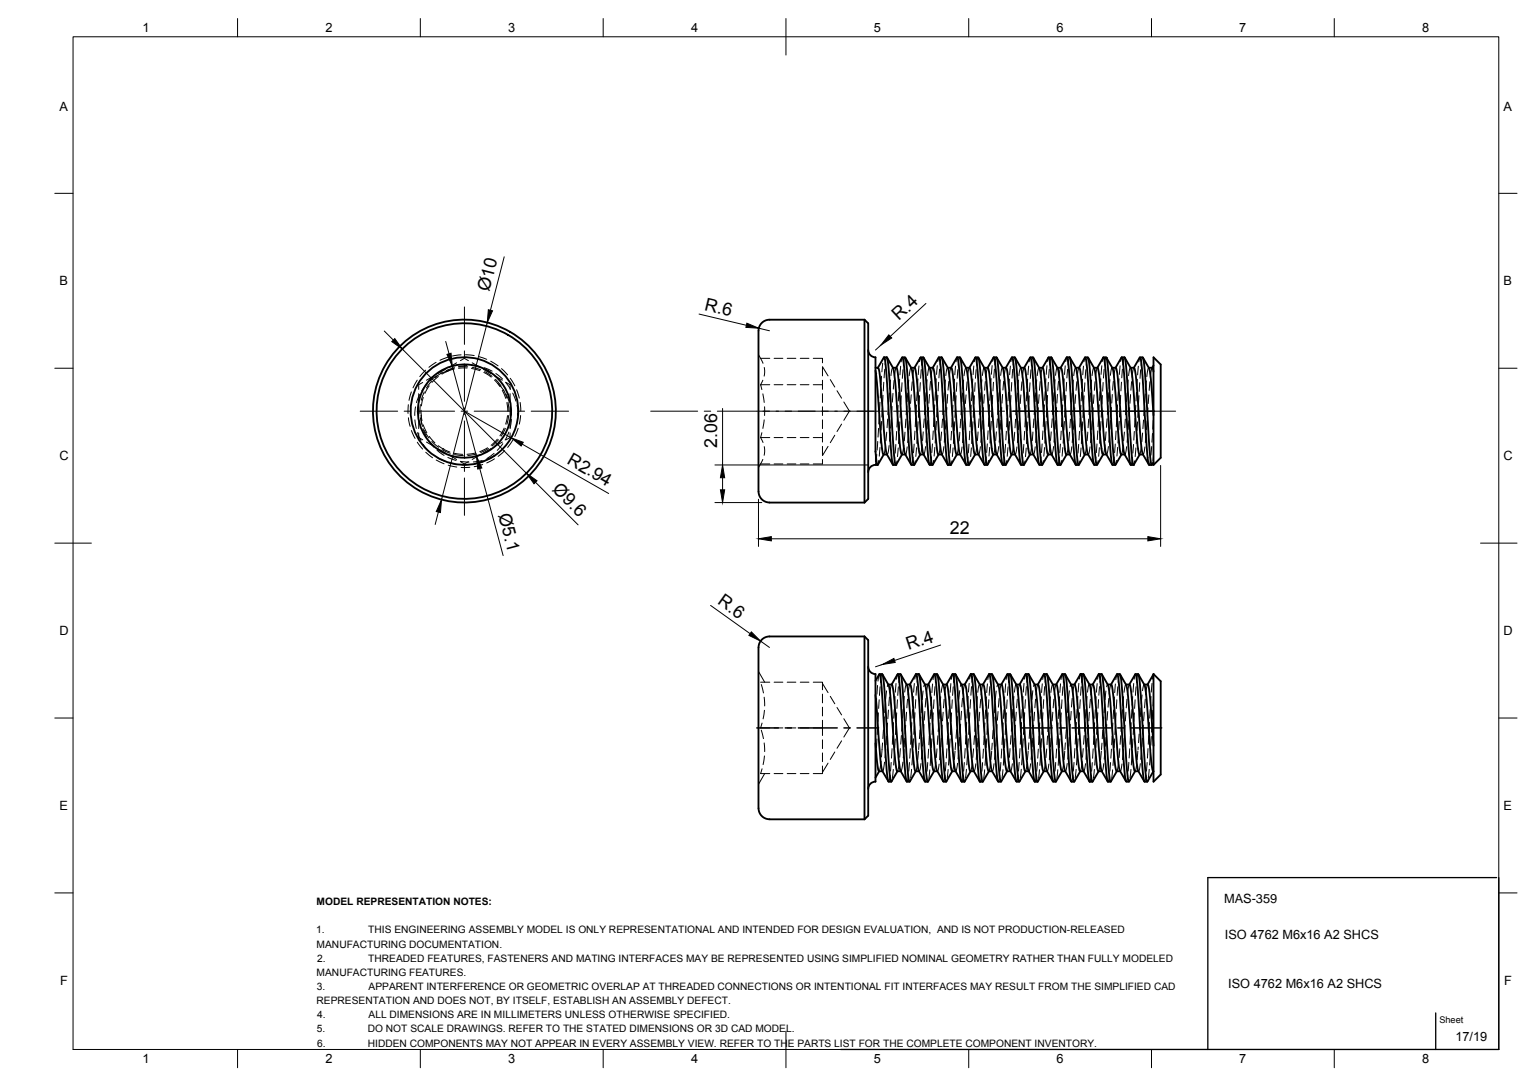
ISO-10303-21;
HEADER;
/* Generated by software containing ST-Developer
 * from STEP Tools, Inc. (www.steptools.com) 
 */

FILE_DESCRIPTION(
/* description */ (''),
/* implementation_level */ '2;1');

FILE_NAME(
/* name */ 'ISO 4762 M6x16 A2 SHCS.step',
/* time_stamp */ '2026-10-15T14:25:16-07:00',
/* author */ (''),
/* organization */ (''),
/* preprocessor_version */ 'ST-DEVELOPER v20.2',
/* originating_system */ 'Autodesk Translation Framework v15.15.0.0',
/* authorisation */ '');

FILE_SCHEMA (('AUTOMOTIVE_DESIGN { 1 0 10303 214 3 1 1 }'));
ENDSEC;

DATA;
#10=MECHANICAL_DESIGN_GEOMETRIC_PRESENTATION_REPRESENTATION('',(#339),#86429);
#159=TOROIDAL_SURFACE('',#17210,0.3342,0.04);
#160=TOROIDAL_SURFACE('',#17226,0.44,0.06);
#258=B_SPLINE_SURFACE_WITH_KNOTS('',3,3,((#85302,#85303,#85304,#85305,#85306,
#85307,#85308,#85309,#85310,#85311,#85312,#85313,#85314,#85315,#85316,#85317,
#85318,#85319,#85320,#85321,#85322,#85323,#85324,#85325,#85326,#85327,#85328,
#85329,#85330,#85331,#85332,#85333,#85334,#85335,#85336,#85337,#85338,#85339,
#85340,#85341,#85342,#85343,#85344,#85345,#85346,#85347,#85348,#85349,#85350,
#85351,#85352,#85353,#85354,#85355,#85356,#85357,#85358,#85359,#85360,#85361,
#85362,#85363,#85364,#85365,#85366,#85367,#85368,#85369,#85370,#85371,#85372,
#85373,#85374,#85375,#85376,#85377,#85378,#85379,#85380,#85381,#85382,#85383,
#85384,#85385,#85386,#85387,#85388,#85389,#85390,#85391,#85392,#85393,#85394,
#85395,#85396,#85397,#85398,#85399,#85400,#85401,#85402),(#85403,#85404,
#85405,#85406,#85407,#85408,#85409,#85410,#85411,#85412,#85413,#85414,#85415,
#85416,#85417,#85418,#85419,#85420,#85421,#85422,#85423,#85424,#85425,#85426,
#85427,#85428,#85429,#85430,#85431,#85432,#85433,#85434,#85435,#85436,#85437,
#85438,#85439,#85440,#85441,#85442,#85443,#85444,#85445,#85446,#85447,#85448,
#85449,#85450,#85451,#85452,#85453,#85454,#85455,#85456,#85457,#85458,#85459,
#85460,#85461,#85462,#85463,#85464,#85465,#85466,#85467,#85468,#85469,#85470,
#85471,#85472,#85473,#85474,#85475,#85476,#85477,#85478,#85479,#85480,#85481,
#85482,#85483,#85484,#85485,#85486,#85487,#85488,#85489,#85490,#85491,#85492,
#85493,#85494,#85495,#85496,#85497,#85498,#85499,#85500,#85501,#85502,#85503),
(#85504,#85505,#85506,#85507,#85508,#85509,#85510,#85511,#85512,#85513,
#85514,#85515,#85516,#85517,#85518,#85519,#85520,#85521,#85522,#85523,#85524,
#85525,#85526,#85527,#85528,#85529,#85530,#85531,#85532,#85533,#85534,#85535,
#85536,#85537,#85538,#85539,#85540,#85541,#85542,#85543,#85544,#85545,#85546,
#85547,#85548,#85549,#85550,#85551,#85552,#85553,#85554,#85555,#85556,#85557,
#85558,#85559,#85560,#85561,#85562,#85563,#85564,#85565,#85566,#85567,#85568,
#85569,#85570,#85571,#85572,#85573,#85574,#85575,#85576,#85577,#85578,#85579,
#85580,#85581,#85582,#85583,#85584,#85585,#85586,#85587,#85588,#85589,#85590,
#85591,#85592,#85593,#85594,#85595,#85596,#85597,#85598,#85599,#85600,#85601,
#85602,#85603,#85604),(#85605,#85606,#85607,#85608,#85609,#85610,#85611,
#85612,#85613,#85614,#85615,#85616,#85617,#85618,#85619,#85620,#85621,#85622,
#85623,#85624,#85625,#85626,#85627,#85628,#85629,#85630,#85631,#85632,#85633,
#85634,#85635,#85636,#85637,#85638,#85639,#85640,#85641,#85642,#85643,#85644,
#85645,#85646,#85647,#85648,#85649,#85650,#85651,#85652,#85653,#85654,#85655,
#85656,#85657,#85658,#85659,#85660,#85661,#85662,#85663,#85664,#85665,#85666,
#85667,#85668,#85669,#85670,#85671,#85672,#85673,#85674,#85675,#85676,#85677,
#85678,#85679,#85680,#85681,#85682,#85683,#85684,#85685,#85686,#85687,#85688,
#85689,#85690,#85691,#85692,#85693,#85694,#85695,#85696,#85697,#85698,#85699,
#85700,#85701,#85702,#85703,#85704,#85705)),.UNSPECIFIED.,.F.,.F.,.F.,(4,
4),(4,1,1,1,1,1,1,1,1,1,1,1,1,1,1,1,1,1,1,1,1,1,1,1,1,1,1,1,1,1,1,1,1,1,
1,1,1,1,1,1,1,1,1,1,1,1,1,1,1,1,1,1,1,1,1,1,1,1,1,1,1,1,1,1,1,1,1,1,1,1,
1,1,1,1,1,1,1,1,1,1,1,1,1,1,1,1,1,1,1,1,1,1,1,1,1,1,1,1,4),(-0.000485376732247951,
0.0662851291984278),(8.30747755240103,9.30363388226323,10.2997902121254,
11.2959465419876,12.2921028718499,13.2882592017121,14.2844155315743,15.2805718614365,
16.2767281912987,17.2728845211609,18.2690408510231,19.2651971808853,20.2613535107475,
21.2575098406097,22.2536661704719,23.2498225003341,24.2459788301963,25.2421351600585,
26.2382914899207,27.234447819783,28.2306041496452,29.2267604795074,30.2229168093696,
31.2190731392318,32.215229469094,33.2113857989562,34.2075421288184,35.2036984586806,
36.1998547885428,37.196011118405,38.1921674482672,39.1883237781294,40.1844801079916,
41.1806364378539,42.1767927677161,43.1729490975783,44.1691054274405,45.1652617573027,
46.1614180871649,47.1575744170271,48.1537307468893,49.1498870767515,50.1460434066137,
51.1421997364759,52.1383560663381,53.1345123962003,54.1306687260625,55.1268250559247,
56.122981385787,57.1191377156492,58.1152940455114,59.1114503753736,60.1076067052358,
61.103763035098,62.0999193649602,63.0960756948224,64.0922320246846,65.0883883545468,
66.084544684409,67.0807010142712,68.0768573441334,69.0730136739956,70.0691700038579,
71.0653263337201,72.0614826635823,73.0576389934445,74.0537953233067,75.0499516531689,
76.0461079830311,77.0422643128933,78.0384206427555,79.0345769726177,80.0307333024799,
81.0268896323421,82.0230459622043,83.0192022920665,84.0153586219288,85.011514951791,
86.0076712816532,87.0038276115154,87.9999839413776,88.9961402712398,89.992296601102,
90.9884529309642,91.9846092608264,92.9807655906886,93.9769219205508,94.973078250413,
95.9692345802752,96.9653909101374,97.9615472399996,98.9577035698618,99.9538598997241,
100.950016229586,101.946172559448,102.942328889311,103.938485219173,104.934641549035,
105.931283255629),.UNSPECIFIED.);
#259=B_SPLINE_SURFACE_WITH_KNOTS('',3,3,((#85831,#85832,#85833,#85834,#85835,
#85836,#85837,#85838,#85839,#85840,#85841,#85842,#85843,#85844,#85845,#85846,
#85847,#85848,#85849,#85850,#85851,#85852,#85853,#85854,#85855,#85856,#85857,
#85858,#85859,#85860,#85861,#85862,#85863,#85864,#85865,#85866,#85867,#85868,
#85869,#85870,#85871,#85872,#85873,#85874,#85875,#85876,#85877,#85878,#85879,
#85880,#85881,#85882,#85883,#85884,#85885,#85886,#85887,#85888,#85889,#85890,
#85891,#85892,#85893,#85894,#85895,#85896,#85897,#85898,#85899,#85900,#85901,
#85902,#85903,#85904,#85905,#85906,#85907,#85908,#85909,#85910,#85911,#85912,
#85913,#85914,#85915,#85916,#85917,#85918,#85919,#85920,#85921,#85922,#85923,
#85924,#85925,#85926,#85927,#85928,#85929,#85930,#85931),(#85932,#85933,
#85934,#85935,#85936,#85937,#85938,#85939,#85940,#85941,#85942,#85943,#85944,
#85945,#85946,#85947,#85948,#85949,#85950,#85951,#85952,#85953,#85954,#85955,
#85956,#85957,#85958,#85959,#85960,#85961,#85962,#85963,#85964,#85965,#85966,
#85967,#85968,#85969,#85970,#85971,#85972,#85973,#85974,#85975,#85976,#85977,
#85978,#85979,#85980,#85981,#85982,#85983,#85984,#85985,#85986,#85987,#85988,
#85989,#85990,#85991,#85992,#85993,#85994,#85995,#85996,#85997,#85998,#85999,
#86000,#86001,#86002,#86003,#86004,#86005,#86006,#86007,#86008,#86009,#86010,
#86011,#86012,#86013,#86014,#86015,#86016,#86017,#86018,#86019,#86020,#86021,
#86022,#86023,#86024,#86025,#86026,#86027,#86028,#86029,#86030,#86031,#86032),
(#86033,#86034,#86035,#86036,#86037,#86038,#86039,#86040,#86041,#86042,
#86043,#86044,#86045,#86046,#86047,#86048,#86049,#86050,#86051,#86052,#86053,
#86054,#86055,#86056,#86057,#86058,#86059,#86060,#86061,#86062,#86063,#86064,
#86065,#86066,#86067,#86068,#86069,#86070,#86071,#86072,#86073,#86074,#86075,
#86076,#86077,#86078,#86079,#86080,#86081,#86082,#86083,#86084,#86085,#86086,
#86087,#86088,#86089,#86090,#86091,#86092,#86093,#86094,#86095,#86096,#86097,
#86098,#86099,#86100,#86101,#86102,#86103,#86104,#86105,#86106,#86107,#86108,
#86109,#86110,#86111,#86112,#86113,#86114,#86115,#86116,#86117,#86118,#86119,
#86120,#86121,#86122,#86123,#86124,#86125,#86126,#86127,#86128,#86129,#86130,
#86131,#86132,#86133),(#86134,#86135,#86136,#86137,#86138,#86139,#86140,
#86141,#86142,#86143,#86144,#86145,#86146,#86147,#86148,#86149,#86150,#86151,
#86152,#86153,#86154,#86155,#86156,#86157,#86158,#86159,#86160,#86161,#86162,
#86163,#86164,#86165,#86166,#86167,#86168,#86169,#86170,#86171,#86172,#86173,
#86174,#86175,#86176,#86177,#86178,#86179,#86180,#86181,#86182,#86183,#86184,
#86185,#86186,#86187,#86188,#86189,#86190,#86191,#86192,#86193,#86194,#86195,
#86196,#86197,#86198,#86199,#86200,#86201,#86202,#86203,#86204,#86205,#86206,
#86207,#86208,#86209,#86210,#86211,#86212,#86213,#86214,#86215,#86216,#86217,
#86218,#86219,#86220,#86221,#86222,#86223,#86224,#86225,#86226,#86227,#86228,
#86229,#86230,#86231,#86232,#86233,#86234)),.UNSPECIFIED.,.F.,.F.,.F.,(4,
4),(4,1,1,1,1,1,1,1,1,1,1,1,1,1,1,1,1,1,1,1,1,1,1,1,1,1,1,1,1,1,1,1,1,1,
1,1,1,1,1,1,1,1,1,1,1,1,1,1,1,1,1,1,1,1,1,1,1,1,1,1,1,1,1,1,1,1,1,1,1,1,
1,1,1,1,1,1,1,1,1,1,1,1,1,1,1,1,1,1,1,1,1,1,1,1,1,1,1,1,4),(-0.000418551673040404,
0.0663322186430087),(11.6145474273763,12.6111891776804,13.6073455075426,
14.6035018374048,15.5996581672671,16.5958144971293,17.5919708269915,18.5881271568537,
19.5842834867159,20.5804398165781,21.5765961464403,22.5727524763025,23.5689088061647,
24.5650651360269,25.5612214658891,26.5573777957513,27.5535341256135,28.5496904554757,
29.545846785338,30.5420031152002,31.5381594450624,32.5343157749246,33.5304721047868,
34.526628434649,35.5227847645112,36.5189410943734,37.5150974242356,38.5112537540978,
39.50741008396,40.5035664138222,41.4997227436844,42.4958790735466,43.4920354034089,
44.4881917332711,45.4843480631333,46.4805043929955,47.4766607228577,48.4728170527199,
49.4689733825821,50.4651297124443,51.4612860423065,52.4574423721687,53.4535987020309,
54.4497550318931,55.4459113617553,56.4420676916176,57.4382240214798,58.434380351342,
59.4305366812042,60.4266930110664,61.4228493409286,62.4190056707908,63.415162000653,
64.4113183305152,65.4074746603774,66.4036309902396,67.3997873201018,68.395943649964,
69.3920999798262,70.3882563096884,71.3844126395506,72.3805689694129,73.3767252992751,
74.3728816291373,75.3690379589995,76.3651942888617,77.3613506187239,78.3575069485861,
79.3536632784483,80.3498196083105,81.3459759381727,82.3421322680349,83.3382885978971,
84.3344449277593,85.3306012576216,86.3267575874838,87.322913917346,88.3190702472082,
89.3152265770704,90.3113829069326,91.3075392367948,92.303695566657,93.2998518965192,
94.2960082263814,95.2921645562436,96.2883208861058,97.284477215968,98.2806335458303,
99.2767898756925,100.272946205555,101.269102535417,102.265258865279,103.261415195141,
104.257571525003,105.253727854866,106.249884184728,107.24604051459,108.242196844452,
109.238353174315),.UNSPECIFIED.);
#280=(
BOUNDED_CURVE()
B_SPLINE_CURVE(2,(#86249,#86250,#86251),.UNSPECIFIED.,.F.,.F.)
B_SPLINE_CURVE_WITH_KNOTS((3,3),(-0.639366558443436,-0.433164349146202),
 .UNSPECIFIED.)
CURVE()
GEOMETRIC_REPRESENTATION_ITEM()
RATIONAL_B_SPLINE_CURVE((1.35866716012837,1.4637604307034,1.4637604307034))
REPRESENTATION_ITEM('')
);
#281=(
BOUNDED_CURVE()
B_SPLINE_CURVE(2,(#86253,#86254,#86255),.UNSPECIFIED.,.F.,.F.)
B_SPLINE_CURVE_WITH_KNOTS((3,3),(0.0319010196424347,0.336489692457453),
 .UNSPECIFIED.)
CURVE()
GEOMETRIC_REPRESENTATION_ITEM()
RATIONAL_B_SPLINE_CURVE((1.03712812921102,1.19757240916823,1.03712812921102))
REPRESENTATION_ITEM('')
);
#282=(
BOUNDED_CURVE()
B_SPLINE_CURVE(2,(#86257,#86258,#86259),.UNSPECIFIED.,.F.,.F.)
B_SPLINE_CURVE_WITH_KNOTS((3,3),(0.0319010196424348,0.336489692457454),
 .UNSPECIFIED.)
CURVE()
GEOMETRIC_REPRESENTATION_ITEM()
RATIONAL_B_SPLINE_CURVE((1.03712812921102,1.19757240916823,1.03712812921102))
REPRESENTATION_ITEM('')
);
#283=(
BOUNDED_CURVE()
B_SPLINE_CURVE(2,(#86261,#86262,#86263),.UNSPECIFIED.,.F.,.F.)
B_SPLINE_CURVE_WITH_KNOTS((3,3),(0.031901019642435,0.336489692457454),
 .UNSPECIFIED.)
CURVE()
GEOMETRIC_REPRESENTATION_ITEM()
RATIONAL_B_SPLINE_CURVE((1.03712812921102,1.19757240916823,1.03712812921102))
REPRESENTATION_ITEM('')
);
#284=(
BOUNDED_CURVE()
B_SPLINE_CURVE(2,(#86265,#86266,#86267),.UNSPECIFIED.,.F.,.F.)
B_SPLINE_CURVE_WITH_KNOTS((3,3),(0.0319010196424349,0.336489692457453),
 .UNSPECIFIED.)
CURVE()
GEOMETRIC_REPRESENTATION_ITEM()
RATIONAL_B_SPLINE_CURVE((1.03712812921102,1.19757240916823,1.03712812921102))
REPRESENTATION_ITEM('')
);
#285=(
BOUNDED_CURVE()
B_SPLINE_CURVE(2,(#86269,#86270,#86271),.UNSPECIFIED.,.F.,.F.)
B_SPLINE_CURVE_WITH_KNOTS((3,3),(0.0319010196424348,0.336489692457453),
 .UNSPECIFIED.)
CURVE()
GEOMETRIC_REPRESENTATION_ITEM()
RATIONAL_B_SPLINE_CURVE((1.03712812921102,1.19757240916823,1.03712812921102))
REPRESENTATION_ITEM('')
);
#286=(
BOUNDED_CURVE()
B_SPLINE_CURVE(2,(#86272,#86273,#86274),.UNSPECIFIED.,.F.,.F.)
B_SPLINE_CURVE_WITH_KNOTS((3,3),(-0.433164349146202,-0.226962139848967),
 .UNSPECIFIED.)
CURVE()
GEOMETRIC_REPRESENTATION_ITEM()
RATIONAL_B_SPLINE_CURVE((1.4637604307034,1.4637604307034,1.35866716012837))
REPRESENTATION_ITEM('')
);
#303=SHAPE_REPRESENTATION_RELATIONSHIP('SRR','None',#86518,#321);
#321=ADVANCED_BREP_SHAPE_REPRESENTATION('',(#357),#86427);
#339=STYLED_ITEM('',(#86617),#357);
#357=MANIFOLD_SOLID_BREP('Body1',#15629);
#1057=B_SPLINE_CURVE_WITH_KNOTS('',3,(#77452,#77453,#77454,#77455,#77456,
#77457,#77458,#77459,#77460,#77461,#77462,#77463,#77464,#77465,#77466,#77467,
#77468,#77469,#77470,#77471,#77472,#77473,#77474,#77475,#77476,#77477,#77478,
#77479,#77480,#77481,#77482,#77483,#77484,#77485,#77486,#77487,#77488,#77489,
#77490,#77491,#77492,#77493,#77494,#77495,#77496,#77497,#77498,#77499,#77500,
#77501,#77502,#77503,#77504,#77505,#77506,#77507,#77508,#77509,#77510,#77511,
#77512,#77513,#77514,#77515,#77516,#77517,#77518,#77519,#77520,#77521,#77522,
#77523,#77524,#77525,#77526,#77527),.UNSPECIFIED.,.F.,.F.,(4,3,3,3,3,3,
3,3,3,3,3,3,3,3,3,3,3,3,3,3,3,3,3,3,3,4),(10.3765279447494,10.5534408108777,
10.7390672436552,10.9156311402548,11.092209959865,11.2691639748381,11.2959465419876,
11.4749627408317,11.6536283105826,11.8322755610944,12.0108999290652,12.1899418681108,
12.2921028718499,12.4705669207875,12.6486653263687,12.8267315154106,13.0047661728317,
13.1832164114546,13.2882592017121,13.4670164932441,13.6454135437631,13.8237819839401,
14.0021213662665,14.1808742422402,14.2844155315743,14.3150784600182),
 .UNSPECIFIED.);
#1058=B_SPLINE_CURVE_WITH_KNOTS('',3,(#77530,#77531,#77532,#77533,#77534,
#77535,#77536,#77537,#77538,#77539,#77540,#77541,#77542,#77543,#77544,#77545,
#77546,#77547,#77548,#77549,#77550,#77551,#77552,#77553,#77554,#77555,#77556,
#77557,#77558,#77559,#77560,#77561,#77562,#77563,#77564,#77565,#77566,#77567,
#77568,#77569,#77570,#77571,#77572,#77573,#77574,#77575,#77576,#77577,#77578),
 .UNSPECIFIED.,.F.,.F.,(4,3,3,3,3,3,3,3,3,3,3,3,3,3,3,3,4),(11.6150328478182,
11.7979860071945,11.9808051200463,12.1638372320247,12.3469748436598,12.5306212400219,
12.6111891776804,12.7880694650036,12.9645487109607,13.1409651633225,13.3173295184066,
13.4941088918777,13.6073455075426,13.7863288313326,13.9649582660013,14.1435821147139,
14.3143563514564),.UNSPECIFIED.);
#1059=B_SPLINE_CURVE_WITH_KNOTS('',3,(#77584,#77585,#77586,#77587,#77588,
#77589,#77590,#77591,#77592,#77593,#77594,#77595,#77596,#77597,#77598,#77599,
#77600,#77601,#77602,#77603,#77604,#77605,#77606,#77607,#77608,#77609,#77610,
#77611,#77612,#77613,#77614,#77615,#77616,#77617,#77618,#77619,#77620,#77621,
#77622,#77623,#77624,#77625,#77626,#77627,#77628,#77629,#77630,#77631,#77632,
#77633,#77634,#77635,#77636,#77637,#77638,#77639,#77640,#77641,#77642,#77643,
#77644,#77645,#77646,#77647,#77648,#77649,#77650,#77651,#77652,#77653,#77654,
#77655,#77656,#77657,#77658,#77659,#77660,#77661,#77662,#77663,#77664,#77665,
#77666,#77667,#77668,#77669,#77670,#77671,#77672,#77673,#77674,#77675,#77676,
#77677,#77678,#77679,#77680,#77681,#77682,#77683,#77684,#77685,#77686,#77687,
#77688,#77689,#77690,#77691,#77692,#77693,#77694,#77695,#77696,#77697,#77698,
#77699,#77700,#77701,#77702,#77703,#77704,#77705,#77706,#77707,#77708,#77709,
#77710,#77711,#77712,#77713,#77714,#77715,#77716,#77717,#77718,#77719,#77720,
#77721,#77722,#77723,#77724,#77725,#77726,#77727,#77728,#77729,#77730,#77731,
#77732,#77733,#77734,#77735,#77736,#77737,#77738,#77739,#77740,#77741),
 .UNSPECIFIED.,.F.,.F.,(4,2,2,2,2,2,2,2,2,2,2,2,2,2,2,2,2,2,2,2,2,2,2,2,
2,2,2,2,2,2,2,2,2,2,2,2,2,2,2,2,2,2,2,2,2,2,2,2,2,2,2,2,2,2,2,2,2,2,2,2,
2,2,2,2,2,2,2,2,2,2,2,2,2,2,2,2,2,2,4),(-1.1637686371979,-1.15330190866645,
-1.1266227046362,-1.09256064921497,-1.08738467839962,-1.08447804691533,
-1.08221855966446,-1.078997200995,-1.0720929569109,-1.04172615958735,-0.985477222491362,
-0.973796375831997,-0.968166209598214,-0.963720443538658,-0.958703261039998,
-0.950091205374077,-0.939562238885692,-0.916459677578588,-0.889953461342887,
-0.855674071252519,-0.850495008033263,-0.847587736517607,-0.845328814306583,
-0.84210950273686,-0.835213509442295,-0.804921450089816,-0.748914527944634,
-0.737014184892147,-0.731344381402372,-0.726895540281821,-0.721904410910814,
-0.713411634220441,-0.664373131981111,-0.621067249054008,-0.614391305574181,
-0.611213164706316,-0.608717662740495,-0.605671704503774,-0.599674578529323,
-0.591733080982927,-0.571582639447149,-0.524620788345343,-0.503713938265148,
-0.496545413852407,-0.491834230609183,-0.48728251741021,-0.480927115237638,
-0.464837122792203,-0.440267116686382,-0.389050830868198,-0.379089415497616,
-0.375263526244851,-0.372703238844456,-0.36999731328955,-0.365610004255846,
-0.349585865669542,-0.315288663196602,-0.272878790086403,-0.263461724321359,
-0.257718225983789,-0.253258721643605,-0.248303879589581,-0.239991273220952,
-0.19806005041918,-0.155468977463997,-0.142952258400057,-0.138787202372248,
-0.136393940808784,-0.133822998673744,-0.13006462663369,-0.119778194296598,
-0.103142576294788,-0.050478661657663,-0.0298185732069449,-0.0226922099751356,
-0.0179928562598389,-0.0137879733802478,-0.00934196527458575,-0.000699766182984735),
 .UNSPECIFIED.);
#1060=B_SPLINE_CURVE_WITH_KNOTS('',3,(#77742,#77743,#77744,#77745,#77746,
#77747,#77748,#77749,#77750,#77751,#77752,#77753,#77754,#77755,#77756,#77757,
#77758,#77759,#77760,#77761,#77762,#77763,#77764,#77765,#77766,#77767,#77768,
#77769),.UNSPECIFIED.,.F.,.F.,(4,3,3,3,3,3,3,3,3,4),(14.3150784600182,14.4937457776235,
14.6720840543341,14.8504232808183,15.0287613104912,15.2075061341743,15.2805718614365,
15.4753006968871,15.6687760212031,15.7079632676679),.UNSPECIFIED.);
#1061=B_SPLINE_CURVE_WITH_KNOTS('',3,(#77771,#77772,#77773,#77774,#77775,
#77776,#77777,#77778,#77779,#77780,#77781,#77782,#77783,#77784,#77785,#77786,
#77787,#77788,#77789,#77790,#77791,#77792,#77793,#77794,#77795,#77796,#77797,
#77798),.UNSPECIFIED.,.F.,.F.,(4,3,3,3,3,3,3,3,3,4),(14.3143563514564,14.4933094485465,
14.6035018374048,14.782517919735,14.9611833677346,15.1398304904322,15.3184547270006,
15.4974965315266,15.5996581672671,15.7079632679489),.UNSPECIFIED.);
#1062=B_SPLINE_CURVE_WITH_KNOTS('',3,(#77799,#77800,#77801,#77802,#77803,
#77804,#77805,#77806,#77807),.UNSPECIFIED.,.F.,.F.,(4,1,1,1,1,1,4),(15.7079719561269,
16.5958144971293,17.5919708269915,18.5881271568537,19.5842834867159,20.5804398165781,
20.5982114559267),.UNSPECIFIED.);
#1063=B_SPLINE_CURVE_WITH_KNOTS('',3,(#77812,#77813,#77814,#77815,#77816,
#77817,#77818,#77819,#77820,#77821,#77822,#77823,#77824,#77825,#77826,#77827,
#77828,#77829,#77830,#77831,#77832,#77833,#77834,#77835,#77836,#77837,#77838,
#77839,#77840,#77841,#77842,#77843,#77844,#77845,#77846,#77847,#77848,#77849,
#77850,#77851,#77852,#77853,#77854,#77855,#77856,#77857,#77858,#77859,#77860,
#77861,#77862,#77863,#77864,#77865,#77866,#77867,#77868,#77869,#77870,#77871,
#77872,#77873,#77874,#77875,#77876,#77877,#77878,#77879,#77880,#77881,#77882,
#77883,#77884,#77885,#77886,#77887,#77888,#77889,#77890,#77891,#77892,#77893,
#77894,#77895,#77896,#77897,#77898,#77899,#77900,#77901,#77902,#77903,#77904,
#77905,#77906,#77907,#77908,#77909,#77910,#77911,#77912,#77913,#77914,#77915,
#77916,#77917,#77918,#77919,#77920,#77921,#77922,#77923,#77924,#77925,#77926,
#77927,#77928,#77929,#77930,#77931,#77932,#77933,#77934,#77935,#77936,#77937,
#77938,#77939,#77940,#77941,#77942,#77943,#77944,#77945,#77946,#77947,#77948,
#77949,#77950,#77951,#77952,#77953,#77954,#77955,#77956,#77957,#77958,#77959,
#77960,#77961,#77962,#77963,#77964,#77965,#77966,#77967,#77968,#77969,#77970,
#77971,#77972,#77973,#77974,#77975,#77976,#77977,#77978,#77979,#77980,#77981,
#77982,#77983,#77984,#77985,#77986,#77987,#77988,#77989,#77990,#77991,#77992,
#77993,#77994,#77995,#77996,#77997,#77998,#77999,#78000,#78001,#78002,#78003,
#78004,#78005,#78006,#78007,#78008,#78009,#78010,#78011),.UNSPECIFIED.,
 .F.,.F.,(4,2,2,2,2,2,2,2,2,2,2,2,2,2,2,2,2,2,2,2,2,2,2,2,2,2,2,2,2,2,2,
2,2,2,2,2,2,2,2,2,2,2,2,2,2,2,2,2,2,2,2,2,2,2,2,2,2,2,2,2,2,2,2,2,2,2,2,
2,2,2,2,2,2,2,2,2,2,2,2,2,2,2,2,2,2,2,2,2,2,2,2,2,2,2,2,2,2,2,2,4),(-2.65808856585573,
-2.63896562788725,-2.63024927627796,-2.62521051743156,-2.62076872278231,
-2.61517461241825,-2.6062689530765,-2.5513950124766,-2.51544918010836,-2.50936210629664,
-2.50629807350984,-2.50380303304675,-2.50064471262094,-2.49407411644601,
-2.44976929489784,-2.40203764363037,-2.39331977274927,-2.38828057986316,
-2.38383866330352,-2.37824474799765,-2.36934011948885,-2.31445077379584,
-2.27851439127394,-2.27242733281257,-2.26936323959744,-2.2668681185348,
-2.26370965614897,-2.25713861298752,-2.2017312222126,-2.17077686377812,
-2.15859407969893,-2.15287242873246,-2.14841731415237,-2.14345454859754,
-2.13509748541681,-2.0951234442445,-2.05593101002078,-2.0387950323599,-2.03431776630312,
-2.03159340734376,-2.02904621173316,-2.02588911944168,-2.01787577779181,
-1.96444395966839,-1.93959584089493,-1.92857108602373,-1.91964494170661,
-1.91456171004154,-1.91012494278449,-1.90459542172365,-1.89381350566269,
-1.83664403989336,-1.80598134791393,-1.79904746452727,-1.79582076722484,
-1.79356077273059,-1.79065792279702,-1.78549903676126,-1.75436601730428,
-1.74873945594128,-1.72440702662619,-1.70150725376204,-1.68616841063085,
-1.67992413442162,-1.67539174120084,-1.67121220600676,-1.66437677015089,
-1.64621779537558,-1.59677293989029,-1.57591590069346,-1.56395836850383,
-1.55998444930628,-1.55736887806426,-1.55469837777831,-1.55046830899439,
-1.53739869282542,-1.4952686832497,-1.45374841823445,-1.44537309055035,
-1.44040618715214,-1.43595146846488,-1.43023605973783,-1.41808965995798,
-1.38854667801837,-1.37144368022104,-1.3320774905639,-1.32522592009405,
-1.32201448470216,-1.31951701519194,-1.31649796412889,-1.31063541532598,
-1.27331494399624,-1.21970325024029,-1.2106828051401,-1.20505488719733,
-1.20060947887647,-1.19559121578042,-1.18697354308848,-1.1764356290778,
-1.1637686371979),.UNSPECIFIED.);
#1064=B_SPLINE_CURVE_WITH_KNOTS('',3,(#78013,#78014,#78015,#78016,#78017),
 .UNSPECIFIED.,.F.,.F.,(4,1,4),(20.5982114559267,21.5765961464403,21.9911426690459),
 .UNSPECIFIED.);
#1065=B_SPLINE_CURVE_WITH_KNOTS('',3,(#78018,#78019,#78020,#78021,#78022,
#78023,#78024,#78025,#78026,#78027,#78028,#78029,#78030,#78031,#78032,#78033,
#78034,#78035,#78036,#78037,#78038,#78039,#78040,#78041,#78042,#78043,#78044,
#78045,#78046,#78047,#78048,#78049,#78050,#78051,#78052,#78053,#78054,#78055,
#78056,#78057,#78058,#78059,#78060,#78061,#78062,#78063,#78064,#78065,#78066,
#78067,#78068,#78069,#78070,#78071,#78072,#78073,#78074,#78075,#78076,#78077,
#78078,#78079,#78080,#78081,#78082,#78083,#78084,#78085,#78086,#78087,#78088,
#78089,#78090,#78091,#78092,#78093,#78094,#78095,#78096,#78097,#78098,#78099,
#78100,#78101,#78102,#78103,#78104,#78105,#78106,#78107,#78108,#78109,#78110,
#78111,#78112,#78113,#78114,#78115,#78116,#78117,#78118,#78119,#78120,#78121,
#78122,#78123,#78124,#78125,#78126,#78127,#78128,#78129,#78130,#78131,#78132,
#78133,#78134,#78135,#78136,#78137,#78138,#78139,#78140,#78141,#78142,#78143,
#78144,#78145,#78146,#78147,#78148,#78149,#78150,#78151,#78152,#78153,#78154,
#78155,#78156,#78157,#78158,#78159,#78160,#78161,#78162,#78163,#78164,#78165,
#78166,#78167,#78168,#78169,#78170,#78171,#78172,#78173,#78174,#78175,#78176,
#78177,#78178,#78179),.UNSPECIFIED.,.F.,.F.,(4,2,2,2,2,2,2,2,2,2,2,2,2,
2,2,2,2,2,2,2,2,2,2,2,2,2,2,2,2,2,2,2,2,2,2,2,2,2,2,2,2,2,2,2,2,2,2,2,2,
2,2,2,2,2,2,2,2,2,2,2,2,2,2,2,2,2,2,2,2,2,2,2,2,2,2,2,2,2,2,2,4),(-2.98904427612266,
-2.98271778473439,-2.97723402516263,-2.972808221092,-2.96859102543041,-2.9638636072836,
-2.95660538824093,-2.9347749884518,-2.8780081973523,-2.86484611471672,-2.85611824490066,
-2.85258738524914,-2.85005559451206,-2.84723593943615,-2.84231751051577,
-2.82084252248546,-2.77782499244362,-2.75666538903467,-2.74214902509585,
-2.73603421462947,-2.73152544592232,-2.72731801991099,-2.72032021305432,
-2.70093465123872,-2.65264122893888,-2.63211123115884,-2.62407775210138,
-2.61802862591414,-2.61497288896346,-2.61247871788276,-2.60931409623699,
-2.60270569116392,-2.55889221680947,-2.51069964266647,-2.50201121946722,
-2.49697984405979,-2.49253943310642,-2.48694023389954,-2.47541478443228,
-2.4189661619931,-2.38852972679637,-2.38162043088732,-2.3783993783485,-2.37614113267091,
-2.37323753987195,-2.36807078495652,-2.33461177733176,-2.30788095203421,
-2.28444726017468,-2.27382408444184,-2.26515242446383,-2.260124416451,-2.25568323515178,
-2.25007803662293,-2.23852146689319,-2.18210551792869,-2.15167878190711,
-2.14477021088004,-2.1415491492634,-2.13929074525505,-2.13638671022134,
-2.13121871603868,-2.0976648901883,-2.07107968066547,-2.04761151404457,
-2.03697807939041,-2.02829972680073,-2.02326999295449,-2.01882855559658,
-2.01322473389622,-2.00428263892065,-1.94016200242408,-1.92088338084325,
-1.91316033955907,-1.90729069036377,-1.90427084749759,-1.90177442137465,
-1.89856660520185,-1.89173066883819,-1.85200521610118,-1.82619474000714),
 .UNSPECIFIED.);
#1066=B_SPLINE_CURVE_WITH_KNOTS('',3,(#78185,#78186,#78187,#78188,#78189,
#78190,#78191,#78192,#78193,#78194,#78195,#78196,#78197,#78198,#78199,#78200,
#78201,#78202,#78203,#78204,#78205,#78206,#78207,#78208,#78209,#78210,#78211,
#78212,#78213,#78214,#78215,#78216,#78217,#78218,#78219,#78220,#78221,#78222,
#78223,#78224,#78225,#78226,#78227,#78228,#78229,#78230,#78231,#78232,#78233,
#78234,#78235,#78236,#78237,#78238,#78239,#78240,#78241,#78242,#78243,#78244,
#78245,#78246,#78247,#78248,#78249,#78250,#78251,#78252,#78253,#78254,#78255,
#78256,#78257,#78258,#78259,#78260,#78261,#78262,#78263,#78264,#78265,#78266,
#78267,#78268,#78269,#78270,#78271,#78272,#78273,#78274,#78275,#78276,#78277,
#78278,#78279,#78280,#78281,#78282,#78283,#78284,#78285,#78286,#78287,#78288,
#78289,#78290,#78291,#78292,#78293,#78294,#78295,#78296,#78297,#78298,#78299,
#78300,#78301,#78302,#78303,#78304,#78305,#78306,#78307,#78308,#78309,#78310,
#78311,#78312,#78313,#78314,#78315,#78316,#78317,#78318,#78319,#78320,#78321,
#78322,#78323,#78324,#78325,#78326,#78327,#78328,#78329,#78330,#78331,#78332,
#78333,#78334),.UNSPECIFIED.,.F.,.F.,(4,2,2,2,2,2,2,2,2,2,2,2,2,2,2,2,2,
2,2,2,2,2,2,2,2,2,2,2,2,2,2,2,2,2,2,2,2,2,2,2,2,2,2,2,2,2,2,2,2,2,2,2,2,
2,2,2,2,2,2,2,2,2,2,2,2,2,2,2,2,2,2,2,2,2,4),(-1.16370274550239,-1.1568070636298,
-1.13677589009422,-1.09022559976082,-1.06886026428964,-1.06164448485992,
-1.05692378948761,-1.0523786955524,-1.04605868477085,-1.03020861191811,
-1.00617866458583,-0.960418696062841,-0.945412959897615,-0.940975534683176,
-0.938259967017763,-0.935677531247388,-0.931866614661771,-0.921205588553841,
-0.903674646488405,-0.850676930739111,-0.831467699059262,-0.824489994217004,
-0.820285042041834,-0.81577164368852,-0.809637560886505,-0.795009473094288,
-0.773617630303817,-0.730663875046565,-0.709419145398833,-0.704509960324899,
-0.701691479497393,-0.69915723216955,-0.695618378437064,-0.686847962239203,
-0.673600358750618,-0.640301644144528,-0.597358254095201,-0.589007533560267,
-0.584046121250254,-0.579590717172288,-0.573866598030166,-0.561670356831813,
-0.530349090617642,-0.475447713250732,-0.468765208229255,-0.465585489510032,
-0.463089540991608,-0.460043956096899,-0.454049880629331,-0.419293719725962,
-0.362790523781181,-0.354060467579551,-0.348517507309125,-0.344079690939804,
-0.339005837902028,-0.330124410646265,-0.319169620966451,-0.29457213689166,
-0.24317543339214,-0.233373696231229,-0.229572198251925,-0.227088455460331,
-0.224467495629112,-0.220543910049425,-0.215691303369064,-0.185311480080651,
-0.129024907015343,-0.117373078218063,-0.111748538710975,-0.107303611633095,
-0.102283579199003,-0.093656951979499,-0.045572454012865,-0.0264879389893685,
-0.000696886015620926),.UNSPECIFIED.);
#1067=B_SPLINE_CURVE_WITH_KNOTS('',3,(#78335,#78336,#78337,#78338,#78339,
#78340,#78341,#78342,#78343,#78344,#78345,#78346,#78347,#78348,#78349,#78350,
#78351,#78352,#78353,#78354,#78355,#78356,#78357,#78358,#78359,#78360,#78361,
#78362,#78363,#78364,#78365,#78366,#78367,#78368,#78369,#78370,#78371,#78372,
#78373,#78374,#78375,#78376,#78377,#78378,#78379,#78380,#78381,#78382,#78383,
#78384),.UNSPECIFIED.,.F.,.F.,(4,2,2,2,2,2,2,2,2,2,2,2,2,2,2,2,2,2,2,2,
2,2,2,2,4),(-2.98929417603817,-2.98366351093371,-2.98108078519344,-2.97872868114393,
-2.97602838999981,-2.97166071400982,-2.95731736208476,-2.90550643056215,
-2.88469583141012,-2.87034731868861,-2.86425776659884,-2.85975166729322,
-2.85553532914993,-2.84849538068428,-2.82877056877828,-2.78076354833954,
-2.76031364017731,-2.7522987727458,-2.74625987964001,-2.74320552365715,
-2.74071023304375,-2.73754130231533,-2.73091460922501,-2.68712217695227,
-2.65808856585573),.UNSPECIFIED.);
#1068=B_SPLINE_CURVE_WITH_KNOTS('',3,(#78385,#78386,#78387,#78388,#78389,
#78390,#78391,#78392,#78393,#78394,#78395,#78396,#78397,#78398,#78399,#78400,
#78401,#78402,#78403,#78404,#78405,#78406,#78407,#78408,#78409,#78410,#78411,
#78412,#78413,#78414,#78415,#78416,#78417,#78418,#78419,#78420,#78421,#78422,
#78423,#78424,#78425,#78426,#78427,#78428,#78429,#78430,#78431,#78432,#78433,
#78434,#78435,#78436,#78437,#78438,#78439,#78440,#78441,#78442,#78443,#78444,
#78445,#78446,#78447,#78448,#78449,#78450,#78451,#78452,#78453,#78454,#78455,
#78456,#78457,#78458,#78459,#78460,#78461,#78462,#78463,#78464,#78465,#78466,
#78467,#78468,#78469,#78470,#78471,#78472,#78473,#78474,#78475,#78476,#78477,
#78478,#78479,#78480,#78481,#78482,#78483,#78484,#78485,#78486,#78487,#78488,
#78489,#78490,#78491,#78492,#78493,#78494,#78495,#78496,#78497,#78498,#78499,
#78500,#78501,#78502,#78503,#78504,#78505,#78506,#78507,#78508,#78509,#78510,
#78511,#78512,#78513,#78514,#78515,#78516,#78517,#78518,#78519,#78520,#78521,
#78522,#78523,#78524,#78525,#78526,#78527,#78528,#78529,#78530,#78531,#78532,
#78533,#78534,#78535,#78536,#78537,#78538,#78539,#78540,#78541,#78542,#78543,
#78544,#78545,#78546,#78547,#78548,#78549,#78550,#78551,#78552,#78553,#78554,
#78555,#78556,#78557,#78558,#78559,#78560,#78561,#78562,#78563,#78564,#78565,
#78566,#78567,#78568,#78569,#78570,#78571,#78572,#78573,#78574,#78575,#78576,
#78577,#78578,#78579,#78580,#78581,#78582,#78583,#78584,#78585,#78586,#78587,
#78588,#78589,#78590),.UNSPECIFIED.,.F.,.F.,(4,2,2,2,2,2,2,2,2,2,2,2,2,
2,2,2,2,2,2,2,2,2,2,2,2,2,2,2,2,2,2,2,2,2,2,2,2,2,2,2,2,2,2,2,2,2,2,2,2,
2,2,2,2,2,2,2,2,2,2,2,2,2,2,2,2,2,2,2,2,2,2,2,2,2,2,2,2,2,2,2,2,2,2,2,2,
2,2,2,2,2,2,2,2,2,2,2,2,2,2,2,2,2,4),(-1.82619474000714,-1.81669741450079,
-1.79650086386287,-1.789613921023,-1.78496136321705,-1.78042251728144,-1.77491811234969,
-1.76127711035731,-1.74625882417755,-1.68188711327217,-1.67211761041369,
-1.66842967734056,-1.66587063032776,-1.66311420019153,-1.65848885920151,
-1.64151002192613,-1.60225772689917,-1.56897584375519,-1.55672051941941,
-1.55098639324071,-1.54653051962872,-1.54157609445583,-1.53325563140524,
-1.49466335660825,-1.45743394032513,-1.437550799349,-1.43271462594213,-1.42991222682865,
-1.42737282286278,-1.42379962009082,-1.41480533885329,-1.40108138580043,
-1.34043394780875,-1.32244194173736,-1.31563144561288,-1.31145732217809,
-1.30692316509088,-1.30066249446532,-1.28520789385302,-1.26205154942839,
-1.2352577680559,-1.20133550613098,-1.19616217617814,-1.19325661030326,
-1.19099786028261,-1.18777748573651,-1.18087490185015,-1.15051586874477,
-1.09430007401147,-1.08258277692584,-1.07694694805024,-1.07250191359706,
-1.06749108174361,-1.0589041346484,-1.04841376525451,-1.02544119200211,
-1.00018973591792,-0.96714389852926,-0.960900215830101,-0.957762813917686,
-0.955221096582854,-0.952489029087609,-0.947974317147941,-0.930342404916655,
-0.888683926910013,-0.851675930912225,-0.843385475754152,-0.838437776911538,
-0.833981018607295,-0.828236015619667,-0.815918204719248,-0.780911992980148,
-0.738774158470005,-0.725680028827143,-0.721447940407098,-0.718777634633902,
-0.716163722646667,-0.712194629329707,-0.700269438407626,-0.679498921374576,
-0.630347434893704,-0.611914528525312,-0.605042390726706,-0.600857341912173,
-0.596331960689134,-0.590121185929433,-0.574993877641159,-0.552545240818545,
-0.525568261588957,-0.490706261849459,-0.485516419066132,-0.482607273277968,
-0.480349276223882,-0.477134579256861,-0.470261993623915,-0.440196236852249,
-0.384897242937592,-0.372356597316411,-0.366634047993919,-0.362168080016405,
-0.357259060357152,-0.349149922815078,-0.331944024529),.UNSPECIFIED.);
#1069=B_SPLINE_CURVE_WITH_KNOTS('',3,(#78595,#78596,#78597,#78598,#78599,
#78600,#78601,#78602,#78603,#78604,#78605,#78606,#78607,#78608,#78609,#78610,
#78611,#78612,#78613,#78614,#78615,#78616,#78617,#78618,#78619,#78620,#78621,
#78622,#78623,#78624,#78625,#78626,#78627,#78628,#78629,#78630,#78631,#78632,
#78633,#78634,#78635,#78636,#78637,#78638,#78639,#78640,#78641,#78642,#78643,
#78644,#78645,#78646,#78647,#78648,#78649,#78650,#78651,#78652,#78653,#78654,
#78655,#78656,#78657,#78658,#78659,#78660,#78661,#78662,#78663,#78664,#78665,
#78666,#78667,#78668,#78669,#78670,#78671,#78672,#78673,#78674,#78675,#78676,
#78677,#78678,#78679,#78680,#78681,#78682,#78683,#78684,#78685,#78686,#78687,
#78688,#78689,#78690,#78691,#78692,#78693,#78694,#78695,#78696,#78697,#78698,
#78699,#78700,#78701,#78702,#78703,#78704,#78705,#78706,#78707,#78708,#78709,
#78710,#78711,#78712,#78713,#78714,#78715,#78716,#78717,#78718,#78719,#78720,
#78721,#78722,#78723,#78724,#78725,#78726,#78727,#78728,#78729,#78730,#78731,
#78732,#78733,#78734,#78735,#78736,#78737,#78738,#78739,#78740,#78741,#78742,
#78743,#78744,#78745,#78746,#78747,#78748,#78749,#78750,#78751,#78752,#78753,
#78754,#78755,#78756,#78757,#78758,#78759,#78760,#78761,#78762,#78763,#78764,
#78765,#78766,#78767,#78768,#78769,#78770,#78771,#78772,#78773,#78774,#78775,
#78776,#78777,#78778,#78779,#78780,#78781,#78782,#78783,#78784,#78785,#78786,
#78787,#78788,#78789,#78790,#78791,#78792),.UNSPECIFIED.,.F.,.F.,(4,2,2,
2,2,2,2,2,2,2,2,2,2,2,2,2,2,2,2,2,2,2,2,2,2,2,2,2,2,2,2,2,2,2,2,2,2,2,2,
2,2,2,2,2,2,2,2,2,2,2,2,2,2,2,2,2,2,2,2,2,2,2,2,2,2,2,2,2,2,2,2,2,2,2,2,
2,2,2,2,2,2,2,2,2,2,2,2,2,2,2,2,2,2,2,2,2,2,2,4),(-2.65779610798801,-2.64562846272747,
-2.60539466897641,-2.59993510794725,-2.59699977757073,-2.59449419130625,
-2.59122688046561,-2.58387137384898,-2.52947682521431,-2.5045178668195,
-2.49346363101895,-2.48451958776003,-2.47943357363947,-2.47499861327236,
-2.46947687916789,-2.45836581710353,-2.40144586488319,-2.37086433866569,
-2.36393979188862,-2.3607154206473,-2.3584562875984,-2.35555347922215,-2.35039226412067,
-2.31812074255177,-2.31274400261798,-2.2892518720084,-2.26640335760273,
-2.25594928612956,-2.24738482600682,-2.24237868461594,-2.23793270748448,
-2.23228870337808,-2.22321002925658,-2.17029679400594,-2.13275401676145,
-2.12665282896889,-2.12358626746513,-2.12109169838593,-2.11793716643286,
-2.1113848807021,-2.06676972492304,-2.01930673296878,-2.01060593952897,
-2.00557084313888,-2.00112913862138,-1.99553093590684,-1.98661005050956,
-1.93190836177424,-1.89505724763879,-1.88944323507208,-1.88647547099182,
-1.88397380115751,-1.88075105932935,-1.87364845895274,-1.82617224122379,
-1.78178492927898,-1.77341929044655,-1.76845513984121,-1.76400104671987,
-1.75828386923519,-1.74895229982513,-1.70113421315615,-1.65903167114846,
-1.65288311093852,-1.64980701890483,-1.64731252070541,-1.6441679185956,
-1.63766814368582,-1.59197443816894,-1.57816910688654,-1.5555758876386,
-1.54037970337555,-1.53415780035787,-1.52962986346544,-1.5248794105215,
-1.51752078509346,-1.49484243099641,-1.45484019718156,-1.42066591456986,
-1.41548888453754,-1.41258223510258,-1.41032322344123,-1.40710314550051,
-1.4002036909885,-1.36987820446382,-1.31375981100097,-1.30196519050354,
-1.29631459278727,-1.29186747410937,-1.28686429341757,-1.27831569524545,
-1.22924081769557,-1.18611808435823,-1.17941967489536,-1.17623716529217,
-1.17374136543791,-1.17069882392811,-1.16471888888895,-1.16370274550239),
 .UNSPECIFIED.);
#1070=B_SPLINE_CURVE_WITH_KNOTS('',3,(#78794,#78795,#78796,#78797,#78798,
#78799,#78800,#78801,#78802,#78803,#78804,#78805,#78806,#78807,#78808,#78809,
#78810,#78811,#78812,#78813,#78814,#78815,#78816,#78817,#78818,#78819,#78820,
#78821,#78822,#78823,#78824,#78825,#78826,#78827,#78828,#78829,#78830,#78831,
#78832,#78833,#78834,#78835,#78836,#78837,#78838,#78839,#78840,#78841,#78842,
#78843),.UNSPECIFIED.,.F.,.F.,(4,2,2,2,2,2,2,2,2,2,2,2,2,2,2,2,2,2,2,2,
2,2,2,2,4),(-0.331944024529,-0.312841878134531,-0.295797672941764,-0.256356303392932,
-0.249523574006143,-0.246316348325045,-0.24381997457475,-0.240799682720564,
-0.234927739803417,-0.195081674214772,-0.144398316709289,-0.135177121109271,
-0.129492211160779,-0.125042428831186,-0.12006158181438,-0.111614647314127,
-0.10134315480156,-0.0791140033701062,-0.0287009707118166,-0.0151068306855188,
-0.0108193652246315,-0.00813703130472152,-0.00579380909874595,-0.00316163883082362,
-0.000696074731363536),.UNSPECIFIED.);
#1071=B_SPLINE_CURVE_WITH_KNOTS('',3,(#78844,#78845,#78846,#78847,#78848,
#78849,#78850,#78851,#78852,#78853,#78854,#78855,#78856,#78857,#78858,#78859,
#78860,#78861,#78862,#78863,#78864,#78865,#78866,#78867,#78868,#78869,#78870,
#78871,#78872,#78873,#78874,#78875,#78876,#78877,#78878,#78879,#78880,#78881,
#78882,#78883,#78884,#78885,#78886,#78887,#78888,#78889,#78890,#78891,#78892,
#78893,#78894,#78895,#78896,#78897,#78898,#78899,#78900,#78901,#78902,#78903,
#78904,#78905,#78906,#78907,#78908,#78909,#78910,#78911,#78912,#78913,#78914,
#78915,#78916,#78917,#78918,#78919,#78920,#78921,#78922,#78923,#78924,#78925,
#78926,#78927,#78928,#78929,#78930,#78931,#78932,#78933,#78934,#78935,#78936,
#78937,#78938,#78939,#78940,#78941,#78942,#78943,#78944,#78945,#78946,#78947,
#78948,#78949,#78950,#78951,#78952,#78953,#78954,#78955,#78956,#78957,#78958,
#78959,#78960,#78961,#78962,#78963,#78964,#78965,#78966,#78967,#78968,#78969,
#78970,#78971,#78972,#78973,#78974,#78975,#78976,#78977,#78978,#78979,#78980,
#78981,#78982,#78983,#78984,#78985,#78986,#78987,#78988,#78989,#78990,#78991,
#78992,#78993,#78994,#78995,#78996,#78997,#78998,#78999,#79000,#79001,#79002,
#79003,#79004,#79005,#79006,#79007,#79008,#79009,#79010,#79011,#79012,#79013,
#79014,#79015,#79016,#79017,#79018,#79019,#79020,#79021,#79022,#79023,#79024,
#79025,#79026,#79027,#79028,#79029,#79030,#79031,#79032,#79033,#79034,#79035,
#79036,#79037,#79038,#79039),.UNSPECIFIED.,.F.,.F.,(4,2,2,2,2,2,2,2,2,2,
2,2,2,2,2,2,2,2,2,2,2,2,2,2,2,2,2,2,2,2,2,2,2,2,2,2,2,2,2,2,2,2,2,2,2,2,
2,2,2,2,2,2,2,2,2,2,2,2,2,2,2,2,2,2,2,2,2,2,2,2,2,2,2,2,2,2,2,2,2,2,2,2,
2,2,2,2,2,2,2,2,2,2,2,2,2,2,2,4),(-2.98986290590906,-2.9811645609045,-2.93860454829328,
-2.89411772806824,-2.88536790530145,-2.8803230618328,-2.87588370936346,
-2.87030313328637,-2.86144069728388,-2.79693950862918,-2.77781347126643,
-2.77012912135672,-2.76594868825332,-2.76245881001136,-2.76241330075756,
-2.76236793090525,-2.7623226514419,-2.76227741250219,-2.76223216313041,
-2.76218685102507,-2.7621414222526,-2.76209582093373,-2.7620499889014,-2.76200386531906,
-2.76195738624712,-2.7619104841631,-2.76186308740373,-2.76181511954432,
-2.76176649867618,-2.76171713657784,-2.76166693774644,-2.76161579827013,
-2.76156360450819,-2.76151023152379,-2.76145554121485,-2.76139938008659,
-2.76134157654138,-2.76130713089662,-2.7588952078203,-2.75575019173004,
-2.74924639835194,-2.70397057987953,-2.65698912986836,-2.64833458917462,
-2.64330966533014,-2.63886715545892,-2.63325481985386,-2.62166306138798,
-2.56527676212363,-2.53485753660154,-2.52794910234861,-2.52472774225655,
-2.52246900472342,-2.51956438114988,-2.51439489299499,-2.48075844393766,
-2.45428442783653,-2.43079032625652,-2.42014887725035,-2.41146516604408,
-2.40643384957864,-2.40199191514795,-2.3963886777886,-2.38484700688701,
-2.32839887375958,-2.29795931995531,-2.29104856636941,-2.28782664159736,
-2.2855677078503,-2.28266311284791,-2.2774942984965,-2.24396712553781,-2.21694798800437,
-2.18885651097065,-2.17675251197165,-2.17104566766734,-2.1665928882549,
-2.16162330150009,-2.1532316396023,-2.10914264085504,-2.07326352521092,
-2.05686094880649,-2.05244370148903,-2.04973277551116,-2.0471784146474,
-2.04337912651513,-2.03358852798327,-1.98220305753126,-1.95761568076255,
-1.94151656959651,-1.93516060948433,-1.93060946631103,-1.92589974097122,
-1.91873524137024,-1.89786176046146,-1.85083914353397,-1.83066715315173,
-1.82676239401596),.UNSPECIFIED.);
#1072=B_SPLINE_CURVE_WITH_KNOTS('',3,(#79045,#79046,#79047,#79048,#79049,
#79050,#79051,#79052,#79053,#79054,#79055,#79056,#79057,#79058,#79059,#79060,
#79061,#79062,#79063,#79064,#79065,#79066,#79067,#79068,#79069,#79070,#79071,
#79072,#79073,#79074,#79075,#79076,#79077,#79078,#79079,#79080,#79081,#79082,
#79083,#79084,#79085,#79086,#79087,#79088,#79089,#79090,#79091,#79092,#79093,
#79094,#79095,#79096,#79097,#79098,#79099,#79100,#79101,#79102,#79103,#79104,
#79105,#79106,#79107,#79108,#79109,#79110,#79111,#79112,#79113,#79114,#79115,
#79116,#79117,#79118,#79119,#79120,#79121,#79122,#79123,#79124,#79125,#79126,
#79127,#79128,#79129,#79130,#79131,#79132,#79133,#79134,#79135,#79136,#79137,
#79138,#79139,#79140,#79141,#79142,#79143,#79144,#79145,#79146,#79147,#79148,
#79149,#79150,#79151,#79152,#79153,#79154,#79155,#79156,#79157,#79158,#79159,
#79160,#79161,#79162,#79163,#79164,#79165,#79166,#79167,#79168,#79169,#79170,
#79171,#79172,#79173,#79174,#79175,#79176,#79177,#79178,#79179,#79180,#79181,
#79182,#79183,#79184,#79185,#79186,#79187,#79188,#79189,#79190,#79191,#79192,
#79193,#79194,#79195,#79196,#79197,#79198,#79199,#79200),.UNSPECIFIED.,
 .F.,.F.,(4,2,2,2,2,2,2,2,2,2,2,2,2,2,2,2,2,2,2,2,2,2,2,2,2,2,2,2,2,2,2,
2,2,2,2,2,2,2,2,2,2,2,2,2,2,2,2,2,2,2,2,2,2,2,2,2,2,2,2,2,2,2,2,2,2,2,2,
2,2,2,2,2,2,2,2,2,2,4),(-1.16379924314915,-1.15636896341719,-1.15072066708933,
-1.14627242167782,-1.14126489131265,-1.13270105731949,-1.122248306252,-1.09940987025486,
-1.07662727515485,-1.04094595192493,-1.0339798750836,-1.03074690518291,
-1.02824774255948,-1.02524482100174,-1.01946304593492,-1.01189225967026,
-0.993214480620849,-0.930428876149755,-0.919137758977803,-0.91358027292429,
-0.909140699661688,-0.904075522018791,-0.89523755988362,-0.848586864867644,
-0.803271713780177,-0.796745700141823,-0.79359547923121,-0.791100113886125,
-0.788027371158756,-0.781898592007223,-0.741786031843394,-0.691828023119278,
-0.68256938397034,-0.676872150100689,-0.672419035246775,-0.667440953377183,
-0.659014738978724,-0.610846558273101,-0.566350925816522,-0.559786690543437,
-0.556629115506364,-0.554133508653195,-0.551067343783175,-0.544971869070915,
-0.508097090812731,-0.45439106830036,-0.445377150286841,-0.43975067632214,
-0.43530481552055,-0.430284357372875,-0.421658607396983,-0.411108472381106,
-0.387934685436907,-0.361082605444902,-0.327237667455879,-0.32206376080669,
-0.319157366076106,-0.31689761785202,-0.31367527182871,-0.306766223562171,
-0.276355430680164,-0.220041575978518,-0.208419630605263,-0.202800111613543,
-0.198355065547207,-0.193585482945275,-0.185515120101929,-0.175629661124755,
-0.15468558629736,-0.126343850363146,-0.0930276647544607,-0.0861036582085444,
-0.0828786447279151,-0.0803802108174482,-0.0773715980702051,-0.0715610444402044,
-0.0639408967511788,-0.000697042157991375),.UNSPECIFIED.);
#1073=B_SPLINE_CURVE_WITH_KNOTS('',3,(#79201,#79202,#79203,#79204,#79205,
#79206,#79207,#79208,#79209,#79210,#79211,#79212,#79213,#79214,#79215,#79216,
#79217,#79218,#79219,#79220,#79221,#79222,#79223,#79224,#79225,#79226,#79227,
#79228,#79229,#79230,#79231,#79232,#79233,#79234,#79235,#79236,#79237,#79238,
#79239,#79240,#79241,#79242,#79243,#79244,#79245,#79246,#79247,#79248),
 .UNSPECIFIED.,.F.,.F.,(4,2,2,2,2,2,2,2,2,2,2,2,2,2,2,2,2,2,2,2,2,2,2,4),
(-2.98915910611891,-2.97245947833514,-2.96192457934277,-2.95701634474704,
-2.95285674097329,-2.94840886300484,-2.94274081448435,-2.93357753277321,
-2.90038509321121,-2.85100678772585,-2.84310478890941,-2.83713139739069,
-2.83409067085517,-2.83159548951468,-2.82841268419511,-2.82170994269704,
-2.77869299185966,-2.72942034717541,-2.72097004287315,-2.71598853099697,
-2.71153890583765,-2.70585519559141,-2.69663786776816,-2.65779610798801),
 .UNSPECIFIED.);
#1074=B_SPLINE_CURVE_WITH_KNOTS('',3,(#79249,#79250,#79251,#79252,#79253,
#79254,#79255,#79256,#79257,#79258,#79259,#79260,#79261,#79262,#79263,#79264,
#79265,#79266,#79267,#79268,#79269,#79270,#79271,#79272,#79273,#79274,#79275,
#79276,#79277,#79278,#79279,#79280,#79281,#79282,#79283,#79284,#79285,#79286,
#79287,#79288,#79289,#79290,#79291,#79292,#79293,#79294,#79295,#79296,#79297,
#79298,#79299,#79300,#79301,#79302,#79303,#79304,#79305,#79306,#79307,#79308,
#79309,#79310,#79311,#79312,#79313,#79314,#79315,#79316,#79317,#79318,#79319,
#79320,#79321,#79322,#79323,#79324,#79325,#79326,#79327,#79328,#79329,#79330,
#79331,#79332,#79333,#79334,#79335,#79336,#79337,#79338,#79339,#79340,#79341,
#79342,#79343,#79344,#79345,#79346,#79347,#79348,#79349,#79350,#79351,#79352,
#79353,#79354,#79355,#79356,#79357,#79358,#79359,#79360,#79361,#79362,#79363,
#79364,#79365,#79366,#79367,#79368,#79369,#79370,#79371,#79372,#79373,#79374,
#79375,#79376,#79377,#79378,#79379,#79380,#79381,#79382,#79383,#79384,#79385,
#79386,#79387,#79388,#79389,#79390,#79391,#79392,#79393,#79394,#79395,#79396,
#79397,#79398,#79399,#79400,#79401,#79402,#79403,#79404,#79405,#79406,#79407,
#79408,#79409,#79410,#79411,#79412,#79413,#79414,#79415,#79416,#79417,#79418,
#79419,#79420,#79421,#79422,#79423,#79424,#79425,#79426,#79427,#79428,#79429,
#79430,#79431,#79432,#79433,#79434,#79435,#79436,#79437,#79438,#79439,#79440,
#79441,#79442,#79443,#79444,#79445,#79446),.UNSPECIFIED.,.F.,.F.,(4,2,2,
2,2,2,2,2,2,2,2,2,2,2,2,2,2,2,2,2,2,2,2,2,2,2,2,2,2,2,2,2,2,2,2,2,2,2,2,
2,2,2,2,2,2,2,2,2,2,2,2,2,2,2,2,2,2,2,2,2,2,2,2,2,2,2,2,2,2,2,2,2,2,2,2,
2,2,2,2,2,2,2,2,2,2,2,2,2,2,2,2,2,2,2,2,2,2,2,4),(-1.82676239401596,-1.82272046736094,
-1.81672091864089,-1.81367460450555,-1.81117924027603,-1.80800188504408,
-1.8013298649085,-1.7580267840685,-1.70924301533283,-1.70062747953582,-1.69561033741196,
-1.69116586736496,-1.68553910548193,-1.67652046621759,-1.61274221472753,
-1.59331247162085,-1.58189494164362,-1.57798706850257,-1.57538545123259,
-1.57269840983678,-1.56839104192817,-1.55463061891724,-1.4955156127764,
-1.47041984850611,-1.46275451371483,-1.45793950490291,-1.45344188485792,
-1.44740446573964,-1.43337791652622,-1.413220985141,-1.38407955151575,-1.38005003406147,
-1.34749079807617,-1.34232668583597,-1.33942307286952,-1.33716382487661,
-1.33394011285789,-1.32702015150965,-1.29649124919368,-1.23973617586962,
-1.22848682257969,-1.22293841141856,-1.21850097949893,-1.21343274810444,
-1.20457502187683,-1.15733511690643,-1.11269733616998,-1.10614179980468,
-1.10298658428462,-1.10049195548535,-1.09742599605467,-1.09132813154709,
-1.05408312357184,-1.00082882547132,-0.99177827370505,-0.986142248348315,
-0.981696912608493,-0.976685587035129,-0.968097401569503,-0.957605304200283,
-0.934627738823065,-0.909330944315578,-0.876330208293993,-0.869413873939793,
-0.866190919756722,-0.863693398680025,-0.860685152702294,-0.854873429719196,
-0.847250648331001,-0.82836692863714,-0.763302226245086,-0.754566639982387,
-0.749022920635514,-0.744586250510679,-0.739515645666495,-0.730645165239772,
-0.683031336154004,-0.638842550674269,-0.632260667672222,-0.629100609290637,
-0.626606077557796,-0.623545066603632,-0.617471143539917,-0.582497314957043,
-0.526431192927454,-0.517653839910276,-0.512097855466582,-0.50766019084905,
-0.502597991192227,-0.493767450989743,-0.447247709854124,-0.401792231986257,
-0.395275352028411,-0.39212771591288,-0.389633504948396,-0.386561177872874,
-0.380430377273958,-0.339941241296865,-0.332197600308329),.UNSPECIFIED.);
#1075=B_SPLINE_CURVE_WITH_KNOTS('',3,(#79451,#79452,#79453,#79454,#79455,
#79456,#79457,#79458,#79459,#79460,#79461,#79462,#79463,#79464,#79465,#79466,
#79467,#79468,#79469,#79470,#79471,#79472,#79473,#79474,#79475,#79476,#79477,
#79478,#79479,#79480,#79481,#79482,#79483,#79484,#79485,#79486,#79487,#79488,
#79489,#79490,#79491,#79492,#79493,#79494,#79495,#79496,#79497,#79498,#79499,
#79500,#79501,#79502,#79503,#79504,#79505,#79506,#79507,#79508,#79509,#79510,
#79511,#79512,#79513,#79514,#79515,#79516,#79517,#79518,#79519,#79520,#79521,
#79522,#79523,#79524,#79525,#79526,#79527,#79528,#79529,#79530,#79531,#79532,
#79533,#79534,#79535,#79536,#79537,#79538,#79539,#79540,#79541,#79542,#79543,
#79544,#79545,#79546,#79547,#79548,#79549,#79550,#79551,#79552,#79553,#79554,
#79555,#79556,#79557,#79558,#79559,#79560,#79561,#79562,#79563,#79564,#79565,
#79566,#79567,#79568,#79569,#79570,#79571,#79572,#79573,#79574,#79575,#79576,
#79577,#79578,#79579,#79580,#79581,#79582,#79583,#79584,#79585,#79586,#79587,
#79588,#79589,#79590,#79591,#79592,#79593,#79594,#79595,#79596,#79597,#79598,
#79599,#79600,#79601,#79602,#79603,#79604,#79605,#79606,#79607,#79608,#79609,
#79610,#79611,#79612,#79613,#79614,#79615,#79616,#79617,#79618,#79619,#79620,
#79621,#79622,#79623,#79624,#79625,#79626,#79627,#79628,#79629,#79630,#79631,
#79632,#79633,#79634,#79635,#79636,#79637,#79638,#79639,#79640),
 .UNSPECIFIED.,.F.,.F.,(4,2,2,2,2,2,2,2,2,2,2,2,2,2,2,2,2,2,2,2,2,2,2,2,
2,2,2,2,2,2,2,2,2,2,2,2,2,2,2,2,2,2,2,2,2,2,2,2,2,2,2,2,2,2,2,2,2,2,2,2,
2,2,2,2,2,2,2,2,2,2,2,2,2,2,2,2,2,2,2,2,2,2,2,2,2,2,2,2,2,2,2,2,2,2,4),
(-2.65859608544945,-2.62817910170511,-2.58437028368493,-2.57601440365146,
-2.571051323549,-2.56659528312859,-2.5608715489283,-2.55152047038777,-2.49369700679251,
-2.46283216116232,-2.45587742894055,-2.45264657005837,-2.45038579877802,
-2.44748496724804,-2.44233627240993,-2.41233954330086,-2.40526107340166,
-2.38119073015443,-2.3583020538318,-2.347834471791,-2.33926050119821,-2.33425083955854,
-2.32980295714294,-2.32415819594495,-2.31508180698964,-2.25156923357792,
-2.23202522553656,-2.22056246588569,-2.2166479852476,-2.21404426909698,
-2.21135738552999,-2.20705406924471,-2.19334050291578,-2.15169049035824,
-2.11696751793303,-2.10465790537969,-2.09891227863287,-2.09445312207183,
-2.08950077478548,-2.08119764972497,-2.04378958095283,-1.99125956410559,
-1.98265868956199,-1.97914565951749,-1.97661460206172,-1.97378222075131,
-1.96881201920436,-1.94630493608452,-1.88114589965967,-1.86800701449476,
-1.86211633147386,-1.85763872917848,-1.85275879231972,-1.84479471115785,
-1.81479636460211,-1.76670608254294,-1.74793815324269,-1.74333865183246,
-1.740587009559,-1.73805288610591,-1.73495088315162,-1.72885517867193,-1.68626225621433,
-1.6425125587349,-1.63048752591444,-1.62479329641393,-1.62033998404953,
-1.61535904853054,-1.60692146675987,-1.564779200056,-1.53311180376467,-1.51841426851518,
-1.50897317785005,-1.5053318262702,-1.50278007777218,-1.50000379410264,
-1.49529141098926,-1.47479374619411,-1.41286016526844,-1.3959282015441,
-1.389271789414,-1.38512366001183,-1.38056335713426,-1.37416400039939,-1.35777411797176,
-1.33252148097241,-1.27740740931621,-1.27076402206258,-1.26759127004963,
-1.26509504021232,-1.26204205650427,-1.25601317382717,-1.21827261936714,
-1.16545743281103,-1.16379924314915),.UNSPECIFIED.);
#1076=B_SPLINE_CURVE_WITH_KNOTS('',3,(#79642,#79643,#79644,#79645,#79646,
#79647,#79648,#79649,#79650,#79651,#79652,#79653,#79654,#79655,#79656,#79657,
#79658,#79659,#79660,#79661,#79662,#79663,#79664,#79665,#79666,#79667,#79668,
#79669,#79670,#79671,#79672,#79673,#79674,#79675,#79676,#79677,#79678,#79679,
#79680,#79681,#79682,#79683,#79684,#79685,#79686,#79687),.UNSPECIFIED.,
 .F.,.F.,(4,2,2,2,2,2,2,2,2,2,2,2,2,2,2,2,2,2,2,2,2,2,4),(-0.332197600308329,
-0.290459994424418,-0.281158016782542,-0.275449637666639,-0.270996994379766,
-0.266028932018693,-0.257643229512439,-0.21223658910391,-0.164557803963349,
-0.158226854367379,-0.155115112347663,-0.152621276036858,-0.149514409956841,
-0.143208445307593,-0.134725934841315,-0.0826658288797491,-0.0497946970644482,
-0.0415948920940171,-0.0366663182927132,-0.0323511497472415,-0.0280322450478533,
-0.0224655565253524,-0.000695812465232673),.UNSPECIFIED.);
#1077=B_SPLINE_CURVE_WITH_KNOTS('',3,(#79688,#79689,#79690,#79691,#79692,
#79693,#79694,#79695,#79696,#79697,#79698,#79699,#79700,#79701,#79702,#79703,
#79704,#79705,#79706,#79707,#79708,#79709,#79710,#79711,#79712,#79713,#79714,
#79715,#79716,#79717,#79718,#79719,#79720,#79721,#79722,#79723,#79724,#79725,
#79726,#79727,#79728,#79729,#79730,#79731,#79732,#79733,#79734,#79735,#79736,
#79737,#79738,#79739,#79740,#79741,#79742,#79743,#79744,#79745,#79746,#79747,
#79748,#79749,#79750,#79751,#79752,#79753,#79754,#79755,#79756,#79757,#79758,
#79759,#79760,#79761,#79762,#79763,#79764,#79765,#79766,#79767,#79768,#79769,
#79770,#79771,#79772,#79773,#79774,#79775),.UNSPECIFIED.,.F.,.F.,(4,3,3,
3,3,3,3,3,3,3,3,3,3,3,3,3,3,3,3,3,3,3,3,3,3,3,3,3,3,4),(47.1238898042296,
47.3286926477564,47.4766607228577,47.6553657376643,47.8337102124053,48.0120264379798,
48.1903137393774,48.3690157785142,48.4728170527199,48.6515220675267,48.8298665422679,
49.0081827678426,49.1864700692404,49.3651721083774,49.4689733825821,49.647678397389,
49.8260228721303,50.004339097705,50.1826263991029,50.36132843824,50.4651297124443,
50.6438347272511,50.8221792019923,51.0004954275669,51.1787827289647,51.3574847681017,
51.4612860423065,51.6399881173827,51.8269247910562,52.0138614647296),
 .UNSPECIFIED.);
#1078=B_SPLINE_CURVE_WITH_KNOTS('',3,(#79781,#79782,#79783,#79784,#79785,
#79786,#79787,#79788,#79789,#79790,#79791,#79792,#79793,#79794,#79795,#79796,
#79797,#79798,#79799,#79800,#79801,#79802,#79803,#79804,#79805,#79806,#79807,
#79808,#79809,#79810,#79811,#79812,#79813,#79814,#79815,#79816,#79817,#79818,
#79819,#79820,#79821,#79822,#79823,#79824,#79825,#79826,#79827,#79828,#79829,
#79830,#79831,#79832,#79833,#79834,#79835,#79836,#79837,#79838,#79839,#79840,
#79841,#79842,#79843,#79844,#79845,#79846,#79847,#79848,#79849,#79850,#79851,
#79852,#79853,#79854,#79855,#79856,#79857,#79858,#79859,#79860,#79861,#79862,
#79863,#79864,#79865,#79866,#79867,#79868,#79869,#79870,#79871,#79872,#79873,
#79874,#79875,#79876,#79877,#79878,#79879,#79880,#79881,#79882,#79883,#79884,
#79885,#79886,#79887,#79888,#79889,#79890,#79891,#79892,#79893,#79894,#79895,
#79896,#79897,#79898,#79899,#79900,#79901,#79902,#79903,#79904,#79905,#79906,
#79907,#79908,#79909,#79910,#79911,#79912,#79913,#79914,#79915,#79916,#79917,
#79918,#79919,#79920,#79921,#79922,#79923,#79924,#79925,#79926,#79927,#79928,
#79929,#79930,#79931,#79932,#79933,#79934,#79935,#79936),.UNSPECIFIED.,
 .F.,.F.,(4,2,2,2,2,2,2,2,2,2,2,2,2,2,2,2,2,2,2,2,2,2,2,2,2,2,2,2,2,2,2,
2,2,2,2,2,2,2,2,2,2,2,2,2,2,2,2,2,2,2,2,2,2,2,2,2,2,2,2,2,2,2,2,2,2,2,2,
2,2,2,2,2,2,2,2,2,2,4),(-1.16393257116699,-1.13155274745225,-1.12508806491967,
-1.12194991398079,-1.11945515879177,-1.11637208757233,-1.11018972849946,
-1.10192554845814,-1.08044126644041,-1.02872142490933,-1.01297389570421,
-1.0065022436161,-1.00197480216914,-0.99730401055951,-0.990332310858646,
-0.96940172797567,-0.931778065923655,-0.89532455660756,-0.888423995035991,
-0.885203506784727,-0.882705566670822,-0.879693897099228,-0.873867475291317,
-0.86621997042688,-0.847241099589446,-0.782427276276276,-0.773638560814754,
-0.768078550296022,-0.763639584726894,-0.758577934423205,-0.749753602736751,
-0.703428419713985,-0.657754162968758,-0.651249509549554,-0.648103773210307,
-0.645609003600592,-0.642533342645965,-0.636387935069918,-0.594544566656325,
-0.546486952813495,-0.537163651934748,-0.531448438119805,-0.526994087816146,
-0.522027811896464,-0.513654114227301,-0.468960984030539,-0.420395221834905,
-0.41416299930872,-0.411070136488645,-0.408575570263599,-0.405447822538307,
-0.399036818154827,-0.363229375887451,-0.308855308108324,-0.299906966489975,
-0.294300145689517,-0.289856880380281,-0.284825625308487,-0.276146012998223,
-0.26551053925916,-0.242038703259375,-0.196888389307316,-0.180593129937533,
-0.176038425688853,-0.173297083493113,-0.170729374605992,-0.166996425831666,
-0.15738313407824,-0.130095110759329,-0.0901850250516212,-0.0672920231607177,
-0.059911131319319,-0.0551555669674362,-0.0506293516416139,-0.0461590020233244,
-0.0401480748676892,-0.0268826235989323,-0.00069612616442647),
 .UNSPECIFIED.);
#1079=B_SPLINE_CURVE_WITH_KNOTS('',3,(#79937,#79938,#79939,#79940,#79941,
#79942,#79943,#79944,#79945,#79946,#79947,#79948,#79949,#79950,#79951,#79952,
#79953,#79954,#79955,#79956,#79957,#79958,#79959,#79960,#79961,#79962,#79963,
#79964,#79965,#79966,#79967,#79968,#79969,#79970,#79971,#79972,#79973,#79974,
#79975,#79976,#79977,#79978,#79979,#79980,#79981,#79982,#79983,#79984,#79985,
#79986,#79987,#79988,#79989,#79990,#79991,#79992,#79993,#79994,#79995,#79996,
#79997,#79998,#79999,#80000,#80001,#80002,#80003,#80004,#80005,#80006,#80007,
#80008,#80009,#80010,#80011,#80012),.UNSPECIFIED.,.F.,.F.,(4,2,2,2,2,2,
2,2,2,2,2,2,2,2,2,2,2,2,2,2,2,2,2,2,2,2,2,2,2,2,2,2,2,2,2,2,2,4),(-2.98974118664277,
-2.9416975746077,-2.93336580449747,-2.92978943526336,-2.92656213697401,
-2.92430195639035,-2.921399211717,-2.91624122597365,-2.88532156037506,-2.84760447046011,
-2.82915334249667,-2.81608733299606,-2.81111829359434,-2.8109105208265,
-2.81069964473556,-2.81063190304778,-2.81055390944443,-2.81046354560391,
-2.81035807252723,-2.81023387906299,-2.81008609442015,-2.80990796855895,
-2.80968983646161,-2.80941729046844,-2.80906772872268,-2.80853924051187,
-2.80410704328531,-2.79865537218159,-2.79023542997861,-2.7311467053471,
-2.70772846347949,-2.69486040900539,-2.69078207162925,-2.68814425328089,
-2.68581230526217,-2.68259562236814,-2.6743501568114,-2.65859608544945),
 .UNSPECIFIED.);
#1080=B_SPLINE_CURVE_WITH_KNOTS('',3,(#80014,#80015,#80016,#80017,#80018,
#80019,#80020,#80021,#80022,#80023,#80024,#80025,#80026,#80027,#80028,#80029,
#80030,#80031,#80032,#80033,#80034,#80035,#80036,#80037,#80038,#80039,#80040,
#80041),.UNSPECIFIED.,.F.,.F.,(4,3,3,3,3,3,3,3,3,4),(52.0138614647296,52.1921543062006,
52.3708570227255,52.4574423721687,52.6348644963006,52.8119290116488,52.9889615116405,
53.1659777362677,53.3433764698701,53.4070747282947),.UNSPECIFIED.);
#1081=B_SPLINE_CURVE_WITH_KNOTS('',3,(#80042,#80043,#80044,#80045,#80046,
#80047,#80048,#80049,#80050),.UNSPECIFIED.,.F.,.F.,(4,1,1,1,1,1,4),(53.4070751110264,
53.4535987020309,54.4497550318931,55.4459113617553,56.4420676916176,57.4382240214798,
58.2964842709159),.UNSPECIFIED.);
#1082=B_SPLINE_CURVE_WITH_KNOTS('',3,(#80055,#80056,#80057,#80058,#80059,
#80060,#80061,#80062,#80063,#80064,#80065,#80066,#80067,#80068,#80069,#80070,
#80071,#80072,#80073,#80074,#80075,#80076,#80077,#80078,#80079,#80080,#80081,
#80082,#80083,#80084,#80085,#80086,#80087,#80088,#80089,#80090,#80091,#80092,
#80093,#80094,#80095,#80096,#80097,#80098,#80099,#80100,#80101,#80102,#80103,
#80104,#80105,#80106,#80107,#80108,#80109,#80110,#80111,#80112,#80113,#80114,
#80115,#80116,#80117,#80118,#80119,#80120,#80121,#80122,#80123,#80124,#80125,
#80126,#80127,#80128,#80129,#80130,#80131,#80132,#80133,#80134,#80135,#80136,
#80137,#80138,#80139,#80140,#80141,#80142,#80143,#80144,#80145,#80146,#80147,
#80148,#80149,#80150,#80151,#80152,#80153,#80154,#80155,#80156,#80157,#80158,
#80159,#80160,#80161,#80162,#80163,#80164,#80165,#80166,#80167,#80168,#80169,
#80170,#80171,#80172,#80173,#80174,#80175,#80176,#80177,#80178,#80179,#80180,
#80181,#80182,#80183,#80184,#80185,#80186,#80187,#80188,#80189,#80190,#80191,
#80192,#80193,#80194,#80195,#80196,#80197,#80198,#80199,#80200,#80201,#80202,
#80203,#80204,#80205,#80206,#80207,#80208,#80209,#80210,#80211,#80212,#80213,
#80214,#80215,#80216,#80217,#80218,#80219,#80220,#80221,#80222,#80223,#80224,
#80225,#80226,#80227,#80228,#80229,#80230,#80231,#80232,#80233,#80234,#80235,
#80236,#80237,#80238,#80239,#80240,#80241,#80242,#80243,#80244,#80245,#80246),
 .UNSPECIFIED.,.F.,.F.,(4,2,2,2,2,2,2,2,2,2,2,2,2,2,2,2,2,2,2,2,2,2,2,2,
2,2,2,2,2,2,2,2,2,2,2,2,2,2,2,2,2,2,2,2,2,2,2,2,2,2,2,2,2,2,2,2,2,2,2,2,
2,2,2,2,2,2,2,2,2,2,2,2,2,2,2,2,2,2,2,2,2,2,2,2,2,2,2,2,2,2,2,2,2,2,2,4),
(-2.65812282560335,-2.65609699128128,-2.64955229356263,-2.63339689211074,
-2.58207407150936,-2.56069569338651,-2.55245727120162,-2.54629043259187,
-2.54321084446186,-2.54071658851728,-2.53757615897018,-2.53109744581758,
-2.48509912782643,-2.43835965870025,-2.42995458367584,-2.42498218460008,
-2.42052997378903,-2.41482810673074,-2.40554937263751,-2.35612514627718,
-2.31506274394733,-2.30920697324126,-2.30618966912741,-2.30369261021286,
-2.30048039587027,-2.29362251326402,-2.25497219199909,-2.23716803001726,
-2.21304675727553,-2.1971548306507,-2.19082894486108,-2.18628297735503,
-2.18156429881501,-2.1743574920879,-2.15307812928642,-2.10642116379529,
-2.08635600590746,-2.07843585955492,-2.07245165207644,-2.0694083257875,
-2.06691265799576,-2.06373132326798,-2.05703873172475,-2.01391759173219,
-1.96467170210203,-1.95623993787477,-1.95126162790353,-1.94681015305105,
-1.94111757200194,-1.9318718907078,-1.88162993264105,-1.84175288919916,
-1.83562701974959,-1.83255536611484,-1.83006067600227,-1.82691105577105,
-1.82038544458358,-1.77515741683054,-1.76093619671953,-1.72696074534334,
-1.71896295912128,-1.714076913027,-1.70960311978179,-1.70383039747025,-1.69100500895248,
-1.63598476414788,-1.60600401440032,-1.59913947131505,-1.59592577583619,
-1.59366741375037,-1.59075613963496,-1.58555880492903,-1.55044120753398,
-1.5099349408516,-1.49535496976521,-1.4844335683876,-1.47887576359204,-1.47443686612957,
-1.46937346486588,-1.46054125620643,-1.41401142198338,-1.36857378073382,
-1.36205553265905,-1.35890713458109,-1.35641223781902,-1.35333886831204,
-1.34720528298511,-1.30652825722033,-1.25720599546436,-1.24792404146539,
-1.24222062929442,-1.23776750125297,-1.23279437272048,-1.22438884000068,
-1.17781105905313,-1.16393257116699),.UNSPECIFIED.);
#1083=B_SPLINE_CURVE_WITH_KNOTS('',3,(#80248,#80249,#80250,#80251,#80252,
#80253),.UNSPECIFIED.,.F.,.F.,(4,1,1,4),(58.2964842709159,58.434380351342,
59.4305366812042,59.6902579129782),.UNSPECIFIED.);
#1084=B_SPLINE_CURVE_WITH_KNOTS('',3,(#80254,#80255,#80256,#80257,#80258,
#80259,#80260,#80261,#80262,#80263,#80264,#80265,#80266,#80267,#80268,#80269,
#80270,#80271,#80272,#80273,#80274,#80275,#80276,#80277,#80278,#80279,#80280,
#80281,#80282,#80283,#80284,#80285,#80286,#80287,#80288,#80289,#80290,#80291,
#80292,#80293,#80294,#80295,#80296,#80297,#80298,#80299,#80300,#80301,#80302,
#80303,#80304,#80305,#80306,#80307,#80308,#80309,#80310,#80311,#80312,#80313,
#80314,#80315,#80316,#80317,#80318,#80319,#80320,#80321,#80322,#80323,#80324,
#80325,#80326,#80327,#80328,#80329,#80330,#80331,#80332,#80333,#80334,#80335,
#80336,#80337,#80338,#80339,#80340,#80341,#80342,#80343,#80344,#80345,#80346,
#80347,#80348,#80349,#80350,#80351,#80352,#80353,#80354,#80355,#80356,#80357,
#80358,#80359,#80360,#80361,#80362,#80363,#80364,#80365,#80366,#80367,#80368,
#80369,#80370,#80371,#80372,#80373,#80374,#80375,#80376,#80377,#80378,#80379,
#80380,#80381,#80382,#80383,#80384,#80385,#80386,#80387,#80388,#80389,#80390,
#80391,#80392,#80393,#80394,#80395,#80396,#80397,#80398,#80399,#80400,#80401,
#80402,#80403,#80404,#80405,#80406,#80407,#80408,#80409,#80410,#80411,#80412,
#80413),.UNSPECIFIED.,.F.,.F.,(4,2,2,2,2,2,2,2,2,2,2,2,2,2,2,2,2,2,2,2,
2,2,2,2,2,2,2,2,2,2,2,2,2,2,2,2,2,2,2,2,2,2,2,2,2,2,2,2,2,2,2,2,2,2,2,2,
2,2,2,2,2,2,2,2,2,2,2,2,2,2,2,2,2,2,2,2,2,2,2,4),(-2.98927830252312,-2.96007703371949,
-2.94627172720157,-2.94043632582468,-2.93602942806353,-2.93153805841539,
-2.92671432558015,-2.91900124319429,-2.89258098671331,-2.84704520996693,
-2.82333748062794,-2.81803075287548,-2.81502772865095,-2.81253080016714,
-2.80930383533054,-2.80260575670843,-2.76173416207959,-2.72719450521302,
-2.70725443875293,-2.70039854341351,-2.69575307636219,-2.69121058733973,
-2.68568869997879,-2.6719730477799,-2.60595704463375,-2.59189767154082,
-2.58274940190906,-2.57915338819893,-2.57661080786696,-2.57381939323942,
-2.56903149346558,-2.54976264042986,-2.54549026530621,-2.47961753095012,
-2.46747261778621,-2.46175968744556,-2.45730764938475,-2.45234453173439,
-2.44397768525016,-2.40087635545215,-2.36421314368282,-2.34763317326389,
-2.34320235560184,-2.34048911236113,-2.33793773003614,-2.33415050794017,
-2.32442998449772,-2.27298913602557,-2.24840100875826,-2.23745049704346,
-2.22857202021463,-2.2235005399539,-2.21906521324565,-2.21352594924394,
-2.20231873073976,-2.14550632849385,-2.11495651631871,-2.10803575456699,
-2.10481253480691,-2.10255399373007,-2.09965173184545,-2.09449111839401,
-2.0622021565422,-2.0579190497288,-2.02874782315065,-2.00865073859859,-1.99465383451477,
-1.98862248674134,-1.98412693369933,-1.97931182704577,-1.9716413137151,
-1.9459971387455,-1.8819292548182,-1.87228165100106,-1.86861162301658,-1.86605609540221,
-1.86329368678732,-1.85863965119246,-1.84129763632644,-1.8262871493728),
 .UNSPECIFIED.);
#1085=B_SPLINE_CURVE_WITH_KNOTS('',3,(#80419,#80420,#80421,#80422,#80423,
#80424,#80425,#80426,#80427,#80428,#80429,#80430,#80431,#80432,#80433,#80434,
#80435,#80436,#80437,#80438,#80439,#80440,#80441,#80442,#80443,#80444,#80445,
#80446,#80447,#80448,#80449,#80450,#80451,#80452,#80453,#80454,#80455,#80456,
#80457,#80458,#80459,#80460,#80461,#80462,#80463,#80464,#80465,#80466,#80467,
#80468,#80469,#80470,#80471,#80472,#80473,#80474,#80475,#80476,#80477,#80478,
#80479,#80480,#80481,#80482,#80483,#80484,#80485,#80486,#80487,#80488,#80489,
#80490,#80491,#80492,#80493,#80494,#80495,#80496,#80497,#80498,#80499,#80500,
#80501,#80502,#80503,#80504,#80505,#80506,#80507,#80508,#80509,#80510,#80511,
#80512,#80513,#80514,#80515,#80516,#80517,#80518,#80519,#80520,#80521,#80522,
#80523,#80524,#80525,#80526,#80527,#80528,#80529,#80530,#80531,#80532,#80533,
#80534,#80535,#80536,#80537,#80538,#80539,#80540,#80541,#80542,#80543,#80544,
#80545,#80546,#80547,#80548,#80549,#80550,#80551,#80552,#80553,#80554,#80555,
#80556,#80557,#80558,#80559,#80560,#80561,#80562,#80563,#80564,#80565,#80566,
#80567,#80568,#80569,#80570,#80571,#80572,#80573,#80574,#80575,#80576),
 .UNSPECIFIED.,.F.,.F.,(4,2,2,2,2,2,2,2,2,2,2,2,2,2,2,2,2,2,2,2,2,2,2,2,
2,2,2,2,2,2,2,2,2,2,2,2,2,2,2,2,2,2,2,2,2,2,2,2,2,2,2,2,2,2,2,2,2,2,2,2,
2,2,2,2,2,2,2,2,2,2,2,2,2,2,2,2,2,2,4),(-1.16355052402537,-1.11305031683564,
-1.10152596335983,-1.09592528045025,-1.09148272382327,-1.08644784742858,
-1.07775055560716,-1.03061364858019,-0.985569135421594,-0.979032311349418,
-0.975880384273367,-0.973385441481947,-0.970315406463096,-0.964198472860405,
-0.92512811681522,-0.874022662882113,-0.864822853670405,-0.859143163638298,
-0.854692692973826,-0.849706086437886,-0.841236835269212,-0.79201087328454,
-0.748883051222585,-0.742184258743587,-0.739001515207173,-0.736505506455984,
-0.733462679148961,-0.727482093872668,-0.719569348803431,-0.699535464588616,
-0.652977667494132,-0.631614703220788,-0.624398752927781,-0.619677750668199,
-0.615132218307279,-0.608811362045385,-0.592957825392288,-0.568921095850618,
-0.52315079265491,-0.508155617381412,-0.50371899288127,-0.501003453474276,
-0.498420638942382,-0.494608572700817,-0.483940387963933,-0.466392730706132,
-0.413273339262541,-0.394171618112931,-0.38720759832878,-0.383004907155321,
-0.378489423675612,-0.372344420091701,-0.357648890096711,-0.336116874575393,
-0.293888591595522,-0.272185266102778,-0.267253496571308,-0.264429985420716,
-0.261897136644301,-0.258368366494303,-0.249663408043189,-0.236553980462424,
-0.183645076248432,-0.158706404247294,-0.151054888756445,-0.146242199275311,
-0.141742374417978,-0.135695240735358,-0.121613073214625,-0.10134426098883,
-0.065061020047664,-0.0415041796078312,-0.0326900434510546,-0.0290461462357153,
-0.0265196476117824,-0.0241882205948804,-0.0214282766404578,-0.0173833660770604,
-0.000695720168090065),.UNSPECIFIED.);
#1086=B_SPLINE_CURVE_WITH_KNOTS('',3,(#80577,#80578,#80579,#80580,#80581,
#80582,#80583,#80584,#80585,#80586,#80587,#80588,#80589,#80590,#80591,#80592,
#80593,#80594,#80595,#80596,#80597,#80598,#80599,#80600,#80601,#80602,#80603,
#80604,#80605,#80606,#80607,#80608,#80609,#80610,#80611,#80612,#80613,#80614,
#80615,#80616,#80617,#80618,#80619,#80620,#80621,#80622),.UNSPECIFIED.,
 .F.,.F.,(4,2,2,2,2,2,2,2,2,2,2,2,2,2,2,2,2,2,2,2,2,2,4),(-2.98951265346651,
-2.98409967932115,-2.91825065185881,-2.90610864682674,-2.90039505197607,
-2.89594160028733,-2.89097595314149,-2.88260239747836,-2.84093330960873,
-2.81069275544095,-2.7947630285004,-2.78793211548667,-2.7827841882569,-2.7798871036176,
-2.777388936278,-2.77415583531056,-2.76743020143402,-2.72751422494492,-2.69232778408112,
-2.67217175728409,-2.66528917333918,-2.66063715892619,-2.65812282560335),
 .UNSPECIFIED.);
#1087=B_SPLINE_CURVE_WITH_KNOTS('',3,(#80623,#80624,#80625,#80626,#80627,
#80628,#80629,#80630,#80631,#80632,#80633,#80634,#80635,#80636,#80637,#80638,
#80639,#80640,#80641,#80642,#80643,#80644,#80645,#80646,#80647,#80648,#80649,
#80650,#80651,#80652,#80653,#80654,#80655,#80656,#80657,#80658,#80659,#80660,
#80661,#80662,#80663,#80664,#80665,#80666,#80667,#80668,#80669,#80670,#80671,
#80672,#80673,#80674,#80675,#80676,#80677,#80678,#80679,#80680,#80681,#80682,
#80683,#80684,#80685,#80686,#80687,#80688,#80689,#80690,#80691,#80692,#80693,
#80694,#80695,#80696,#80697,#80698,#80699,#80700,#80701,#80702,#80703,#80704,
#80705,#80706,#80707,#80708,#80709,#80710,#80711,#80712,#80713,#80714,#80715,
#80716,#80717,#80718,#80719,#80720,#80721,#80722,#80723,#80724,#80725,#80726,
#80727,#80728,#80729,#80730,#80731,#80732,#80733,#80734,#80735,#80736,#80737,
#80738,#80739,#80740,#80741,#80742,#80743,#80744,#80745,#80746,#80747,#80748,
#80749,#80750,#80751,#80752,#80753,#80754,#80755,#80756,#80757,#80758,#80759,
#80760,#80761,#80762,#80763,#80764,#80765,#80766,#80767,#80768,#80769,#80770,
#80771,#80772,#80773,#80774,#80775,#80776,#80777,#80778,#80779,#80780,#80781,
#80782,#80783,#80784,#80785,#80786,#80787,#80788,#80789,#80790,#80791,#80792,
#80793,#80794,#80795,#80796,#80797,#80798,#80799,#80800,#80801,#80802,#80803,
#80804,#80805,#80806,#80807,#80808,#80809,#80810,#80811,#80812,#80813,#80814,
#80815,#80816,#80817,#80818,#80819,#80820),.UNSPECIFIED.,.F.,.F.,(4,2,2,
2,2,2,2,2,2,2,2,2,2,2,2,2,2,2,2,2,2,2,2,2,2,2,2,2,2,2,2,2,2,2,2,2,2,2,2,
2,2,2,2,2,2,2,2,2,2,2,2,2,2,2,2,2,2,2,2,2,2,2,2,2,2,2,2,2,2,2,2,2,2,2,2,
2,2,2,2,2,2,2,2,2,2,2,2,2,2,2,2,2,2,2,2,2,2,2,4),(-1.8262871493728,-1.80231153183424,
-1.76317482492192,-1.75458341261169,-1.74957200192133,-1.74512764668482,
-1.73949430107403,-1.73045098226865,-1.67708805318982,-1.63952445875179,
-1.63366206118258,-1.63064371219958,-1.62814720372425,-1.62493760734453,
-1.61809210874062,-1.57885366766302,-1.54321036276671,-1.52957411040255,
-1.51906339441778,-1.51365803596146,-1.50922989415587,-1.5040540523161,
-1.49493674754578,-1.48342831534252,-1.45679658909519,-1.41757600249844,
-1.40051642176199,-1.39588458032644,-1.39312690873883,-1.3905688321058,
-1.38688535720896,-1.37714522893103,-1.31287498189162,-1.28761151980343,
-1.27993194034675,-1.27511452193528,-1.27061909236573,-1.26459140667491,
-1.25062010980713,-1.2305730718803,-1.20129097680454,-1.19694774515022,
-1.16467323340541,-1.15951111923406,-1.15660829078806,-1.15434944133921,
-1.15112602167638,-1.14420561004622,-1.11366484499995,-1.05686365683889,
-1.04566575910983,-1.04012777584703,-1.03569194194172,-1.03061821398927,
-1.02173142218677,-1.01076702095896,-0.986131013649406,-0.934426257952615,
-0.924901040653196,-0.921144895470947,-0.918599012583689,-0.915875003085733,
-0.911396556173234,-0.894230505109473,-0.854880502643915,-0.815140363222623,
-0.806794432270155,-0.801835142114099,-0.797381233503409,-0.791658504462818,
-0.779463359793706,-0.74811391703015,-0.693256936246748,-0.686566635393643,
-0.683386101912153,-0.680890962640978,-0.677848233663168,-0.671865222917363,
-0.640466832042411,-0.585326097563374,-0.573891800094391,-0.568225906993194,
-0.564061034403986,-0.55952030999714,-0.553219711707989,-0.537494340710455,
-0.513740587855433,-0.468351771957618,-0.452650916068628,-0.448149534932015,
-0.445420442114275,-0.442847332738486,-0.439082302120109,-0.428758307467109,
-0.412035592363433,-0.381659463879675,-0.341395124898333,-0.333023989020014,
-0.33210769087985),.UNSPECIFIED.);
#1088=B_SPLINE_CURVE_WITH_KNOTS('',3,(#80825,#80826,#80827,#80828,#80829,
#80830,#80831,#80832,#80833,#80834,#80835,#80836,#80837,#80838,#80839,#80840,
#80841,#80842,#80843,#80844,#80845,#80846,#80847,#80848,#80849,#80850,#80851,
#80852,#80853,#80854,#80855,#80856,#80857,#80858,#80859,#80860,#80861,#80862,
#80863,#80864,#80865,#80866,#80867,#80868,#80869,#80870,#80871,#80872,#80873,
#80874,#80875,#80876,#80877,#80878,#80879,#80880,#80881,#80882,#80883,#80884,
#80885,#80886,#80887,#80888,#80889,#80890,#80891,#80892,#80893,#80894,#80895,
#80896,#80897,#80898,#80899,#80900,#80901,#80902,#80903,#80904,#80905,#80906,
#80907,#80908,#80909,#80910,#80911,#80912,#80913,#80914,#80915,#80916,#80917,
#80918,#80919,#80920,#80921,#80922,#80923,#80924,#80925,#80926,#80927,#80928,
#80929,#80930,#80931,#80932,#80933,#80934,#80935,#80936,#80937,#80938,#80939,
#80940,#80941,#80942,#80943,#80944,#80945,#80946,#80947,#80948,#80949,#80950,
#80951,#80952,#80953,#80954,#80955,#80956,#80957,#80958,#80959,#80960,#80961,
#80962,#80963,#80964,#80965,#80966,#80967,#80968,#80969,#80970,#80971,#80972,
#80973,#80974,#80975,#80976,#80977,#80978,#80979,#80980,#80981,#80982,#80983,
#80984,#80985,#80986,#80987,#80988,#80989,#80990,#80991,#80992,#80993,#80994,
#80995,#80996,#80997,#80998,#80999,#81000,#81001,#81002,#81003,#81004,#81005,
#81006,#81007,#81008,#81009,#81010,#81011,#81012,#81013,#81014,#81015,#81016,
#81017,#81018,#81019,#81020,#81021,#81022),.UNSPECIFIED.,.F.,.F.,(4,2,2,
2,2,2,2,2,2,2,2,2,2,2,2,2,2,2,2,2,2,2,2,2,2,2,2,2,2,2,2,2,2,2,2,2,2,2,2,
2,2,2,2,2,2,2,2,2,2,2,2,2,2,2,2,2,2,2,2,2,2,2,2,2,2,2,2,2,2,2,2,2,2,2,2,
2,2,2,2,2,2,2,2,2,2,2,2,2,2,2,2,2,2,2,2,2,2,2,4),(-2.65781287416919,-2.64452458263601,
-2.63763443226677,-2.6344163790306,-2.63215791714073,-2.62925068407198,
-2.62406985834844,-2.58961924028388,-2.56330650341922,-2.54024357241541,
-2.52972695456487,-2.5211225969632,-2.51610793400733,-2.51166322141039,
-2.50603280806457,-2.49700118311198,-2.44351098074392,-2.40644724033001,
-2.40035087378956,-2.39728523066004,-2.39479057739968,-2.3916348901716,
-2.38507677746596,-2.32962104463382,-2.29199842368044,-2.28383444530008,
-2.27891335216599,-2.27444973177503,-2.26874847442395,-2.25925642730268,
-2.1954186295027,-2.17662729409528,-2.16902820931757,-2.16323075013755,
-2.16022522160023,-2.15772714908705,-2.15449981001434,-2.14756081804742,
-2.11213657532916,-2.07385580968631,-2.05272779956298,-2.04573496809047,
-2.04106023952762,-2.03653656997462,-2.03008359002822,-2.01443384402534,
-1.96258581996294,-1.94106195088109,-1.93278861124956,-1.92660168798422,
-1.92351790494313,-1.92102341739039,-1.91788667059428,-1.91142827520871,
-1.86514624005752,-1.81937373430837,-1.81057139679469,-1.80551446017698,
-1.80107501721763,-1.79550830048053,-1.78669640842405,-1.73090798214196,
-1.69559636414734,-1.68957275138425,-1.68652136761554,-1.68402583644888,
-1.68085321850392,-1.67420755885897,-1.63070156683914,-1.58229125606155,
-1.57357002651287,-1.5685300904386,-1.56408822303984,-1.55849531224362,
-1.54959423227013,-1.49466742663082,-1.4872583395619,-1.45730012689484,
-1.45215228713223,-1.44925201259168,-1.44699168114663,-1.44376152696734,
-1.43680844822086,-1.40595251031668,-1.34812381945398,-1.33881054290913,
-1.33309820891804,-1.32864418493815,-1.32367630115275,-1.315295037307,-1.27019914879147,
-1.22214161567689,-1.21585191515742,-1.21274778148194,-1.21025330736599,
-1.20713713731564,-1.20078575746744,-1.17550652352677,-1.16355052402537),
 .UNSPECIFIED.);
#1089=B_SPLINE_CURVE_WITH_KNOTS('',3,(#81024,#81025,#81026,#81027,#81028,
#81029,#81030,#81031,#81032,#81033,#81034,#81035,#81036,#81037,#81038,#81039,
#81040,#81041,#81042,#81043,#81044,#81045,#81046,#81047,#81048,#81049,#81050,
#81051,#81052,#81053,#81054,#81055,#81056,#81057,#81058,#81059,#81060,#81061,
#81062,#81063,#81064,#81065,#81066,#81067,#81068,#81069,#81070,#81071),
 .UNSPECIFIED.,.F.,.F.,(4,2,2,2,2,2,2,2,2,2,2,2,2,2,2,2,2,2,2,2,2,2,2,4),
(-0.33210769087985,-0.328059088261506,-0.323605902234908,-0.31789213185177,
-0.305748148990684,-0.276217211565336,-0.259902966633279,-0.219658665821679,
-0.212943503580916,-0.209712607696378,-0.207214780482136,-0.204349414940198,
-0.199210667556835,-0.192416821766954,-0.176619567210251,-0.146253599696267,
-0.10453081021936,-0.0961590965829314,-0.0911940749908607,-0.0867409169303314,
-0.0810273722970079,-0.0688846258861045,-0.039398452645496,-0.000697109447201426),
 .UNSPECIFIED.);
#1090=B_SPLINE_CURVE_WITH_KNOTS('',3,(#81072,#81073,#81074,#81075,#81076,
#81077,#81078,#81079,#81080,#81081,#81082,#81083,#81084,#81085,#81086,#81087,
#81088,#81089,#81090,#81091,#81092,#81093,#81094,#81095,#81096,#81097,#81098,
#81099,#81100,#81101,#81102,#81103,#81104,#81105,#81106,#81107,#81108,#81109,
#81110,#81111,#81112,#81113,#81114,#81115,#81116,#81117,#81118,#81119,#81120,
#81121,#81122,#81123,#81124,#81125,#81126,#81127,#81128,#81129,#81130,#81131,
#81132,#81133,#81134,#81135,#81136,#81137,#81138,#81139,#81140,#81141,#81142,
#81143,#81144,#81145,#81146,#81147,#81148,#81149,#81150,#81151,#81152,#81153,
#81154,#81155,#81156,#81157,#81158,#81159,#81160,#81161,#81162,#81163,#81164,
#81165,#81166,#81167,#81168,#81169,#81170,#81171,#81172,#81173,#81174,#81175,
#81176,#81177,#81178,#81179,#81180,#81181,#81182,#81183,#81184,#81185,#81186,
#81187,#81188,#81189,#81190,#81191,#81192,#81193,#81194,#81195,#81196,#81197,
#81198,#81199,#81200,#81201,#81202,#81203,#81204,#81205,#81206,#81207,#81208,
#81209,#81210,#81211,#81212,#81213,#81214,#81215,#81216,#81217,#81218,#81219,
#81220,#81221,#81222,#81223,#81224,#81225,#81226,#81227,#81228,#81229,#81230,
#81231,#81232,#81233,#81234,#81235),.UNSPECIFIED.,.F.,.F.,(4,2,2,2,2,2,
2,2,2,2,2,2,2,2,2,2,2,2,2,2,2,2,2,2,2,2,2,2,2,2,2,2,2,2,2,2,2,2,2,2,2,2,
2,2,2,2,2,2,2,2,2,2,2,2,2,2,2,2,2,2,2,2,2,2,2,2,2,2,2,2,2,2,2,2,2,2,2,2,
2,2,2,4),(-2.98939743642882,-2.96835144039151,-2.9647712532952,-2.96219240493113,
-2.95983841105715,-2.95746526525625,-2.95340026082852,-2.94167647306,-2.91588423164734,
-2.86658934259498,-2.85168263796954,-2.84550571718206,-2.84098586649046,
-2.83622166805944,-2.82879551810349,-2.80545418853011,-2.75655623314502,
-2.73962359178398,-2.72921181604712,-2.7254346039411,-2.72285901348154,
-2.72013352220118,-2.71564940110566,-2.70014088060965,-2.65469733861,-2.63086652725387,
-2.61510458520335,-2.60879819721514,-2.60425606021241,-2.59953246006995,
-2.59230030085221,-2.57077638517103,-2.52431636916258,-2.50430537704207,
-2.49639864036218,-2.49042224854389,-2.48738068552722,-2.48488524393333,
-2.4817027474507,-2.47500294878607,-2.43192614339766,-2.41853940276316,
-2.39425261496233,-2.37828663069864,-2.37195011035848,-2.3674024978012,
-2.36268737663663,-2.35549660725407,-2.33436986387042,-2.28756598933452,
-2.26745652904114,-2.25952532087595,-2.25353473207695,-2.25049024547462,
-2.24799483986087,-2.24481547920095,-2.23813268746026,-2.18326252362536,
-2.14524523089891,-2.13706533189525,-2.13214087507022,-2.12767817400871,
-2.12198357181017,-2.10960490711176,-2.05408794301891,-2.02394370074289,
-2.01706266851227,-2.01384615013527,-2.01158772873051,-2.00867917593621,
-2.0034930462812,-1.96881826720647,-1.96719841414491,-1.93881374806733,
-1.91809286439524,-1.90378779879486,-1.8977053555061,-1.89320059286199,
-1.88898272223026,-1.88193359129712,-1.86212851150957,-1.82653497020089),
 .UNSPECIFIED.);
#1091=B_SPLINE_CURVE_WITH_KNOTS('',3,(#81241,#81242,#81243,#81244,#81245,
#81246,#81247,#81248,#81249,#81250,#81251,#81252,#81253,#81254,#81255,#81256,
#81257,#81258,#81259,#81260,#81261,#81262,#81263,#81264,#81265,#81266,#81267,
#81268,#81269,#81270,#81271,#81272,#81273,#81274,#81275,#81276,#81277,#81278,
#81279,#81280,#81281,#81282,#81283,#81284,#81285,#81286,#81287,#81288,#81289,
#81290,#81291,#81292,#81293,#81294,#81295,#81296,#81297,#81298,#81299,#81300,
#81301,#81302,#81303,#81304,#81305,#81306,#81307,#81308,#81309,#81310,#81311,
#81312,#81313,#81314,#81315,#81316,#81317,#81318,#81319,#81320,#81321,#81322,
#81323,#81324,#81325,#81326,#81327,#81328,#81329,#81330,#81331,#81332,#81333,
#81334,#81335,#81336,#81337,#81338,#81339,#81340,#81341,#81342,#81343,#81344,
#81345,#81346,#81347,#81348,#81349,#81350,#81351,#81352,#81353,#81354,#81355,
#81356,#81357,#81358,#81359,#81360,#81361,#81362,#81363,#81364,#81365,#81366,
#81367,#81368,#81369,#81370,#81371,#81372,#81373,#81374,#81375,#81376,#81377,
#81378,#81379,#81380,#81381,#81382,#81383,#81384,#81385,#81386,#81387,#81388),
 .UNSPECIFIED.,.F.,.F.,(4,2,2,2,2,2,2,2,2,2,2,2,2,2,2,2,2,2,2,2,2,2,2,2,
2,2,2,2,2,2,2,2,2,2,2,2,2,2,2,2,2,2,2,2,2,2,2,2,2,2,2,2,2,2,2,2,2,2,2,2,
2,2,2,2,2,2,2,2,2,2,2,2,2,4),(-1.16384962784558,-1.13264335480885,-1.07715530874494,
-1.07059133960003,-1.06743397258959,-1.06493857029011,-1.06187270615642,
-1.0557779741105,-1.01892944759953,-0.965199630107386,-0.956188937264403,
-0.950563649251036,-0.946118225201842,-0.941097731460923,-0.932470567389394,
-0.921917960664898,-0.898734552015196,-0.871842118459206,-0.838060186815542,
-0.832887368854638,-0.829981362007405,-0.827721775901371,-0.824499479219632,
-0.817589829347381,-0.787169934316597,-0.730758840244741,-0.719212225213826,
-0.713607026565303,-0.709163647339682,-0.704130774896473,-0.695444530628105,
-0.684798810565613,-0.661292250463344,-0.634801420664341,-0.601144198999232,
-0.595972829888898,-0.593067215233445,-0.590807670862498,-0.587585090621078,
-0.580673498084995,-0.55023286625569,-0.493754106648572,-0.482269168287115,
-0.476675636536854,-0.472233474315141,-0.467193412963167,-0.458472563350708,
-0.410693023895285,-0.366384122349361,-0.359809939061885,-0.356650751067447,
-0.354155460181701,-0.351091641407931,-0.345006552785591,-0.309055812988115,
-0.254217043324424,-0.245314970891639,-0.239721543313514,-0.235279364284549,
-0.230239177579371,-0.221517835180842,-0.175626962922634,-0.129244721292173,
-0.122789592906387,-0.119653223917238,-0.117158420905985,-0.114073477391005,
-0.107881932826869,-0.0996017141090048,-0.0780501408867098,-0.0249406429271444,
-0.0102564647077087,-0.00445491911353678,-0.000696437445735352),
 .UNSPECIFIED.);
#1092=B_SPLINE_CURVE_WITH_KNOTS('',3,(#81389,#81390,#81391,#81392,#81393,
#81394,#81395,#81396,#81397,#81398,#81399,#81400,#81401,#81402,#81403,#81404,
#81405,#81406,#81407,#81408,#81409,#81410,#81411,#81412,#81413,#81414,#81415,
#81416,#81417,#81418,#81419,#81420,#81421,#81422,#81423,#81424,#81425,#81426,
#81427,#81428),.UNSPECIFIED.,.F.,.F.,(4,2,2,2,2,2,2,2,2,2,2,2,2,2,2,2,2,
2,2,4),(-2.98908128197759,-2.98562339621579,-2.98018070717797,-2.96981470620473,
-2.92242024352145,-2.88025232492701,-2.87410391415925,-2.87102811807109,
-2.86853398070648,-2.86538998549565,-2.85889195534857,-2.81319177366175,
-2.76619866467017,-2.75779080014898,-2.75281805627472,-2.74836633530827,
-2.74266620295889,-2.73059757337088,-2.67476448383729,-2.65781287416919),
 .UNSPECIFIED.);
#1093=B_SPLINE_CURVE_WITH_KNOTS('',3,(#81429,#81430,#81431,#81432,#81433,
#81434,#81435,#81436,#81437,#81438,#81439,#81440,#81441,#81442,#81443,#81444,
#81445,#81446,#81447,#81448,#81449,#81450,#81451,#81452,#81453,#81454,#81455,
#81456,#81457,#81458,#81459,#81460,#81461,#81462,#81463,#81464,#81465,#81466,
#81467,#81468,#81469,#81470,#81471,#81472,#81473,#81474,#81475,#81476,#81477,
#81478,#81479,#81480,#81481,#81482,#81483,#81484,#81485,#81486,#81487,#81488,
#81489,#81490,#81491,#81492,#81493,#81494,#81495,#81496,#81497,#81498,#81499,
#81500,#81501,#81502,#81503,#81504,#81505,#81506,#81507,#81508,#81509,#81510,
#81511,#81512,#81513,#81514,#81515,#81516,#81517,#81518,#81519,#81520,#81521,
#81522,#81523,#81524,#81525,#81526,#81527,#81528,#81529,#81530,#81531,#81532,
#81533,#81534,#81535,#81536,#81537,#81538,#81539,#81540,#81541,#81542,#81543,
#81544,#81545,#81546,#81547,#81548,#81549,#81550,#81551,#81552,#81553,#81554,
#81555,#81556,#81557,#81558,#81559,#81560,#81561,#81562,#81563,#81564,#81565,
#81566,#81567,#81568,#81569,#81570,#81571,#81572,#81573,#81574,#81575,#81576,
#81577,#81578,#81579,#81580,#81581,#81582,#81583,#81584,#81585,#81586,#81587,
#81588,#81589,#81590,#81591,#81592,#81593,#81594,#81595,#81596,#81597,#81598,
#81599,#81600,#81601,#81602,#81603,#81604,#81605,#81606,#81607,#81608,#81609,
#81610,#81611,#81612,#81613,#81614,#81615,#81616,#81617,#81618,#81619,#81620,
#81621,#81622,#81623,#81624,#81625,#81626,#81627,#81628,#81629,#81630,#81631,
#81632,#81633,#81634),.UNSPECIFIED.,.F.,.F.,(4,2,2,2,2,2,2,2,2,2,2,2,2,
2,2,2,2,2,2,2,2,2,2,2,2,2,2,2,2,2,2,2,2,2,2,2,2,2,2,2,2,2,2,2,2,2,2,2,2,
2,2,2,2,2,2,2,2,2,2,2,2,2,2,2,2,2,2,2,2,2,2,2,2,2,2,2,2,2,2,2,2,2,2,2,2,
2,2,2,2,2,2,2,2,2,2,2,2,2,2,2,2,2,4),(-1.82653497020089,-1.80970112590821,
-1.79223671915726,-1.78160366613386,-1.77779654584285,-1.77521499236538,
-1.77283311144874,-1.76872392079423,-1.75665454088319,-1.71373795786615,
-1.67162914340665,-1.66331574795128,-1.65836263079241,-1.65390612043639,
-1.64816863631824,-1.63633962047401,-1.58037622390727,-1.5500883571337,
-1.54319246721,-1.53997305408032,-1.53771417055892,-1.5348072324978,-1.52962889991144,
-1.49537729579061,-1.43656226837672,-1.42810495650653,-1.4226429597602,
-1.41821132711221,-1.41307957725786,-1.40391956544992,-1.39251914782045,
-1.3662945897991,-1.32810688953579,-1.30957141369085,-1.30482950014318,
-1.30204754187357,-1.29949989274249,-1.29587758674125,-1.28655857555477,
-1.27213009987825,-1.21883910084207,-1.19588830545804,-1.18850229049503,
-1.18374628345475,-1.17922171494027,-1.17301839267407,-1.15794298019146,
-1.13560674937987,-1.10851324759428,-1.07357300437759,-1.06838069201022,
-1.06547076784632,-1.06321254212297,-1.05999800865932,-1.05312766154127,
-1.02308871631241,-0.967877693020767,-0.955247820130009,-0.949509277762876,
-0.945040663176737,-0.940138728298648,-0.932064768603922,-0.896549822177602,
-0.851311238800805,-0.835306948598925,-0.830778069511122,-0.828042671806354,
-0.825472451545619,-0.821724346534809,-0.811526696793529,-0.795103250329995,
-0.764916273838363,-0.724067180882814,-0.715648247158712,-0.710672661396939,
-0.706220696233654,-0.700523478843023,-0.688474018259306,-0.644969752440523,
-0.602092906725322,-0.595362899456894,-0.592174485393937,-0.589678522256883,
-0.586641333543003,-0.580687761865217,-0.572821570930227,-0.552975160005654,
-0.490249253756482,-0.481024746731182,-0.475338339429444,-0.470887707456453,
-0.465906243441543,-0.457459094231963,-0.447187788532852,-0.424961487981722,
-0.397763238210572,-0.36275099754082,-0.35755692854549,-0.354646635873784,
-0.352388506059758,-0.349174606164239,-0.342307530389767,-0.332036819262125),
 .UNSPECIFIED.);
#1094=B_SPLINE_CURVE_WITH_KNOTS('',3,(#81639,#81640,#81641,#81642,#81643,
#81644,#81645,#81646,#81647,#81648,#81649,#81650,#81651,#81652,#81653,#81654,
#81655,#81656,#81657,#81658,#81659,#81660,#81661,#81662,#81663,#81664,#81665,
#81666,#81667,#81668,#81669,#81670,#81671,#81672,#81673,#81674,#81675,#81676,
#81677,#81678,#81679,#81680,#81681,#81682,#81683,#81684,#81685,#81686,#81687,
#81688,#81689,#81690,#81691,#81692,#81693,#81694,#81695,#81696,#81697,#81698,
#81699,#81700,#81701,#81702,#81703,#81704,#81705,#81706,#81707,#81708,#81709,
#81710,#81711,#81712,#81713,#81714,#81715,#81716,#81717,#81718,#81719,#81720,
#81721,#81722,#81723,#81724,#81725,#81726,#81727,#81728,#81729,#81730,#81731,
#81732,#81733,#81734,#81735,#81736,#81737,#81738,#81739,#81740,#81741,#81742,
#81743,#81744,#81745,#81746,#81747,#81748,#81749,#81750,#81751,#81752,#81753,
#81754,#81755,#81756,#81757,#81758,#81759,#81760,#81761,#81762,#81763,#81764,
#81765,#81766,#81767,#81768,#81769,#81770,#81771,#81772,#81773,#81774,#81775,
#81776,#81777,#81778,#81779,#81780,#81781,#81782,#81783,#81784,#81785,#81786,
#81787,#81788,#81789,#81790,#81791,#81792,#81793,#81794,#81795,#81796,#81797,
#81798,#81799,#81800,#81801,#81802,#81803,#81804,#81805,#81806,#81807,#81808,
#81809,#81810,#81811,#81812,#81813,#81814,#81815,#81816,#81817,#81818,#81819,
#81820,#81821,#81822,#81823,#81824,#81825,#81826,#81827,#81828),
 .UNSPECIFIED.,.F.,.F.,(4,2,2,2,2,2,2,2,2,2,2,2,2,2,2,2,2,2,2,2,2,2,2,2,
2,2,2,2,2,2,2,2,2,2,2,2,2,2,2,2,2,2,2,2,2,2,2,2,2,2,2,2,2,2,2,2,2,2,2,2,
2,2,2,2,2,2,2,2,2,2,2,2,2,2,2,2,2,2,2,2,2,2,2,2,2,2,2,2,2,2,2,2,2,2,4),
(-2.65823196508423,-2.62110632888272,-2.61260737370035,-2.60761486878515,
-2.60316612921432,-2.59749825886872,-2.58833798236918,-2.53654601965269,
-2.49804054988087,-2.49192895580075,-2.48886017720573,-2.48636546161178,
-2.48321283390219,-2.47667132807758,-2.43180034859266,-2.38404627703729,
-2.37562801733836,-2.37065256201901,-2.3662005135559,-2.36050287082104,
-2.35123965814575,-2.30140043264854,-2.26115885295507,-2.25502920647947,
-2.25195679406253,-2.2494621128433,-2.24631329017173,-2.23979187175334,
-2.19447794775182,-2.14712476661639,-2.13871097780566,-2.13373640570348,
-2.12928407254857,-2.12358457635096,-2.11431514562047,-2.06462207977832,
-2.02424534077738,-2.01811417731508,-2.01504142661204,-2.01254669968366,
-2.00939810899445,-2.00287812134408,-1.95753201883435,-1.91074393192334,
-1.90203820104005,-1.89700165348496,-1.89255949656753,-1.88696183311689,
-1.87804410547757,-1.82329139556471,-1.78724515641804,-1.78115848851448,
-1.7780945186559,-1.77559945337939,-1.77244100577951,-1.76586982460099,
-1.72157259258723,-1.67410050420845,-1.66523473290619,-1.66016431823936,
-1.655726314816,-1.65017891756596,-1.64143325680447,-1.57637817630137,-1.55747048118079,
-1.54984112311895,-1.54402573878985,-1.54101627206618,-1.53851808255814,
-1.53529464053577,-1.52837837356498,-1.49536490985464,-1.43847530064763,
-1.42978861385701,-1.42425835965677,-1.41982145750941,-1.41473856344693,
-1.40581438615714,-1.3947916545609,-1.36995071078761,-1.3166640969491,-1.30854201286324,
-1.30534551307528,-1.30278805391383,-1.30008043360708,-1.29568022180041,
-1.27948573374916,-1.24448601134699,-1.20304942653334,-1.19355766283247,
-1.18785570882297,-1.18339107176011,-1.17846837607184,-1.17030063341044,
-1.16384962784558),.UNSPECIFIED.);
#1095=B_SPLINE_CURVE_WITH_KNOTS('',3,(#81830,#81831,#81832,#81833,#81834,
#81835,#81836,#81837,#81838,#81839,#81840,#81841,#81842,#81843,#81844,#81845,
#81846,#81847,#81848,#81849,#81850,#81851,#81852,#81853,#81854,#81855,#81856,
#81857,#81858,#81859,#81860,#81861,#81862,#81863,#81864,#81865,#81866,#81867,
#81868,#81869,#81870,#81871),.UNSPECIFIED.,.F.,.F.,(4,2,2,2,2,2,2,2,2,2,
2,2,2,2,2,2,2,2,2,2,4),(-0.332036819262125,-0.312300142779555,-0.257186157337942,
-0.244467488921226,-0.238713611913341,-0.23424293479366,-0.229348731392269,
-0.22131084064477,-0.186545904668108,-0.159874092150857,-0.125791004616353,
-0.120615431454693,-0.117709309595276,-0.115450563461532,-0.112230764800162,
-0.105331638943737,-0.0750080527306256,-0.0161391283607585,-0.00623627656673708,
-0.00289603065962882,-0.000696476426962337),.UNSPECIFIED.);
#1096=B_SPLINE_CURVE_WITH_KNOTS('',3,(#81872,#81873,#81874,#81875,#81876,
#81877,#81878,#81879,#81880,#81881,#81882,#81883,#81884,#81885,#81886,#81887,
#81888,#81889,#81890,#81891,#81892,#81893,#81894,#81895,#81896,#81897,#81898,
#81899,#81900,#81901,#81902,#81903,#81904,#81905,#81906,#81907,#81908,#81909,
#81910,#81911,#81912,#81913,#81914,#81915,#81916,#81917,#81918,#81919,#81920,
#81921,#81922,#81923,#81924,#81925,#81926,#81927,#81928,#81929,#81930,#81931,
#81932,#81933,#81934,#81935,#81936,#81937,#81938,#81939,#81940,#81941,#81942,
#81943,#81944,#81945,#81946,#81947,#81948,#81949,#81950,#81951,#81952,#81953,
#81954,#81955,#81956,#81957,#81958,#81959,#81960,#81961,#81962,#81963,#81964,
#81965,#81966,#81967,#81968,#81969,#81970,#81971,#81972,#81973,#81974,#81975,
#81976,#81977,#81978,#81979,#81980,#81981,#81982,#81983,#81984,#81985,#81986,
#81987,#81988,#81989,#81990,#81991,#81992,#81993,#81994,#81995,#81996,#81997,
#81998,#81999,#82000,#82001,#82002,#82003,#82004,#82005,#82006,#82007,#82008,
#82009,#82010,#82011,#82012,#82013,#82014,#82015,#82016,#82017,#82018,#82019,
#82020,#82021,#82022,#82023,#82024,#82025,#82026,#82027,#82028,#82029,#82030,
#82031),.UNSPECIFIED.,.F.,.F.,(4,2,2,2,2,2,2,2,2,2,2,2,2,2,2,2,2,2,2,2,
2,2,2,2,2,2,2,2,2,2,2,2,2,2,2,2,2,2,2,2,2,2,2,2,2,2,2,2,2,2,2,2,2,2,2,2,
2,2,2,2,2,2,2,2,2,2,2,2,2,2,2,2,2,2,2,2,2,2,2,4),(-2.98894236366457,-2.98719149497955,
-2.98443472872881,-2.97928353659024,-2.96996586450606,-2.91021203323611,
-2.87979806344222,-2.87289157639098,-2.86967129382463,-2.8674133773373,
-2.86450990169052,-2.8593426609542,-2.82575399741682,-2.7992377903783,-2.77576224811274,
-2.76512756988451,-2.75644886827549,-2.75141979058993,-2.74697944090185,
-2.74137767630826,-2.73244029328463,-2.67797095581945,-2.64094100389821,
-2.63532294805655,-2.63235510916507,-2.62985468633074,-2.62663528583978,
-2.61980101151154,-2.58650162489828,-2.55805194956485,-2.53721659057297,
-2.522857418972,-2.51676780410154,-2.51226328374442,-2.50804960782287,-2.50101700566144,
-2.48133850377286,-2.42880805142329,-2.41133405691687,-2.40069840458855,
-2.39689187828238,-2.3943111619637,-2.39159610067171,-2.38715737684294,
-2.37212450614887,-2.32644037719591,-2.29713038581901,-2.28499762108514,
-2.27928669817212,-2.27483468300157,-2.26987000698712,-2.26149663538401,
-2.21998530978775,-2.19016840541577,-2.1738674119672,-2.1637240432157,-2.15998428942998,
-2.15741636088112,-2.15467964946188,-2.15014177579511,-2.13401942462286,
-2.0889146535275,-2.06533955199009,-2.05467593333234,-2.04597869801342,
-2.04094541600944,-2.03650520492702,-2.03090878091542,-2.01939841783481,
-1.96293407093485,-1.93249298140593,-1.92558314687327,-1.92236193561823,
-1.92010361250951,-1.91719995817811,-1.91203316117005,-1.87858219865173,
-1.85183610129742,-1.82840647336711,-1.82633887734828),.UNSPECIFIED.);
#1097=B_SPLINE_CURVE_WITH_KNOTS('',3,(#82037,#82038,#82039,#82040,#82041,
#82042,#82043,#82044,#82045,#82046,#82047,#82048,#82049,#82050,#82051,#82052,
#82053,#82054,#82055,#82056,#82057,#82058,#82059,#82060,#82061,#82062,#82063,
#82064,#82065,#82066,#82067,#82068,#82069,#82070,#82071,#82072,#82073,#82074,
#82075,#82076,#82077,#82078,#82079,#82080,#82081,#82082,#82083,#82084,#82085,
#82086,#82087,#82088,#82089,#82090,#82091,#82092,#82093,#82094,#82095,#82096,
#82097,#82098,#82099,#82100,#82101,#82102,#82103,#82104,#82105,#82106,#82107,
#82108,#82109,#82110,#82111,#82112,#82113,#82114,#82115,#82116,#82117,#82118,
#82119,#82120,#82121,#82122,#82123,#82124,#82125,#82126,#82127,#82128,#82129,
#82130,#82131,#82132,#82133,#82134,#82135,#82136,#82137,#82138,#82139,#82140,
#82141,#82142,#82143,#82144,#82145,#82146,#82147,#82148,#82149,#82150,#82151,
#82152,#82153,#82154,#82155,#82156,#82157,#82158,#82159,#82160,#82161,#82162,
#82163,#82164,#82165,#82166,#82167,#82168,#82169,#82170,#82171,#82172,#82173,
#82174,#82175,#82176,#82177,#82178,#82179,#82180,#82181,#82182,#82183,#82184,
#82185,#82186,#82187,#82188,#82189,#82190,#82191,#82192),.UNSPECIFIED.,
 .F.,.F.,(4,2,2,2,2,2,2,2,2,2,2,2,2,2,2,2,2,2,2,2,2,2,2,2,2,2,2,2,2,2,2,
2,2,2,2,2,2,2,2,2,2,2,2,2,2,2,2,2,2,2,2,2,2,2,2,2,2,2,2,2,2,2,2,2,2,2,2,
2,2,2,2,2,2,2,2,2,2,4),(-1.16376602945442,-1.16069183205709,-1.15788286783102,
-1.15534608126095,-1.15178827005644,-1.14289274022277,-1.12937902479356,
-1.07160488054321,-1.05111372195162,-1.04399028483296,-1.03928943753722,
-1.03473338399442,-1.02834798046327,-1.01204166188582,-0.986976188406588,
-0.931462349770898,-0.924907314360272,-0.921752336311438,-0.919257683878152,
-0.916191330562035,-0.910092298094168,-0.872713837837185,-0.819644568669884,
-0.810580671528279,-0.804940403647636,-0.800494115179469,-0.795484189056702,
-0.78690454654695,-0.738174578636503,-0.694706752770642,-0.688052232068289,
-0.684877863401551,-0.682382267047372,-0.679332385297111,-0.673315895924059,
-0.665340757268196,-0.645052723320984,-0.597600621152522,-0.577284300091211,
-0.570178639171276,-0.565480807648226,-0.560921155593607,-0.554519718165925,
-0.538106663783663,-0.512796923779453,-0.457844888627675,-0.451173484115442,
-0.447996040263678,-0.445500401990743,-0.442453399209398,-0.436451416613632,
-0.428501483072402,-0.408316308829892,-0.361227182980276,-0.340485179414432,
-0.333334250511204,-0.328626938157609,-0.324073265515375,-0.317705627872007,
-0.301529337907284,-0.276763475956864,-0.224150018076021,-0.215441685501549,
-0.211811169687327,-0.209261854479781,-0.206655163671707,-0.202527887014327,
-0.197317962810966,-0.18669839331063,-0.153474588505777,-0.109606078461187,
-0.100196887992094,-0.0944569491039428,-0.0899996154102394,-0.0850466495916382,
-0.0767360479998006,-0.0347791378764354,-0.000700874915968101),
 .UNSPECIFIED.);
#1098=B_SPLINE_CURVE_WITH_KNOTS('',3,(#82193,#82194,#82195,#82196,#82197,
#82198,#82199,#82200,#82201,#82202,#82203,#82204,#82205,#82206,#82207,#82208,
#82209,#82210,#82211,#82212,#82213,#82214,#82215,#82216,#82217,#82218,#82219,
#82220,#82221,#82222,#82223,#82224,#82225,#82226,#82227,#82228,#82229,#82230,
#82231,#82232,#82233,#82234,#82235,#82236,#82237,#82238,#82239,#82240,#82241,
#82242,#82243,#82244),.UNSPECIFIED.,.F.,.F.,(4,2,2,2,2,2,2,2,2,2,2,2,2,
2,2,2,2,2,2,2,2,2,2,2,2,4),(-2.9893126115947,-2.97005979873191,-2.96636877391737,
-2.96374759619947,-2.96141745538025,-2.95908107747098,-2.95521289072605,
-2.94493468189805,-2.92042789239686,-2.86975750041926,-2.85356624816674,
-2.84719691549601,-2.84264325775646,-2.83793701408568,-2.83078981462581,
-2.81008153844967,-2.76293463701884,-2.74272978446433,-2.73477523313501,
-2.72877119265797,-2.72572393422581,-2.72322851526505,-2.72005190500433,
-2.71338406009976,-2.67023979413528,-2.65823196508423),.UNSPECIFIED.);
#1099=B_SPLINE_CURVE_WITH_KNOTS('',3,(#82245,#82246,#82247,#82248,#82249,
#82250,#82251,#82252,#82253,#82254,#82255,#82256,#82257,#82258,#82259,#82260,
#82261,#82262,#82263,#82264,#82265,#82266,#82267,#82268,#82269,#82270,#82271,
#82272,#82273,#82274,#82275,#82276,#82277,#82278,#82279,#82280,#82281,#82282,
#82283,#82284,#82285,#82286,#82287,#82288,#82289,#82290,#82291,#82292,#82293,
#82294,#82295,#82296,#82297,#82298,#82299,#82300,#82301,#82302,#82303,#82304,
#82305,#82306,#82307,#82308,#82309,#82310,#82311,#82312,#82313,#82314,#82315,
#82316,#82317,#82318,#82319,#82320,#82321,#82322,#82323,#82324,#82325,#82326,
#82327,#82328,#82329,#82330,#82331,#82332,#82333,#82334,#82335,#82336,#82337,
#82338,#82339,#82340,#82341,#82342,#82343,#82344,#82345,#82346,#82347,#82348,
#82349,#82350,#82351,#82352,#82353,#82354,#82355,#82356,#82357,#82358,#82359,
#82360,#82361,#82362,#82363,#82364,#82365,#82366,#82367,#82368,#82369,#82370,
#82371,#82372,#82373,#82374,#82375,#82376,#82377,#82378,#82379,#82380,#82381,
#82382,#82383,#82384,#82385,#82386,#82387,#82388,#82389,#82390,#82391,#82392,
#82393,#82394,#82395,#82396,#82397,#82398,#82399,#82400,#82401,#82402,#82403,
#82404,#82405,#82406,#82407,#82408,#82409,#82410,#82411,#82412,#82413,#82414,
#82415,#82416,#82417,#82418,#82419,#82420,#82421,#82422,#82423,#82424,#82425,
#82426,#82427,#82428,#82429,#82430,#82431,#82432,#82433,#82434,#82435,#82436),
 .UNSPECIFIED.,.F.,.F.,(4,2,2,2,2,2,2,2,2,2,2,2,2,2,2,2,2,2,2,2,2,2,2,2,
2,2,2,2,2,2,2,2,2,2,2,2,2,2,2,2,2,2,2,2,2,2,2,2,2,2,2,2,2,2,2,2,2,2,2,2,
2,2,2,2,2,2,2,2,2,2,2,2,2,2,2,2,2,2,2,2,2,2,2,2,2,2,2,2,2,2,2,2,2,2,2,4),
(-1.82633887734828,-1.81778438982932,-1.80911337743571,-1.80408541932622,
-1.79964408722359,-1.79403843363767,-1.78247992116622,-1.72606559545518,
-1.69563933742603,-1.68873073421178,-1.68550961687525,-1.6832511741358,
-1.68034710540596,-1.67517899349204,-1.64161586580808,-1.63875966479735,
-1.61414104677741,-1.59122616610754,-1.58075296432143,-1.5721765304958,
-1.56716836970222,-1.56272361565377,-1.55708530700346,-1.5480246417816,
-1.49487570158239,-1.45878925147032,-1.45187245394213,-1.44864969526387,
-1.44615251690247,-1.4431449137955,-1.43733506746339,-1.42971516231225,
-1.41084110585146,-1.34576832318268,-1.33703781485929,-1.33149601454951,
-1.32706006941872,-1.32198941293647,-1.31311650352168,-1.26540547197718,
-1.22134970219043,-1.21475849771345,-1.21159693789433,-1.20910270947118,
-1.20604390169432,-1.19997966466723,-1.16400355881563,-1.10918103807951,
-1.10027672432412,-1.09468401753295,-1.09024375636261,-1.08520721585225,
-1.07649610651083,-1.02998165767351,-0.984299111980955,-0.977796403120067,
-0.974651757277269,-0.972157961488794,-0.96908373430611,-0.962941999958468,
-0.921310530522911,-0.873028955391398,-0.863714270511721,-0.85800266421684,
-0.853550189728759,-0.84858507725612,-0.840211156485884,-0.795393860740249,
-0.746991056580356,-0.740741741693939,-0.737646220303662,-0.735152642582859,
-0.732030147604351,-0.725642726513586,-0.700044265587319,-0.635016468947442,
-0.626276268734541,-0.62073157684054,-0.616295340693097,-0.611226544975979,
-0.602362709434634,-0.554908348522705,-0.510543429062609,-0.503975026865087,
-0.500817793190879,-0.498323688466495,-0.495260989210625,-0.489177160976494,
-0.453157721312071,-0.398425869330592,-0.389512560884695,-0.38391725076205,
-0.37947678512828,-0.374442000829828,-0.365739087200185,-0.332021502204684),
 .UNSPECIFIED.);
#1100=B_SPLINE_CURVE_WITH_KNOTS('',3,(#82441,#82442,#82443,#82444,#82445,
#82446,#82447,#82448,#82449,#82450,#82451,#82452,#82453,#82454,#82455,#82456,
#82457,#82458,#82459,#82460,#82461,#82462,#82463,#82464,#82465,#82466,#82467,
#82468,#82469,#82470,#82471,#82472,#82473,#82474,#82475,#82476,#82477,#82478,
#82479,#82480,#82481,#82482,#82483,#82484,#82485,#82486,#82487,#82488,#82489,
#82490,#82491,#82492,#82493,#82494,#82495,#82496,#82497,#82498,#82499,#82500,
#82501,#82502,#82503,#82504,#82505,#82506,#82507,#82508,#82509,#82510,#82511,
#82512,#82513,#82514,#82515,#82516,#82517,#82518,#82519,#82520,#82521,#82522,
#82523,#82524,#82525,#82526,#82527,#82528,#82529,#82530,#82531,#82532,#82533,
#82534,#82535,#82536,#82537,#82538,#82539,#82540,#82541,#82542,#82543,#82544,
#82545,#82546,#82547,#82548,#82549,#82550,#82551,#82552,#82553,#82554,#82555,
#82556,#82557,#82558,#82559,#82560,#82561,#82562,#82563,#82564,#82565,#82566,
#82567,#82568,#82569,#82570,#82571,#82572,#82573,#82574,#82575,#82576,#82577,
#82578,#82579,#82580,#82581,#82582,#82583,#82584,#82585,#82586,#82587,#82588,
#82589,#82590,#82591,#82592,#82593,#82594,#82595,#82596,#82597,#82598,#82599,
#82600,#82601,#82602,#82603,#82604,#82605,#82606,#82607,#82608,#82609,#82610,
#82611,#82612,#82613,#82614,#82615,#82616,#82617,#82618,#82619,#82620,#82621,
#82622,#82623,#82624,#82625,#82626,#82627,#82628,#82629,#82630,#82631,#82632,
#82633,#82634,#82635,#82636,#82637,#82638),.UNSPECIFIED.,.F.,.F.,(4,2,2,
2,2,2,2,2,2,2,2,2,2,2,2,2,2,2,2,2,2,2,2,2,2,2,2,2,2,2,2,2,2,2,2,2,2,2,2,
2,2,2,2,2,2,2,2,2,2,2,2,2,2,2,2,2,2,2,2,2,2,2,2,2,2,2,2,2,2,2,2,2,2,2,2,
2,2,2,2,2,2,2,2,2,2,2,2,2,2,2,2,2,2,2,2,2,2,2,4),(-2.65783630003039,-2.62025724672317,
-2.59026002352647,-2.58338687452484,-2.58016987293391,-2.5779147849277,
-2.57502409443245,-2.56987023535567,-2.53601410385819,-2.53220384264842,
-2.49351727602241,-2.47229634900656,-2.46532441422057,-2.46067808289738,
-2.45619347261433,-2.44981793026436,-2.43447698099005,-2.37014745084294,
-2.35617882808727,-2.34708317286216,-2.34351202890345,-2.34098411339723,
-2.33819456913727,-2.33342023946376,-2.31439865527741,-2.27656576230403,
-2.25046201662442,-2.2336953270014,-2.22723427987696,-2.22265502762685,
-2.21850597538671,-2.21188319660244,-2.1952193536177,-2.13968639896198,
-2.12187022712013,-2.11108962809155,-2.10725338800942,-2.10465873617751,
-2.10194101691624,-2.09750404117048,-2.08253386131033,-2.03682544207648,
-2.00077115297086,-1.99267221472486,-1.98776352547717,-1.9832940128199,
-1.9775615295873,-1.96497607002037,-1.90962833227616,-1.87953157722104,
-1.87265534989017,-1.86944013225431,-1.86718284167032,-1.8642768303556,
-1.85909501772978,-1.82448791316893,-1.82281279576623,-1.79437275401685,
-1.77368709296597,-1.75940217335275,-1.75332653976141,-1.74882637293204,
-1.74461255893049,-1.73756980486417,-1.71778446752739,-1.65914474589488,
-1.64556051353102,-1.6366337722647,-1.63307296305554,-1.63053680646219,
-1.62772995463092,-1.6228752428456,-1.60267263019481,-1.5595181903213,-1.52774610497277,
-1.51916513964252,-1.51415363199657,-1.50970538931478,-1.50406182407289,
-1.4949905037558,-1.45921070096346,-1.42149493248338,-1.40234472336841,
-1.3975609912891,-1.39476861893207,-1.39222334445913,-1.38861959501525,
-1.37942803110678,-1.36527856082562,-1.29750524316419,-1.28502018875945,
-1.27922076477125,-1.27474336494521,-1.26987046074447,-1.26193349746236,
-1.22909285958213,-1.18598859412965,-1.16555856101527,-1.16376602945442),
 .UNSPECIFIED.);
#1101=B_SPLINE_CURVE_WITH_KNOTS('',3,(#82640,#82641,#82642,#82643,#82644,
#82645,#82646,#82647,#82648,#82649,#82650,#82651,#82652,#82653,#82654,#82655,
#82656,#82657,#82658,#82659,#82660,#82661,#82662,#82663,#82664,#82665,#82666,
#82667,#82668,#82669,#82670,#82671,#82672,#82673,#82674,#82675,#82676,#82677,
#82678,#82679,#82680,#82681,#82682,#82683,#82684,#82685,#82686,#82687,#82688,
#82689),.UNSPECIFIED.,.F.,.F.,(4,2,2,2,2,2,2,2,2,2,2,2,2,2,2,2,2,2,2,2,
2,2,2,2,4),(-0.332021502204684,-0.314750276325415,-0.273945377692634,-0.267828768211411,
-0.264722750239849,-0.262188964339053,-0.259442466591306,-0.254860805888606,
-0.236311830470826,-0.201955244629108,-0.158843121856831,-0.150476168811389,
-0.145512529941376,-0.14105972825867,-0.135345410942993,-0.12319611792551,
-0.05728481023809,-0.0357895690043997,-0.0298688139829515,-0.0268006421772528,
-0.0245072135341658,-0.0221157627278488,-0.0190823675188528,-0.0121964569415065,
-0.000855159943180343),.UNSPECIFIED.);
#1102=B_SPLINE_CURVE_WITH_KNOTS('',3,(#82690,#82691,#82692,#82693,#82694,
#82695,#82696,#82697,#82698,#82699,#82700,#82701,#82702,#82703,#82704,#82705,
#82706,#82707,#82708,#82709,#82710,#82711,#82712,#82713,#82714,#82715,#82716,
#82717,#82718,#82719,#82720,#82721,#82722,#82723,#82724,#82725,#82726,#82727,
#82728,#82729,#82730,#82731,#82732,#82733,#82734,#82735,#82736,#82737,#82738,
#82739,#82740,#82741,#82742,#82743,#82744,#82745,#82746,#82747,#82748,#82749,
#82750,#82751,#82752,#82753,#82754,#82755,#82756,#82757,#82758,#82759,#82760,
#82761,#82762,#82763,#82764,#82765,#82766,#82767,#82768,#82769,#82770,#82771,
#82772,#82773,#82774,#82775,#82776,#82777,#82778,#82779,#82780,#82781,#82782,
#82783,#82784,#82785,#82786,#82787,#82788,#82789,#82790,#82791,#82792,#82793,
#82794,#82795,#82796,#82797,#82798,#82799,#82800,#82801,#82802,#82803,#82804,
#82805,#82806,#82807,#82808,#82809,#82810,#82811,#82812,#82813,#82814,#82815,
#82816,#82817,#82818,#82819,#82820,#82821,#82822,#82823,#82824,#82825,#82826,
#82827,#82828,#82829,#82830,#82831,#82832,#82833,#82834,#82835,#82836,#82837,
#82838,#82839,#82840,#82841,#82842,#82843,#82844,#82845,#82846,#82847,#82848,
#82849,#82850,#82851),.UNSPECIFIED.,.F.,.F.,(4,2,2,2,2,2,2,2,2,2,2,2,2,
2,2,2,2,2,2,2,2,2,2,2,2,2,2,2,2,2,2,2,2,2,2,2,2,2,2,2,2,2,2,2,2,2,2,2,2,
2,2,2,2,2,2,2,2,2,2,2,2,2,2,2,2,2,2,2,2,2,2,2,2,2,2,2,2,2,2,2,4),(1.16366148960649,
1.16368973496222,1.16649156184632,1.16902779165957,1.17259386188237,1.18155821463464,
1.19522459278802,1.25504508512148,1.27376199386646,1.28066823112477,1.28485582794688,
1.28936993467832,1.29553965423417,1.31043035232553,1.33237825308395,1.37553549347217,
1.39574582192838,1.4005868449715,1.4033878162072,1.40592494672093,1.4094909219926,
1.41844118160067,1.4320738560481,1.49139262735065,1.51053614798074,1.51750495550926,
1.52170799288443,1.52622192218291,1.53236145229041,1.54702780299661,1.56850079790653,
1.61077965475065,1.63238866505133,1.6373149755014,1.64013737238837,1.64266977575962,
1.64619984252791,1.65491927423381,1.66806293992059,1.72134718560026,1.74593068914121,
1.75354531019233,1.75834813960603,1.76284784104249,1.76890878188728,1.78309104304976,
1.80356421713465,1.83230168321304,1.83454973361319,1.86865084058222,1.87382418604824,
1.87672887053467,1.87898624884471,1.88220381332518,1.88909702423443,1.91938336237638,
1.97536231073971,1.98611570852936,1.99161727673111,1.99615375622198,2.00080384543155,
2.00768701961816,2.02787095104097,2.06315115545376,2.10291576507191,2.10972923896683,
2.11293185190813,2.11529397402805,2.11821543299602,2.12325668911744,2.12992878450712,
2.14529984158548,2.17611547722575,2.21808329528982,2.22645135701701,2.23141448867634,
2.23586611452627,2.24157793785585,2.25371829376451,2.31956693196985,2.32642657710849),
 .UNSPECIFIED.);
#1103=B_SPLINE_CURVE_WITH_KNOTS('',3,(#82855,#82856,#82857,#82858,#82859,
#82860),.UNSPECIFIED.,.F.,.F.,(4,1,1,4),(-4.09293042013066,-3.98462531944883,
-2.98846898958662,-2.06883560534994),.UNSPECIFIED.);
#1104=B_SPLINE_CURVE_WITH_KNOTS('',3,(#82864,#82865,#82866,#82867,#82868),
 .UNSPECIFIED.,.F.,.F.,(4,1,4),(0.,0.996156329862203,1.11730040836818),
 .UNSPECIFIED.);
#1105=B_SPLINE_CURVE_WITH_KNOTS('',3,(#82870,#82871,#82872,#82873,#82874,
#82875,#82876,#82877,#82878,#82879,#82880,#82881,#82882,#82883,#82884,#82885,
#82886,#82887,#82888,#82889,#82890,#82891,#82892,#82893,#82894,#82895,#82896,
#82897,#82898,#82899,#82900,#82901,#82902,#82903,#82904,#82905,#82906,#82907,
#82908,#82909,#82910,#82911,#82912,#82913,#82914,#82915,#82916,#82917,#82918,
#82919,#82920,#82921,#82922,#82923,#82924,#82925,#82926,#82927,#82928,#82929,
#82930,#82931,#82932,#82933,#82934,#82935,#82936,#82937,#82938,#82939,#82940,
#82941,#82942,#82943,#82944,#82945,#82946,#82947,#82948,#82949,#82950,#82951,
#82952,#82953,#82954,#82955,#82956,#82957,#82958,#82959,#82960,#82961,#82962,
#82963,#82964,#82965,#82966,#82967,#82968,#82969,#82970,#82971,#82972,#82973,
#82974,#82975,#82976,#82977,#82978,#82979,#82980,#82981,#82982,#82983,#82984,
#82985,#82986,#82987),.UNSPECIFIED.,.F.,.F.,(4,3,3,3,3,3,3,3,3,3,3,3,3,
3,3,3,3,3,3,3,3,3,3,3,3,3,3,3,3,3,3,3,3,3,3,3,3,3,3,4),(1.11730040836818,
1.28262178372048,1.44765157556473,1.61268575152221,1.77772714966095,1.94312500432988,
1.99231265972441,2.16189896620006,2.33115735598945,2.50038270972217,2.66956176012431,
2.83913553552575,2.98846898958662,3.15809751684031,3.32740711791633,3.49669689813223,
3.66594774295676,3.83560425255262,3.98462531944882,4.15373065172872,4.32250351684065,
4.49124368676202,4.65993689797336,4.82903410602685,4.98078164931103,5.15016484644186,
5.31922045795961,5.48824672073902,5.6572283792484,5.82661190548429,5.97693797917324,
6.14630615262454,6.31534759373514,6.48436122853589,6.6533310844071,6.82270445493501,
6.97309430903544,7.15761149677957,7.34097651449696,7.40048571521261),
 .UNSPECIFIED.);
#1106=B_SPLINE_CURVE_WITH_KNOTS('',3,(#82989,#82990,#82991,#82992,#82993,
#82994,#82995,#82996,#82997,#82998,#82999,#83000,#83001,#83002,#83003,#83004,
#83005,#83006,#83007,#83008,#83009,#83010,#83011,#83012,#83013,#83014,#83015,
#83016,#83017,#83018,#83019,#83020,#83021,#83022,#83023,#83024,#83025,#83026,
#83027,#83028,#83029,#83030,#83031,#83032,#83033,#83034,#83035,#83036,#83037,
#83038,#83039,#83040,#83041,#83042,#83043,#83044,#83045,#83046,#83047,#83048,
#83049,#83050,#83051,#83052,#83053,#83054,#83055,#83056,#83057,#83058,#83059,
#83060,#83061,#83062,#83063,#83064,#83065,#83066,#83067,#83068,#83069,#83070,
#83071,#83072,#83073,#83074,#83075,#83076,#83077,#83078,#83079,#83080,#83081,
#83082,#83083,#83084,#83085,#83086,#83087,#83088,#83089,#83090,#83091,#83092,
#83093,#83094,#83095,#83096,#83097,#83098,#83099,#83100,#83101,#83102,#83103,
#83104,#83105,#83106),.UNSPECIFIED.,.F.,.F.,(4,3,3,3,3,3,3,3,3,3,3,3,3,
3,3,3,3,3,3,3,3,3,3,3,3,3,3,3,3,3,3,3,3,3,3,3,3,3,3,4),(7.40048571554775,
7.57307735536024,7.74582609884619,7.91907496157944,7.96925063889765,8.13859372637515,
8.30760905245861,8.47659536915156,8.64553719871405,8.81488194247415,8.96540696875986,
9.13474435570046,9.30375402266731,9.47273483050185,9.64167122408181,9.81101077077705,
9.96156329862207,10.1308922600792,10.299893255479,10.4688651405637,10.6377924578226,
10.8071228616149,10.9577196284843,11.127054944352,11.2960624227752,11.465040892599,
11.6339748619994,11.8033118903903,11.9538759583465,12.1232099666738,12.2922161317669,
12.461193299171,12.6301259698601,12.7994617334433,12.9500322882087,13.1176514663611,
13.2849613103928,13.4520936828031,13.6193212956903,13.6836710227273),
 .UNSPECIFIED.);
#1107=B_SPLINE_CURVE_WITH_KNOTS('',3,(#83108,#83109,#83110,#83111,#83112,
#83113,#83114,#83115,#83116,#83117,#83118,#83119,#83120,#83121,#83122,#83123,
#83124,#83125,#83126,#83127,#83128,#83129,#83130,#83131,#83132,#83133,#83134,
#83135,#83136,#83137,#83138,#83139,#83140,#83141,#83142,#83143,#83144,#83145,
#83146,#83147,#83148,#83149,#83150,#83151,#83152,#83153,#83154,#83155,#83156,
#83157,#83158,#83159,#83160,#83161,#83162,#83163,#83164,#83165,#83166,#83167,
#83168,#83169,#83170,#83171,#83172,#83173,#83174,#83175,#83176,#83177,#83178,
#83179,#83180,#83181,#83182,#83183,#83184,#83185,#83186,#83187,#83188,#83189,
#83190,#83191,#83192,#83193,#83194,#83195,#83196,#83197,#83198,#83199,#83200,
#83201,#83202,#83203,#83204,#83205,#83206,#83207,#83208,#83209,#83210,#83211,
#83212,#83213,#83214,#83215,#83216,#83217,#83218,#83219,#83220,#83221,#83222,
#83223,#83224,#83225),.UNSPECIFIED.,.F.,.F.,(4,3,3,3,3,3,3,3,3,3,3,3,3,
3,3,3,3,3,3,3,3,3,3,3,3,3,3,3,3,3,3,3,3,3,3,3,3,3,3,4),(13.6836710228995,
13.8982811297081,13.9461886180709,14.1155225548806,14.2845286362706,14.4535057022928,
14.6224382617149,14.7917738996828,14.9423449479331,15.1116786313851,15.2806844569256,
15.4496612671025,15.6185935702331,15.7879289566079,15.9385012777953,16.1078348519791,
16.2768405642568,16.445817256677,16.6147494393768,16.7840847033611,16.9346576076575,
17.1039913134022,17.272997160196,17.4419739896877,17.6109063111027,17.7802417136301,
17.9308139375197,18.1001475983451,18.2691533996324,18.4381301833948,18.6070624588776,
18.7763978161076,18.9269702673819,19.0963039177279,19.2653097080604,19.4342864802948,
19.6032187439149,19.7725540889681,19.9231265972441,19.9668563299069),
 .UNSPECIFIED.);
#1108=B_SPLINE_CURVE_WITH_KNOTS('',3,(#83227,#83228,#83229,#83230,#83231,
#83232,#83233,#83234,#83235,#83236,#83237,#83238,#83239,#83240,#83241,#83242,
#83243,#83244,#83245,#83246,#83247,#83248,#83249,#83250,#83251,#83252,#83253,
#83254,#83255,#83256,#83257,#83258,#83259,#83260,#83261,#83262,#83263,#83264,
#83265,#83266,#83267,#83268,#83269,#83270,#83271,#83272,#83273,#83274,#83275,
#83276,#83277,#83278,#83279,#83280,#83281,#83282,#83283,#83284,#83285,#83286,
#83287,#83288,#83289,#83290,#83291,#83292,#83293,#83294,#83295,#83296,#83297,
#83298,#83299,#83300,#83301,#83302,#83303,#83304,#83305,#83306,#83307,#83308,
#83309,#83310,#83311,#83312,#83313,#83314,#83315,#83316,#83317,#83318,#83319,
#83320,#83321,#83322,#83323,#83324,#83325,#83326,#83327,#83328,#83329,#83330,
#83331,#83332,#83333,#83334,#83335,#83336,#83337,#83338,#83339,#83340,#83341),
 .UNSPECIFIED.,.F.,.F.,(4,3,3,3,3,3,3,3,3,3,3,3,3,3,3,3,3,3,3,3,3,3,3,3,
3,3,3,3,3,3,3,3,3,3,3,3,3,3,4),(19.966856330194,20.135016386822,20.3028589202274,
20.4706807137549,20.6384750732032,20.8066513695237,20.9192829271063,21.0886165881965,
21.2576223895894,21.4265991732081,21.5955314484101,21.7648668051334,21.9154392569686,
22.0847729173349,22.2537787179511,22.4227555007232,22.5916877750386,22.7610231308267,
22.9115955868308,23.080929249669,23.2499350528188,23.4189118381815,23.5878441151235,
23.7571794735431,23.907751916693,24.0770855783232,24.2460913802444,24.415068164365,
24.5840004400555,24.7533357972341,24.9039082465552,25.0732419081956,25.2422477101218,
25.4112244942395,25.5801567699226,25.7494921270864,25.9000645764174,26.0945925740695,
26.2500413990553),.UNSPECIFIED.);
#1109=B_SPLINE_CURVE_WITH_KNOTS('',3,(#83343,#83344,#83345,#83346,#83347,
#83348,#83349,#83350,#83351,#83352),.UNSPECIFIED.,.F.,.F.,(4,1,1,1,1,1,
1,4),(26.2500416370865,26.8962209062796,27.8923772361418,28.888533566004,
29.8846898958662,30.8808462257284,31.8770025555906,32.5332269442661),
 .UNSPECIFIED.);
#1110=B_SPLINE_CURVE_WITH_KNOTS('',3,(#83354,#83355,#83356,#83357,#83358,
#83359,#83360,#83361,#83362,#83363),.UNSPECIFIED.,.F.,.F.,(4,1,1,1,1,1,
1,4),(32.5332269442661,32.8731588854528,33.869315215315,34.8654715451772,
35.8616278750394,36.8577842049016,37.8539405347639,38.8164122514457),
 .UNSPECIFIED.);
#1111=B_SPLINE_CURVE_WITH_KNOTS('',3,(#83365,#83366,#83367,#83368,#83369,
#83370,#83371,#83372,#83373,#83374,#83375),.UNSPECIFIED.,.F.,.F.,(4,1,1,
1,1,1,1,1,4),(38.8164122514457,38.8500968646261,39.8462531944883,40.8424095243505,
41.8385658542127,42.8347221840749,43.8308785139371,44.8270348437993,45.0995938882313),
 .UNSPECIFIED.);
#1112=B_SPLINE_CURVE_WITH_KNOTS('',3,(#83377,#83378,#83379,#83380,#83381,
#83382,#83383,#83384,#83385,#83386,#83387,#83388,#83389,#83390,#83391,#83392,
#83393,#83394,#83395,#83396,#83397,#83398,#83399,#83400,#83401,#83402,#83403,
#83404,#83405,#83406,#83407,#83408,#83409,#83410,#83411,#83412,#83413,#83414,
#83415,#83416,#83417,#83418,#83419,#83420,#83421,#83422,#83423,#83424,#83425,
#83426,#83427,#83428,#83429,#83430,#83431,#83432,#83433,#83434,#83435,#83436,
#83437,#83438,#83439,#83440,#83441,#83442,#83443,#83444,#83445,#83446,#83447,
#83448,#83449,#83450,#83451,#83452,#83453,#83454,#83455,#83456,#83457,#83458,
#83459,#83460,#83461,#83462,#83463,#83464,#83465,#83466,#83467,#83468,#83469,
#83470,#83471,#83472,#83473,#83474,#83475,#83476,#83477,#83478,#83479,#83480,
#83481,#83482,#83483,#83484,#83485,#83486,#83487,#83488,#83489,#83490,#83491,
#83492,#83493,#83494),.UNSPECIFIED.,.F.,.F.,(4,3,3,3,3,3,3,3,3,3,3,3,3,
3,3,3,3,3,3,3,3,3,3,3,3,3,3,3,3,3,3,3,3,3,3,3,3,3,3,4),(45.0995975586253,
45.2669647013515,45.4343603268434,45.6017766473786,45.7695612509881,45.8231911736615,
45.9925248354768,46.1615306375833,46.330507421887,46.4994396977595,46.6687750551146,
46.8193475035237,46.988681165339,47.1576869674455,47.3266637517491,47.4955960276217,
47.6649313849767,47.8155038333859,47.9848374952012,48.1538432973077,48.3228200816114,
48.4917523574839,48.6610877148389,48.8116601632481,48.9809938250634,49.14999962717,
49.3189764114737,49.4879086873463,49.6572440447014,49.8078164931104,49.9771501549257,
50.1461559570324,50.3151327413361,50.4840650172086,50.6534003745637,50.8039728229726,
50.9766852054187,51.1489995200855,51.3210324932485,51.3827828658049),
 .UNSPECIFIED.);
#1113=B_SPLINE_CURVE_WITH_KNOTS('',3,(#83496,#83497,#83498,#83499,#83500,
#83501,#83502,#83503,#83504,#83505,#83506,#83507,#83508,#83509,#83510,#83511,
#83512,#83513,#83514,#83515,#83516,#83517,#83518,#83519,#83520,#83521,#83522,
#83523,#83524,#83525,#83526,#83527,#83528,#83529,#83530,#83531,#83532,#83533,
#83534,#83535,#83536,#83537,#83538,#83539,#83540,#83541,#83542,#83543,#83544,
#83545,#83546,#83547,#83548,#83549,#83550,#83551,#83552,#83553,#83554,#83555,
#83556,#83557,#83558,#83559,#83560,#83561,#83562,#83563,#83564,#83565,#83566,
#83567,#83568,#83569,#83570,#83571,#83572,#83573,#83574,#83575,#83576,#83577,
#83578,#83579,#83580,#83581,#83582,#83583,#83584,#83585,#83586,#83587,#83588,
#83589,#83590,#83591,#83592,#83593,#83594,#83595,#83596,#83597,#83598,#83599,
#83600,#83601,#83602,#83603,#83604,#83605,#83606,#83607,#83608,#83609,#83610,
#83611,#83612,#83613),.UNSPECIFIED.,.F.,.F.,(4,3,3,3,3,3,3,3,3,3,3,3,3,
3,3,3,3,3,3,3,3,3,3,3,3,3,3,3,3,3,3,3,3,3,3,3,3,3,3,4),(51.3827828659881,
51.5671902339565,51.7528607040205,51.8001291528347,51.9694628146501,52.1384686167567,
52.3074454010605,52.4763776769332,52.6457130342883,52.796285482697,52.9656191445123,
53.1346249466188,53.3036017309224,53.472534006795,53.64186936415,53.7924418125592,
53.9617754743744,54.1307812764809,54.2997580607846,54.4686903366571,54.6380256940121,
54.7885981424214,54.9579318042367,55.1269376063432,55.2959143906469,55.4648466665194,
55.6341820238745,55.7847544722836,55.9540881340989,56.1230939362054,56.292070720509,
56.4610029963816,56.6303383537366,56.7809108021458,56.9480120911382,57.1147891675956,
57.281513061229,57.4482111102018,57.6152110190328,57.665968172762),
 .UNSPECIFIED.);
#1114=B_SPLINE_CURVE_WITH_KNOTS('',3,(#83615,#83616,#83617,#83618,#83619,
#83620,#83621,#83622,#83623,#83624,#83625,#83626,#83627,#83628,#83629,#83630,
#83631,#83632,#83633,#83634,#83635,#83636,#83637,#83638,#83639,#83640,#83641,
#83642,#83643,#83644,#83645,#83646,#83647,#83648,#83649,#83650,#83651,#83652,
#83653,#83654,#83655,#83656,#83657,#83658,#83659,#83660,#83661,#83662,#83663,
#83664,#83665,#83666,#83667,#83668,#83669,#83670,#83671,#83672,#83673,#83674,
#83675,#83676,#83677,#83678,#83679,#83680,#83681,#83682,#83683,#83684,#83685,
#83686,#83687,#83688,#83689,#83690,#83691,#83692,#83693,#83694,#83695,#83696,
#83697,#83698,#83699,#83700,#83701,#83702,#83703,#83704,#83705,#83706,#83707,
#83708,#83709,#83710,#83711,#83712,#83713,#83714,#83715,#83716,#83717,#83718,
#83719,#83720,#83721,#83722,#83723,#83724,#83725,#83726,#83727,#83728,#83729),
 .UNSPECIFIED.,.F.,.F.,(4,3,3,3,3,3,3,3,3,3,3,3,3,3,3,3,3,3,3,3,3,3,3,3,
3,3,3,3,3,3,3,3,3,3,3,3,3,3,4),(57.6659681729845,57.777067132008,57.9464007938234,
58.1154065959299,58.2843833802337,58.4533156561063,58.6226510134614,58.7732234618702,
58.9425571236855,59.1115629257921,59.2805397100958,59.4494719859684,59.6188073433234,
59.7693797917324,59.9387134535477,60.1077192556542,60.2766960399578,60.4456283158303,
60.6149636731854,60.7655361215946,60.9348697834097,61.103875585516,61.2728523698194,
61.4417846456918,61.6111200030466,61.7616924514568,61.9310261132726,62.1000319153795,
62.2690086996837,62.4379409755567,62.6072763329121,62.7578487813191,62.9271824431342,
63.0961882452405,63.265165029544,63.4340973054164,63.6034326627713,63.7540051111813,
63.9491534801641),.UNSPECIFIED.);
#1115=B_SPLINE_CURVE_WITH_KNOTS('',3,(#83731,#83732,#83733,#83734,#83735,
#83736,#83737,#83738,#83739,#83740),.UNSPECIFIED.,.F.,.F.,(4,1,1,1,1,1,
1,4),(63.9491570786823,64.7501614410435,65.7463177709057,66.7424741007679,
67.7386304306301,68.7347867604923,69.7309430903545,70.2323387873437),
 .UNSPECIFIED.);
#1116=B_SPLINE_CURVE_WITH_KNOTS('',3,(#83742,#83743,#83744,#83745,#83746,
#83747,#83748,#83749,#83750,#83751),.UNSPECIFIED.,.F.,.F.,(4,1,1,1,1,1,
1,4),(70.2323387873437,70.7270994202167,71.7232557500789,72.7194120799411,
73.7155684098033,74.7117247396655,75.7078810695277,76.5155240945233),
 .UNSPECIFIED.);
#1117=B_SPLINE_CURVE_WITH_KNOTS('',3,(#83753,#83754,#83755,#83756,#83757,
#83758,#83759,#83760,#83761,#83762,#83763),.UNSPECIFIED.,.F.,.F.,(4,1,1,
1,1,1,1,1,4),(76.5155240945233,76.7040373993899,77.7001937292521,78.6963500591144,
79.6925063889766,80.6886627188388,81.684819048701,82.6809753785631,82.7987094017029),
 .UNSPECIFIED.);
#1118=B_SPLINE_CURVE_WITH_KNOTS('',3,(#83765,#83766,#83767,#83768,#83769,
#83770,#83771,#83772,#83773,#83774,#83775,#83776,#83777,#83778,#83779,#83780,
#83781,#83782,#83783,#83784,#83785,#83786,#83787,#83788,#83789,#83790,#83791,
#83792,#83793,#83794,#83795,#83796,#83797,#83798,#83799,#83800,#83801,#83802,
#83803,#83804,#83805,#83806,#83807,#83808,#83809,#83810,#83811,#83812,#83813,
#83814,#83815,#83816,#83817,#83818,#83819,#83820,#83821,#83822,#83823,#83824,
#83825,#83826,#83827,#83828,#83829,#83830,#83831,#83832,#83833,#83834,#83835,
#83836,#83837,#83838,#83839,#83840,#83841,#83842,#83843,#83844,#83845,#83846,
#83847,#83848,#83849,#83850,#83851,#83852,#83853,#83854,#83855,#83856,#83857,
#83858,#83859,#83860,#83861,#83862,#83863,#83864,#83865,#83866,#83867,#83868,
#83869,#83870,#83871,#83872,#83873,#83874,#83875,#83876,#83877,#83878,#83879,
#83880,#83881,#83882),.UNSPECIFIED.,.F.,.F.,(4,3,3,3,3,3,3,3,3,3,3,3,3,
3,3,3,3,3,3,3,3,3,3,3,3,3,3,3,3,3,3,3,3,3,3,3,3,3,3,4),(82.7987094017029,
82.965636580998,83.1322893848818,83.2989591266341,83.4656459127014,83.632687711285,
83.6771317084254,83.8464646791663,84.0154697909957,84.1844458962506,84.3533774980481,
84.5227122036214,84.6732880382876,84.842622109511,85.0116283124841,85.1806054790275,
85.3495381275839,85.5188738342397,85.6694443681498,85.8387797027031,86.00778719238,
86.176765661948,86.3456996247729,86.5150366362511,86.665600698012,86.8349293911137,
87.00393022489,87.1729021136412,87.3418295253239,87.511160171998,87.6617570278742,
87.8310949042705,88.0001048660142,88.1690856671441,88.3380218884775,88.5073609921549,
88.6579133577364,88.8428584338325,89.0266242915967,89.0818943520482),
 .UNSPECIFIED.);
#1119=B_SPLINE_CURVE_WITH_KNOTS('',3,(#83884,#83885,#83886,#83887,#83888,
#83889,#83890,#83891,#83892,#83893),.UNSPECIFIED.,.F.,.F.,(4,1,1,1,1,1,
1,4),(89.0818947088824,89.6540696875986,90.6502260174608,91.646382347323,
92.6425386771853,93.6386950070475,94.6348513369097,95.365080016062),
 .UNSPECIFIED.);
#1120=B_SPLINE_CURVE_WITH_KNOTS('',3,(#83901,#83902,#83903,#83904,#83905,
#83906,#83907,#83908,#83909),.UNSPECIFIED.,.F.,.F.,(4,1,1,1,1,1,4),(-97.6233203264963,
-96.6271639966341,-95.6310076667719,-94.6348513369097,-93.6386950070475,
-92.6425386771853,-92.0575247206449),.UNSPECIFIED.);
#1121=B_SPLINE_CURVE_WITH_KNOTS('',3,(#83911,#83912,#83913,#83914,#83915,
#83916,#83917,#83918,#83919,#83920,#83921,#83922,#83923,#83924,#83925,#83926,
#83927,#83928,#83929,#83930,#83931,#83932,#83933,#83934,#83935,#83936,#83937,
#83938,#83939,#83940,#83941,#83942,#83943,#83944,#83945,#83946,#83947,#83948,
#83949,#83950,#83951,#83952,#83953,#83954,#83955,#83956,#83957,#83958,#83959,
#83960,#83961,#83962,#83963,#83964,#83965,#83966,#83967,#83968,#83969,#83970,
#83971,#83972,#83973,#83974,#83975,#83976,#83977,#83978,#83979,#83980,#83981,
#83982,#83983,#83984,#83985,#83986,#83987,#83988,#83989,#83990,#83991,#83992,
#83993,#83994,#83995,#83996,#83997,#83998,#83999,#84000,#84001,#84002,#84003,
#84004,#84005,#84006,#84007,#84008,#84009,#84010,#84011,#84012,#84013,#84014,
#84015,#84016,#84017,#84018,#84019,#84020,#84021,#84022,#84023,#84024,#84025,
#84026,#84027,#84028),.UNSPECIFIED.,.F.,.F.,(4,3,3,3,3,3,3,3,3,3,3,3,3,
3,3,3,3,3,3,3,3,3,3,3,3,3,3,3,3,3,3,3,3,3,3,3,3,3,3,4),(-92.0575243311351,
-91.8725281814524,-91.686228476792,-91.6463823473231,-91.4770142027803,
-91.3079727917837,-91.1389591885252,-90.9699893650353,-90.8006160276294,
-90.6502260174609,-90.4809254554687,-90.3119534642138,-90.1430110847365,
-89.9741136005011,-89.8048129492577,-89.6540696875987,-89.4847266274735,
-89.3157113291214,-89.1467250403316,-88.9777832388153,-88.8084385227493,
-88.6579133577364,-88.4885759751671,-88.3195663127972,-88.1505855098421,
-87.9816491213052,-87.8123095798237,-87.6617570278742,-87.4924280547676,
-87.3234270474557,-87.1544551502299,-86.9855278206825,-86.8161974046127,
-86.665600698012,-86.4984322992574,-86.3315880451506,-86.1647945025351,
-85.9980272414912,-85.8309511841658,-85.7743394136888),.UNSPECIFIED.);
#1122=B_SPLINE_CURVE_WITH_KNOTS('',3,(#84030,#84031,#84032,#84033,#84034,
#84035,#84036,#84037,#84038,#84039,#84040,#84041,#84042,#84043,#84044,#84045,
#84046,#84047,#84048,#84049,#84050,#84051,#84052,#84053,#84054,#84055,#84056,
#84057,#84058,#84059,#84060,#84061,#84062,#84063,#84064,#84065,#84066,#84067,
#84068,#84069,#84070,#84071,#84072,#84073,#84074,#84075,#84076,#84077,#84078,
#84079,#84080,#84081,#84082,#84083,#84084,#84085,#84086,#84087,#84088,#84089,
#84090,#84091,#84092,#84093,#84094,#84095,#84096,#84097,#84098,#84099,#84100,
#84101,#84102,#84103,#84104,#84105,#84106,#84107,#84108,#84109,#84110,#84111,
#84112,#84113,#84114,#84115,#84116,#84117,#84118,#84119,#84120,#84121,#84122,
#84123,#84124,#84125,#84126,#84127,#84128,#84129,#84130,#84131,#84132,#84133,
#84134,#84135,#84136,#84137,#84138,#84139,#84140,#84141,#84142,#84143,#84144),
 .UNSPECIFIED.,.F.,.F.,(4,3,3,3,3,3,3,3,3,3,3,3,3,3,3,3,3,3,3,3,3,3,3,3,
3,3,3,3,3,3,3,3,3,3,3,3,3,3,4),(-85.7743394134653,-85.6694443681498,-85.500110360217,
-85.3311041955529,-85.1621270286254,-84.9931943584398,-84.8238585953951,
-84.6732880382876,-84.503955024643,-84.334949886129,-84.1659737793373,-83.9970421898078,
-83.8277075191266,-83.6771317084254,-83.5077977726898,-83.3387916923914,
-83.1698146274717,-83.0008820691601,-82.8315464322925,-82.6809753785632,
-82.5116416950953,-82.3426358695433,-82.173659059362,-82.0047267562309,
-81.8353913698622,-81.684819048701,-81.5154854741947,-81.3464797615862,
-81.1775030688277,-81.0085708857849,-80.8392356214567,-80.6886627188388,
-80.5193290132907,-80.350323166697,-80.1813463374077,-80.0124140161968,
-79.8430786138719,-79.6925063889766,-79.4911541062857),.UNSPECIFIED.);
#1123=B_SPLINE_CURVE_WITH_KNOTS('',3,(#84146,#84147,#84148,#84149,#84150,
#84151,#84152,#84153,#84154,#84155,#84156,#84157,#84158,#84159,#84160,#84161,
#84162,#84163,#84164,#84165,#84166,#84167,#84168,#84169,#84170,#84171,#84172,
#84173,#84174,#84175,#84176,#84177,#84178,#84179,#84180,#84181,#84182,#84183,
#84184,#84185,#84186,#84187,#84188,#84189,#84190,#84191,#84192,#84193,#84194,
#84195,#84196,#84197,#84198,#84199,#84200,#84201,#84202,#84203,#84204,#84205,
#84206,#84207,#84208,#84209,#84210,#84211,#84212,#84213,#84214,#84215,#84216,
#84217,#84218,#84219,#84220,#84221,#84222,#84223,#84224,#84225,#84226,#84227,
#84228,#84229,#84230,#84231,#84232,#84233,#84234,#84235,#84236,#84237,#84238,
#84239,#84240,#84241,#84242,#84243,#84244,#84245,#84246,#84247,#84248,#84249,
#84250,#84251,#84252,#84253,#84254,#84255,#84256,#84257,#84258,#84259,#84260),
 .UNSPECIFIED.,.F.,.F.,(4,3,3,3,3,3,3,3,3,3,3,3,3,3,3,3,3,3,3,3,3,3,3,3,
3,3,3,3,3,3,3,3,3,3,3,3,3,3,4),(-79.4911541059791,-79.3245057004151,-79.1579164140378,
-78.9913821131007,-78.8244722076974,-78.6963500591144,-78.5270164087195,
-78.3580106183368,-78.189033846051,-78.0201015823787,-77.8507662372729,
-77.7001937292522,-77.530860060675,-77.3618542516806,-77.1928774603977,
-77.0239451774834,-76.854609813131,-76.7040373993899,-76.5347037382941,
-76.3656979368956,-76.1967211532715,-76.0277888780641,-75.8584535213355,
-75.7078810695277,-75.5385474091545,-75.369541608531,-75.2005648257516,
-75.0316325514286,-74.862297195633,-74.7117247396655,-74.542391076833,-74.3733852736891,
-74.2044084883325,-74.0354762113964,-73.8661408529829,-73.7155684098033,
-73.5384040357233,-73.3618892358082,-73.2079687991062),.UNSPECIFIED.);
#1124=B_SPLINE_CURVE_WITH_KNOTS('',3,(#84262,#84263,#84264,#84265,#84266,
#84267,#84268,#84269,#84270,#84271),.UNSPECIFIED.,.F.,.F.,(4,1,1,1,1,1,
1,4),(-73.2079680704952,-72.7194120799411,-71.7232557500789,-70.7270994202167,
-69.7309430903545,-68.7347867604923,-67.7386304306301,-66.9247834919266),
 .UNSPECIFIED.);
#1125=B_SPLINE_CURVE_WITH_KNOTS('',3,(#84273,#84274,#84275,#84276,#84277,
#84278,#84279,#84280,#84281,#84282,#84283),.UNSPECIFIED.,.F.,.F.,(4,1,1,
1,1,1,1,1,4),(-66.9247834919266,-66.7424741007679,-65.7463177709057,-64.7501614410435,
-63.7540051111813,-62.757848781319,-61.7616924514569,-60.7655361215946,
-60.641598184747),.UNSPECIFIED.);
#1126=B_SPLINE_CURVE_WITH_KNOTS('',3,(#84285,#84286,#84287,#84288,#84289,
#84290,#84291,#84292,#84293,#84294),.UNSPECIFIED.,.F.,.F.,(4,1,1,1,1,1,
1,4),(-60.641598184747,-59.7693797917324,-58.7732234618702,-57.777067132008,
-56.7809108021458,-55.7847544722836,-54.7885981424214,-54.35841793122),
 .UNSPECIFIED.);
#1127=B_SPLINE_CURVE_WITH_KNOTS('',3,(#84296,#84297,#84298,#84299,#84300,
#84301,#84302,#84303,#84304,#84305,#84306,#84307,#84308,#84309,#84310,#84311,
#84312,#84313,#84314,#84315,#84316,#84317,#84318,#84319,#84320,#84321,#84322,
#84323,#84324,#84325,#84326,#84327,#84328,#84329,#84330,#84331,#84332,#84333,
#84334,#84335,#84336,#84337,#84338,#84339,#84340,#84341,#84342,#84343,#84344,
#84345,#84346,#84347,#84348,#84349,#84350,#84351,#84352,#84353,#84354,#84355,
#84356,#84357,#84358,#84359,#84360,#84361,#84362,#84363,#84364,#84365,#84366,
#84367,#84368,#84369,#84370,#84371,#84372,#84373,#84374,#84375,#84376,#84377,
#84378,#84379,#84380,#84381,#84382,#84383,#84384,#84385,#84386,#84387,#84388,
#84389,#84390,#84391,#84392,#84393,#84394,#84395,#84396,#84397,#84398,#84399,
#84400,#84401,#84402,#84403,#84404,#84405,#84406,#84407,#84408,#84409,#84410,
#84411,#84412,#84413),.UNSPECIFIED.,.F.,.F.,(4,3,3,3,3,3,3,3,3,3,3,3,3,
3,3,3,3,3,3,3,3,3,3,3,3,3,3,3,3,3,3,3,3,3,3,3,3,3,3,4),(-54.3584128775674,
-54.1856448261282,-54.0127120160945,-53.8392756664467,-53.7924418125592,
-53.6231081507439,-53.4541023486374,-53.2851255643338,-53.1161932884612,
-52.9468579311062,-52.796285482697,-52.6269518208817,-52.4579460187752,
-52.2889692344716,-52.120036958599,-51.950701601244,-51.8001291528348,-51.6307954910195,
-51.461789688913,-51.2928129046094,-51.1238806287368,-50.9545452713818,
-50.8039728229726,-50.6346391611574,-50.4656333590508,-50.2966565747472,
-50.1277242988747,-49.9583889415196,-49.8078164931104,-49.6384828312951,
-49.4694770291886,-49.3005002448849,-49.1315679690123,-48.9622326116573,
-48.8116601632482,-48.6440875454568,-48.4768218743308,-48.3097330096438,
-48.1425443209698,-48.0752275703878),.UNSPECIFIED.);
#1128=B_SPLINE_CURVE_WITH_KNOTS('',3,(#84415,#84416,#84417,#84418,#84419,
#84420,#84421,#84422,#84423,#84424,#84425,#84426,#84427,#84428,#84429,#84430,
#84431,#84432,#84433,#84434,#84435,#84436,#84437,#84438,#84439,#84440,#84441,
#84442,#84443,#84444,#84445,#84446,#84447,#84448,#84449,#84450,#84451,#84452,
#84453,#84454,#84455,#84456,#84457,#84458,#84459,#84460,#84461,#84462,#84463,
#84464,#84465,#84466,#84467,#84468,#84469,#84470,#84471,#84472,#84473,#84474,
#84475,#84476,#84477,#84478,#84479,#84480,#84481,#84482,#84483,#84484,#84485,
#84486,#84487,#84488,#84489,#84490,#84491,#84492,#84493,#84494,#84495,#84496,
#84497,#84498,#84499,#84500,#84501,#84502,#84503,#84504,#84505,#84506,#84507,
#84508,#84509,#84510,#84511,#84512,#84513,#84514,#84515,#84516,#84517,#84518,
#84519,#84520,#84521,#84522,#84523,#84524,#84525,#84526,#84527,#84528,#84529,
#84530,#84531,#84532),.UNSPECIFIED.,.F.,.F.,(4,3,3,3,3,3,3,3,3,3,3,3,3,
3,3,3,3,3,3,3,3,3,3,3,3,3,3,3,3,3,3,3,3,3,3,3,3,3,3,4),(-48.0752275700732,
-47.8597259048151,-47.8155038333859,-47.6461701715708,-47.4771643694644,
-47.3081875851609,-47.1392553092885,-46.9699199519336,-46.8193475035237,
-46.6500138417084,-46.4810080396019,-46.3120312552982,-46.1430989794257,
-45.9737636220706,-45.8231911736615,-45.6538575118462,-45.4848517097396,
-45.3158749254359,-45.1469426495634,-44.9776072922083,-44.8270348437993,
-44.657701181984,-44.4886953798776,-44.3197185955739,-44.1507863197014,
-43.9814509623464,-43.8308785139371,-43.6615448521218,-43.4925390500153,
-43.3235622657117,-43.1546299898391,-42.9852946324841,-42.8347221840749,
-42.6653885222596,-42.4963827201531,-42.3274059358494,-42.1584736599769,
-41.9891383026218,-41.8385658542127,-41.7920422632082),.UNSPECIFIED.);
#1129=B_SPLINE_CURVE_WITH_KNOTS('',3,(#84534,#84535,#84536,#84537,#84538,
#84539,#84540,#84541,#84542,#84543,#84544,#84545,#84546,#84547,#84548,#84549,
#84550,#84551,#84552,#84553,#84554,#84555,#84556,#84557,#84558,#84559,#84560,
#84561,#84562,#84563,#84564,#84565,#84566,#84567,#84568,#84569,#84570,#84571,
#84572,#84573,#84574,#84575,#84576,#84577,#84578,#84579,#84580,#84581,#84582,
#84583,#84584,#84585,#84586,#84587,#84588,#84589,#84590,#84591,#84592,#84593,
#84594,#84595,#84596,#84597,#84598,#84599,#84600,#84601,#84602,#84603,#84604,
#84605,#84606,#84607,#84608,#84609,#84610,#84611,#84612,#84613,#84614,#84615,
#84616,#84617,#84618,#84619,#84620,#84621,#84622,#84623,#84624,#84625,#84626,
#84627,#84628,#84629,#84630,#84631,#84632,#84633,#84634,#84635,#84636,#84637,
#84638,#84639,#84640,#84641,#84642,#84643,#84644,#84645,#84646,#84647,#84648),
 .UNSPECIFIED.,.F.,.F.,(4,3,3,3,3,3,3,3,3,3,3,3,3,3,3,3,3,3,3,3,3,3,3,3,
3,3,3,3,3,3,3,3,3,3,3,3,3,3,4),(-41.7920422629071,-41.6239457944974,-41.456165739063,
-41.2884054719728,-41.1206712858633,-40.9525563903589,-40.8424095243505,
-40.6730758625352,-40.5040700604288,-40.3350932761251,-40.1661610002525,
-39.9968256428975,-39.8462531944883,-39.6769195326731,-39.5079137305666,
-39.338936946263,-39.1700046703904,-39.0006693130355,-38.8500968646261,
-38.6807632028108,-38.5117574007042,-38.3427806164005,-38.1738483405279,
-38.0045129831728,-37.8539405347639,-37.6846068729486,-37.5156010708421,
-37.3466242865385,-37.1776920106659,-37.0083566533109,-36.8577842049017,
-36.6884505430866,-36.5194447409802,-36.3504679566768,-36.1815356808044,
-36.0122003234496,-35.8616278750395,-35.6675649622913,-35.5088571949304),
 .UNSPECIFIED.);
#1130=B_SPLINE_CURVE_WITH_KNOTS('',3,(#84650,#84651,#84652,#84653,#84654,
#84655,#84656,#84657,#84658,#84659),.UNSPECIFIED.,.F.,.F.,(4,1,1,1,1,1,
1,4),(-35.5088569560286,-34.8654715451773,-33.869315215315,-32.8731588854528,
-31.8770025555906,-30.8808462257284,-29.8846898958662,-29.225671648849),
 .UNSPECIFIED.);
#1131=B_SPLINE_CURVE_WITH_KNOTS('',3,(#84661,#84662,#84663,#84664,#84665,
#84666,#84667,#84668,#84669,#84670),.UNSPECIFIED.,.F.,.F.,(4,1,1,1,1,1,
1,4),(-29.225671648849,-28.888533566004,-27.8923772361418,-26.8962209062796,
-25.9000645764174,-24.9039082465552,-23.907751916693,-22.9424863416694),
 .UNSPECIFIED.);
#1132=B_SPLINE_CURVE_WITH_KNOTS('',3,(#84672,#84673,#84674,#84675,#84676,
#84677,#84678,#84679,#84680,#84681,#84682),.UNSPECIFIED.,.F.,.F.,(4,1,1,
1,1,1,1,1,4),(-22.9424863416694,-22.9115955868308,-21.9154392569686,-20.9192829271064,
-19.9231265972441,-18.9269702673819,-17.9308139375197,-16.9346576076575,
-16.6593049270061),.UNSPECIFIED.);
#1133=B_SPLINE_CURVE_WITH_KNOTS('',3,(#84684,#84685,#84686,#84687,#84688,
#84689,#84690,#84691,#84692,#84693,#84694,#84695,#84696,#84697,#84698,#84699,
#84700,#84701,#84702,#84703,#84704,#84705,#84706,#84707,#84708,#84709,#84710,
#84711,#84712,#84713,#84714,#84715,#84716,#84717,#84718,#84719,#84720,#84721,
#84722,#84723,#84724,#84725,#84726,#84727,#84728,#84729,#84730,#84731,#84732,
#84733,#84734,#84735,#84736,#84737,#84738,#84739,#84740,#84741,#84742,#84743,
#84744,#84745,#84746,#84747,#84748,#84749,#84750,#84751,#84752,#84753,#84754,
#84755,#84756,#84757,#84758,#84759,#84760,#84761,#84762,#84763,#84764,#84765,
#84766,#84767,#84768,#84769,#84770,#84771,#84772,#84773,#84774,#84775,#84776,
#84777,#84778,#84779,#84780,#84781,#84782,#84783,#84784,#84785,#84786,#84787,
#84788,#84789,#84790,#84791,#84792,#84793,#84794,#84795,#84796,#84797,#84798,
#84799,#84800,#84801),.UNSPECIFIED.,.F.,.F.,(4,3,3,3,3,3,3,3,3,3,3,3,3,
3,3,3,3,3,3,3,3,3,3,3,3,3,3,3,3,3,3,3,3,3,3,3,3,3,3,4),(-16.6593010344898,
-16.4918869660773,-16.3244404407765,-16.1569698807986,-15.9891309057531,
-15.9385012777953,-15.7691675865852,-15.6001617563704,-15.4311849462951,
-15.2622526458884,-15.0929172665271,-14.9423449479331,-14.7730110061835,
-14.6040049222631,-14.4350278574257,-14.2660953012303,-14.0967596698059,
-13.9461886180709,-13.776855645198,-13.6078505312393,-13.4388744238898,
-13.2699428200133,-13.1006081124298,-12.9500322882087,-12.7806982175314,
-12.6116920150786,-12.4427148490098,-12.2737822009037,-12.1044464946493,
-11.9538759583465,-11.7845406294793,-11.6155331455289,-11.4465546816653,
-11.2776207245426,-11.1082837186434,-10.9577196284843,-10.785155110263,
-10.6129857262874,-10.4410898767007,-10.3761157273103),.UNSPECIFIED.);
#1134=B_SPLINE_CURVE_WITH_KNOTS('',3,(#84802,#84803,#84804,#84805,#84806,
#84807,#84808,#84809,#84810,#84811,#84812,#84813,#84814,#84815,#84816,#84817,
#84818,#84819,#84820,#84821,#84822,#84823,#84824,#84825,#84826,#84827,#84828,
#84829,#84830,#84831,#84832,#84833,#84834,#84835,#84836,#84837,#84838,#84839,
#84840,#84841,#84842,#84843,#84844,#84845,#84846,#84847,#84848,#84849,#84850,
#84851,#84852,#84853,#84854,#84855,#84856,#84857,#84858,#84859,#84860,#84861,
#84862,#84863,#84864,#84865,#84866,#84867,#84868,#84869,#84870,#84871,#84872,
#84873,#84874,#84875,#84876,#84877,#84878,#84879,#84880,#84881,#84882,#84883,
#84884,#84885,#84886,#84887,#84888,#84889,#84890,#84891,#84892,#84893,#84894,
#84895,#84896,#84897,#84898,#84899,#84900,#84901,#84902,#84903,#84904,#84905,
#84906,#84907,#84908,#84909,#84910,#84911,#84912,#84913,#84914,#84915,#84916,
#84917,#84918,#84919),.UNSPECIFIED.,.F.,.F.,(4,3,3,3,3,3,3,3,3,3,3,3,3,
3,3,3,3,3,3,3,3,3,3,3,3,3,3,3,3,3,3,3,3,3,3,3,3,3,3,4),(-10.3761157271227,
-10.1914014079995,-10.0053992180424,-9.96156329862207,-9.79222542748429,
-9.62321547087196,-9.45423467460939,-9.28529845800698,-9.11595935874042,
-8.96540696875987,-8.79606394541769,-8.62704866921784,-8.45806237992334,
-8.28912056546132,-8.11977581610114,-7.96925063889766,-7.7999517813462,
-7.63098081674628,-7.46203841417896,-7.29314033051832,-7.12383813689975,
-6.97309430903545,-6.80372247429962,-6.6346788411425,-6.46566528890928,
-6.29669676477763,-6.12732676810572,-5.97693797917325,-5.80755632104186,
-5.63850168868863,-5.46947553628278,-5.30049351124867,-5.13110883596115,
-4.98078164931104,-4.8138683916711,-4.64727985048099,-4.48074211867273,
-4.314230116654,-4.14740991101127,-4.09293042013066),.UNSPECIFIED.);
#1135=B_SPLINE_CURVE_WITH_KNOTS('',3,(#84922,#84923,#84924,#84925,#84926,
#84927,#84928,#84929,#84930,#84931,#84932,#84933,#84934,#84935,#84936,#84937,
#84938,#84939,#84940,#84941,#84942,#84943,#84944,#84945,#84946,#84947,#84948,
#84949,#84950,#84951,#84952,#84953,#84954,#84955,#84956,#84957,#84958,#84959,
#84960,#84961,#84962,#84963,#84964,#84965,#84966,#84967,#84968,#84969,#84970,
#84971,#84972,#84973,#84974,#84975,#84976,#84977,#84978,#84979,#84980,#84981,
#84982,#84983,#84984,#84985,#84986,#84987,#84988,#84989,#84990,#84991,#84992,
#84993,#84994,#84995,#84996,#84997,#84998,#84999,#85000,#85001,#85002,#85003,
#85004,#85005,#85006,#85007,#85008,#85009,#85010,#85011,#85012,#85013,#85014,
#85015,#85016,#85017,#85018,#85019,#85020,#85021,#85022,#85023,#85024,#85025,
#85026,#85027,#85028,#85029,#85030,#85031,#85032,#85033,#85034,#85035,#85036,
#85037,#85038,#85039,#85040,#85041,#85042,#85043,#85044,#85045,#85046,#85047,
#85048,#85049,#85050,#85051,#85052,#85053,#85054,#85055,#85056,#85057,#85058,
#85059,#85060,#85061,#85062,#85063,#85064,#85065,#85066,#85067,#85068,#85069,
#85070,#85071,#85072,#85073,#85074,#85075,#85076,#85077,#85078,#85079,#85080,
#85081),.UNSPECIFIED.,.F.,.F.,(4,2,2,2,2,2,2,2,2,2,2,2,2,2,2,2,2,2,2,2,
2,2,2,2,2,2,2,2,2,2,2,2,2,2,2,2,2,2,2,2,2,2,2,2,2,2,2,2,2,2,2,2,2,2,2,2,
2,2,2,2,2,2,2,2,2,2,2,2,2,2,2,2,2,2,2,2,2,2,2,4),(0.0037894336419437,0.0430356641860205,
0.0816654995582311,0.0944090195370889,0.10028843357464,0.104826742950533,
0.109844865848441,0.118215085431042,0.158714606729488,0.18953617842965,
0.203985206295049,0.213340553110937,0.216833118665897,0.216873434713236,
0.21691409292274,0.216955135511277,0.21699660669252,0.217038552916791,0.217081023126943,
0.21962791747299,0.222392878739332,0.227007458458016,0.244659730636135,
0.283265341964775,0.316028949995482,0.328266850645602,0.334014749141327,
0.338491571663838,0.343480349474412,0.351886723920434,0.39549170993468,
0.432154251058751,0.443340737203487,0.451101966433715,0.454477510257664,
0.456985700903143,0.459871212205737,0.465002090560286,0.495183546490613,
0.501954524685721,0.53129663610334,0.561154378227613,0.568873002424849,
0.57367596829627,0.578130790318737,0.583959426123131,0.597265089807999,
0.652012489915787,0.674374418380701,0.686862979979659,0.69087766331876,
0.693487609183072,0.695821509488802,0.699679311169684,0.709878809040578,
0.754382509818591,0.790721901918114,0.80311274421278,0.808879711359274,
0.813349033484928,0.818306542891483,0.826604873211624,0.863880795845579,
0.916066721898791,0.924649096982799,0.928166674428858,0.930704235403835,
0.933544348212949,0.938544735806543,0.961543109543472,1.02756233922703,
1.03971098335327,1.04542649467273,1.04988097155688,1.05484728448991,1.06322075096602,
1.10523472414197,1.13607244536971,1.15885208833088,1.16366148960649),
 .UNSPECIFIED.);
#1136=B_SPLINE_CURVE_WITH_KNOTS('',3,(#85085,#85086,#85087,#85088,#85089,
#85090,#85091,#85092,#85093,#85094,#85095,#85096,#85097,#85098,#85099,#85100,
#85101,#85102,#85103,#85104,#85105,#85106,#85107,#85108,#85109,#85110,#85111,
#85112,#85113,#85114,#85115,#85116,#85117,#85118,#85119,#85120,#85121,#85122,
#85123,#85124,#85125,#85126,#85127),.UNSPECIFIED.,.F.,.F.,(4,3,3,3,3,3,
3,3,3,3,3,3,3,3,4),(103.672557568796,103.902573542604,103.938485219173,
104.115263612104,104.291682738526,104.468102235349,104.644505119859,104.821378175675,
104.934641549035,105.118296438428,105.301515543515,105.48449990958,105.667333099215,
105.850293575283,105.930797878897),.UNSPECIFIED.);
#1137=B_SPLINE_CURVE_WITH_KNOTS('',3,(#85128,#85129,#85130,#85131,#85132,
#85133,#85134,#85135,#85136,#85137,#85138,#85139,#85140,#85141,#85142,#85143,
#85144,#85145,#85146,#85147,#85148,#85149,#85150,#85151,#85152,#85153,#85154,
#85155,#85156,#85157,#85158,#85159,#85160,#85161,#85162,#85163,#85164,#85165,
#85166,#85167,#85168,#85169,#85170,#85171,#85172,#85173,#85174,#85175,#85176,
#85177),.UNSPECIFIED.,.F.,.F.,(4,2,2,2,2,2,2,2,2,2,2,2,2,2,2,2,2,2,2,2,
2,2,2,2,4),(-2.98914753351539,-2.95921878800075,-2.94518237031271,-2.93931598206595,
-2.93485723662925,-2.93029823022713,-2.92535465387828,-2.91733473317169,
-2.8871990170832,-2.84176481800093,-2.82559177589516,-2.81999954053876,
-2.81687727857855,-2.81432736386882,-2.81108041717311,-2.8041445851037,
-2.77114378395878,-2.74348280282388,-2.71161027045087,-2.70371041291119,
-2.69882975919512,-2.69432439898856,-2.68845850206672,-2.67518725330161,
-2.65783630003039),.UNSPECIFIED.);
#1138=B_SPLINE_CURVE_WITH_KNOTS('',3,(#85181,#85182,#85183,#85184,#85185,
#85186,#85187,#85188,#85189,#85190,#85191,#85192,#85193,#85194,#85195,#85196,
#85197,#85198,#85199,#85200,#85201,#85202,#85203,#85204,#85205,#85206,#85207,
#85208,#85209,#85210,#85211,#85212,#85213,#85214,#85215,#85216,#85217,#85218,
#85219,#85220,#85221,#85222,#85223,#85224,#85225,#85226,#85227,#85228,#85229,
#85230,#85231,#85232,#85233,#85234,#85235,#85236,#85237,#85238),
 .UNSPECIFIED.,.F.,.F.,(4,3,3,3,3,3,3,3,3,3,3,3,3,3,3,3,3,3,3,4),(-0.547417054864566,
-0.53033882791749,-0.495307986319534,-0.475290491773116,-0.447607237097599,
-0.419654534866616,-0.400079102935313,-0.381999937381865,-0.332300949859174,
-0.29983044961068,-0.283628237747696,-0.251952142272621,-0.205914518250308,
-0.18058812353789,-0.13617659674883,-0.103458346379604,-0.0834567189867998,
-0.0389725148624793,-0.00294201638164863,0.),.UNSPECIFIED.);
#1139=B_SPLINE_CURVE_WITH_KNOTS('',3,(#85240,#85241,#85242,#85243),
 .UNSPECIFIED.,.F.,.F.,(4,4),(0.,0.0130412808333173),.UNSPECIFIED.);
#1140=B_SPLINE_CURVE_WITH_KNOTS('',3,(#85244,#85245,#85246,#85247,#85248,
#85249,#85250,#85251,#85252,#85253,#85254,#85255,#85256,#85257,#85258,#85259,
#85260,#85261,#85262,#85263,#85264,#85265,#85266,#85267,#85268,#85269,#85270,
#85271,#85272,#85273,#85274,#85275,#85276,#85277,#85278,#85279,#85280,#85281,
#85282,#85283,#85284,#85285,#85286,#85287,#85288,#85289,#85290,#85291,#85292,
#85293,#85294,#85295,#85296,#85297,#85298,#85299,#85300,#85301),
 .UNSPECIFIED.,.F.,.F.,(4,3,3,3,3,3,3,3,3,3,3,3,3,3,3,3,3,3,3,4),(-0.555272788399386,
-0.536878011109323,-0.499667654095302,-0.47690792776006,-0.441414459291682,
-0.425702691834984,-0.411668346210502,-0.363225278150133,-0.331446939414361,
-0.313088391824243,-0.28194190366226,-0.246699165704478,-0.225030257188244,
-0.2082576414013,-0.156193231050975,-0.129811100532013,-0.111596852253624,
-0.0945316768920992,-0.0422149050010466,0.),.UNSPECIFIED.);
#1141=B_SPLINE_CURVE_WITH_KNOTS('',3,(#85706,#85707,#85708,#85709),
 .UNSPECIFIED.,.F.,.F.,(4,4),(-0.00534461024793257,0.),.UNSPECIFIED.);
#1142=B_SPLINE_CURVE_WITH_KNOTS('',3,(#85710,#85711,#85712,#85713,#85714,
#85715,#85716,#85717,#85718,#85719,#85720,#85721,#85722,#85723,#85724,#85725,
#85726,#85727,#85728,#85729,#85730,#85731,#85732,#85733,#85734,#85735,#85736,
#85737,#85738,#85739,#85740,#85741,#85742,#85743,#85744,#85745,#85746,#85747,
#85748,#85749,#85750,#85751,#85752,#85753,#85754,#85755,#85756,#85757,#85758,
#85759,#85760,#85761,#85762,#85763,#85764,#85765,#85766,#85767),
 .UNSPECIFIED.,.F.,.F.,(4,3,3,3,3,3,3,3,3,3,3,3,3,3,3,3,3,3,3,4),(-0.555272788399383,
-0.536878011109319,-0.49966765582956,-0.476907936094555,-0.441413399121164,
-0.425725415706225,-0.411671954797729,-0.363223558783216,-0.331446021165907,
-0.313087741258502,-0.281941903662256,-0.246699165704475,-0.225030248355765,
-0.208257626954711,-0.156193220216035,-0.129811093853198,-0.111596847794653,
-0.094531660643926,-0.0422148723537678,-6.70332118037912E-15),
 .UNSPECIFIED.);
#1143=B_SPLINE_CURVE_WITH_KNOTS('',3,(#85773,#85774,#85775,#85776,#85777,
#85778,#85779,#85780,#85781,#85782,#85783,#85784,#85785,#85786,#85787,#85788,
#85789,#85790,#85791,#85792,#85793,#85794,#85795,#85796,#85797,#85798,#85799,
#85800,#85801,#85802,#85803,#85804,#85805,#85806,#85807,#85808,#85809,#85810,
#85811,#85812,#85813,#85814,#85815,#85816,#85817,#85818,#85819,#85820,#85821,
#85822,#85823,#85824,#85825,#85826,#85827,#85828,#85829,#85830),
 .UNSPECIFIED.,.F.,.F.,(4,3,3,3,3,3,3,3,3,3,3,3,3,3,3,3,3,3,3,4),(-0.5474172947136,
-0.530338827917456,-0.495308046545021,-0.475290501025032,-0.447608014023609,
-0.419656418536863,-0.400079548458063,-0.382001269621687,-0.332302227775843,
-0.299831205494185,-0.283628559844453,-0.251952142272604,-0.205910804141385,
-0.180596553086976,-0.136182931568932,-0.103452591178888,-0.0834625820348813,
-0.0389782829583399,-0.00294206701479738,0.),.UNSPECIFIED.);
#1144=B_SPLINE_CURVE_WITH_KNOTS('',3,(#86235,#86236,#86237,#86238),
 .UNSPECIFIED.,.F.,.F.,(4,4),(0.,0.00538265464589753),.UNSPECIFIED.);
#1344=CONICAL_SURFACE('',#17215,0.320138837486628,1.0471975511966);
#1345=CONICAL_SURFACE('',#17220,0.1225,1.0267507402002);
#1346=CONICAL_SURFACE('',#17235,0.2775,0.785398163397449);
#1347=CONICAL_SURFACE('',#17236,0.49,0.785398163397449);
#1581=CYLINDRICAL_SURFACE('',#17182,0.237175);
#1582=CYLINDRICAL_SURFACE('',#17184,0.237175);
#1583=CYLINDRICAL_SURFACE('',#17185,0.237175);
#1584=CYLINDRICAL_SURFACE('',#17186,0.237175);
#1585=CYLINDRICAL_SURFACE('',#17187,0.237175);
#1586=CYLINDRICAL_SURFACE('',#17188,0.237175);
#1587=CYLINDRICAL_SURFACE('',#17189,0.237175);
#1588=CYLINDRICAL_SURFACE('',#17190,0.237175);
#1589=CYLINDRICAL_SURFACE('',#17191,0.237175);
#1590=CYLINDRICAL_SURFACE('',#17192,0.237175);
#1591=CYLINDRICAL_SURFACE('',#17193,0.237175);
#1592=CYLINDRICAL_SURFACE('',#17194,0.237175);
#1593=CYLINDRICAL_SURFACE('',#17195,0.237175);
#1594=CYLINDRICAL_SURFACE('',#17196,0.237175);
#1595=CYLINDRICAL_SURFACE('',#17197,0.237175);
#1596=CYLINDRICAL_SURFACE('',#17198,0.2942);
#1597=CYLINDRICAL_SURFACE('',#17203,0.237175);
#1598=CYLINDRICAL_SURFACE('',#17230,0.5);
#1749=FACE_BOUND('',#4251,.T.);
#1750=FACE_BOUND('',#4261,.T.);
#1751=FACE_BOUND('',#4265,.T.);
#2357=CIRCLE('',#17183,0.237175);
#2358=CIRCLE('',#17199,0.2942);
#2359=CIRCLE('',#17200,0.295065672210827);
#2360=CIRCLE('',#17201,0.2942);
#2361=CIRCLE('',#17202,0.2942);
#2362=CIRCLE('',#17204,0.237175);
#2363=CIRCLE('',#17206,0.2942);
#2364=CIRCLE('',#17208,0.2942);
#2365=CIRCLE('',#17209,0.2942);
#2366=CIRCLE('',#17211,0.3342);
#2367=CIRCLE('',#17212,0.04);
#2368=CIRCLE('',#17214,0.48);
#2369=CIRCLE('',#17216,0.308675134594813);
#2370=CIRCLE('',#17221,0.243346949651439);
#2371=CIRCLE('',#17227,0.44);
#2372=CIRCLE('',#17228,0.06);
#2373=CIRCLE('',#17229,0.5);
#2374=CIRCLE('',#17231,0.5);
#2375=CIRCLE('',#17234,0.255);
#3209=FACE_OUTER_BOUND('',#4228,.T.);
#3210=FACE_OUTER_BOUND('',#4229,.T.);
#3211=FACE_OUTER_BOUND('',#4230,.T.);
#3212=FACE_OUTER_BOUND('',#4231,.T.);
#3213=FACE_OUTER_BOUND('',#4232,.T.);
#3214=FACE_OUTER_BOUND('',#4233,.T.);
#3215=FACE_OUTER_BOUND('',#4234,.T.);
#3216=FACE_OUTER_BOUND('',#4235,.T.);
#3217=FACE_OUTER_BOUND('',#4236,.T.);
#3218=FACE_OUTER_BOUND('',#4237,.T.);
#3219=FACE_OUTER_BOUND('',#4238,.T.);
#3220=FACE_OUTER_BOUND('',#4239,.T.);
#3221=FACE_OUTER_BOUND('',#4240,.T.);
#3222=FACE_OUTER_BOUND('',#4241,.T.);
#3223=FACE_OUTER_BOUND('',#4242,.T.);
#3224=FACE_OUTER_BOUND('',#4243,.T.);
#3225=FACE_OUTER_BOUND('',#4244,.T.);
#3226=FACE_OUTER_BOUND('',#4245,.T.);
#3227=FACE_OUTER_BOUND('',#4246,.T.);
#3228=FACE_OUTER_BOUND('',#4247,.T.);
#3229=FACE_OUTER_BOUND('',#4248,.T.);
#3230=FACE_OUTER_BOUND('',#4249,.T.);
#3231=FACE_OUTER_BOUND('',#4250,.T.);
#3232=FACE_OUTER_BOUND('',#4252,.T.);
#3233=FACE_OUTER_BOUND('',#4253,.T.);
#3234=FACE_OUTER_BOUND('',#4254,.T.);
#3235=FACE_OUTER_BOUND('',#4255,.T.);
#3236=FACE_OUTER_BOUND('',#4256,.T.);
#3237=FACE_OUTER_BOUND('',#4257,.T.);
#3238=FACE_OUTER_BOUND('',#4258,.T.);
#3239=FACE_OUTER_BOUND('',#4259,.T.);
#3240=FACE_OUTER_BOUND('',#4260,.T.);
#3241=FACE_OUTER_BOUND('',#4262,.T.);
#3242=FACE_OUTER_BOUND('',#4263,.T.);
#3243=FACE_OUTER_BOUND('',#4264,.T.);
#3244=FACE_OUTER_BOUND('',#4266,.T.);
#3245=FACE_OUTER_BOUND('',#4267,.T.);
#3246=FACE_OUTER_BOUND('',#4268,.T.);
#4228=EDGE_LOOP('',(#14137,#14138,#14139,#14140));
#4229=EDGE_LOOP('',(#14141,#14142,#14143,#14144,#14145,#14146));
#4230=EDGE_LOOP('',(#14147,#14148,#14149,#14150,#14151));
#4231=EDGE_LOOP('',(#14152,#14153,#14154,#14155,#14156));
#4232=EDGE_LOOP('',(#14157,#14158,#14159,#14160,#14161));
#4233=EDGE_LOOP('',(#14162,#14163,#14164,#14165,#14166));
#4234=EDGE_LOOP('',(#14167,#14168,#14169,#14170,#14171));
#4235=EDGE_LOOP('',(#14172,#14173,#14174,#14175,#14176,#14177));
#4236=EDGE_LOOP('',(#14178,#14179,#14180,#14181,#14182));
#4237=EDGE_LOOP('',(#14183,#14184,#14185,#14186,#14187));
#4238=EDGE_LOOP('',(#14188,#14189,#14190,#14191,#14192));
#4239=EDGE_LOOP('',(#14193,#14194,#14195,#14196,#14197));
#4240=EDGE_LOOP('',(#14198,#14199,#14200,#14201,#14202));
#4241=EDGE_LOOP('',(#14203,#14204,#14205,#14206,#14207));
#4242=EDGE_LOOP('',(#14208,#14209,#14210,#14211,#14212));
#4243=EDGE_LOOP('',(#14213,#14214,#14215,#14216,#14217,#14218,#14219,#14220,
#14221,#14222,#14223,#14224,#14225,#14226,#14227,#14228,#14229,#14230,#14231,
#14232,#14233,#14234,#14235,#14236,#14237,#14238,#14239,#14240,#14241,#14242,
#14243,#14244,#14245,#14246,#14247,#14248));
#4244=EDGE_LOOP('',(#14249,#14250,#14251,#14252,#14253));
#4245=EDGE_LOOP('',(#14254,#14255,#14256,#14257,#14258));
#4246=EDGE_LOOP('',(#14259,#14260,#14261,#14262,#14263,#14264,#14265,#14266,
#14267,#14268,#14269,#14270,#14271,#14272,#14273,#14274,#14275,#14276,#14277,
#14278,#14279,#14280,#14281,#14282,#14283,#14284,#14285,#14286,#14287,#14288,
#14289,#14290,#14291,#14292,#14293,#14294,#14295,#14296,#14297,#14298,#14299,
#14300,#14301,#14302));
#4247=EDGE_LOOP('',(#14303,#14304,#14305,#14306,#14307));
#4248=EDGE_LOOP('',(#14308,#14309,#14310,#14311,#14312,#14313,#14314,#14315,
#14316,#14317,#14318,#14319,#14320,#14321,#14322,#14323,#14324,#14325,#14326,
#14327,#14328,#14329,#14330,#14331,#14332,#14333,#14334,#14335,#14336,#14337,
#14338,#14339,#14340,#14341,#14342,#14343,#14344,#14345,#14346,#14347,#14348,
#14349,#14350,#14351,#14352));
#4249=EDGE_LOOP('',(#14353,#14354,#14355,#14356,#14357,#14358,#14359));
#4250=EDGE_LOOP('',(#14360));
#4251=EDGE_LOOP('',(#14361));
#4252=EDGE_LOOP('',(#14362,#14363,#14364,#14365,#14366,#14367,#14368,#14369,
#14370,#14371));
#4253=EDGE_LOOP('',(#14372,#14373,#14374,#14375));
#4254=EDGE_LOOP('',(#14376,#14377,#14378,#14379));
#4255=EDGE_LOOP('',(#14380,#14381,#14382,#14383));
#4256=EDGE_LOOP('',(#14384,#14385,#14386));
#4257=EDGE_LOOP('',(#14387,#14388,#14389,#14390));
#4258=EDGE_LOOP('',(#14391,#14392,#14393,#14394));
#4259=EDGE_LOOP('',(#14395,#14396,#14397,#14398,#14399));
#4260=EDGE_LOOP('',(#14400,#14401,#14402,#14403,#14404,#14405));
#4261=EDGE_LOOP('',(#14406));
#4262=EDGE_LOOP('',(#14407,#14408,#14409,#14410));
#4263=EDGE_LOOP('',(#14411,#14412,#14413,#14414));
#4264=EDGE_LOOP('',(#14415));
#4265=EDGE_LOOP('',(#14416));
#4266=EDGE_LOOP('',(#14417));
#4267=EDGE_LOOP('',(#14418,#14419,#14420,#14421,#14422,#14423,#14424));
#4268=EDGE_LOOP('',(#14425,#14426,#14427,#14428));
#5103=LINE('',#77450,#5963);
#5104=LINE('',#77582,#5964);
#5105=LINE('',#77811,#5965);
#5106=LINE('',#78183,#5966);
#5107=LINE('',#78594,#5967);
#5108=LINE('',#79043,#5968);
#5109=LINE('',#79450,#5969);
#5110=LINE('',#79779,#5970);
#5111=LINE('',#80054,#5971);
#5112=LINE('',#80417,#5972);
#5113=LINE('',#80824,#5973);
#5114=LINE('',#81239,#5974);
#5115=LINE('',#81638,#5975);
#5116=LINE('',#82035,#5976);
#5117=LINE('',#82440,#5977);
#5118=LINE('',#86276,#5978);
#5119=LINE('',#86280,#5979);
#5120=LINE('',#86282,#5980);
#5121=LINE('',#86283,#5981);
#5122=LINE('',#86286,#5982);
#5123=LINE('',#86287,#5983);
#5124=LINE('',#86290,#5984);
#5125=LINE('',#86291,#5985);
#5126=LINE('',#86295,#5986);
#5127=LINE('',#86299,#5987);
#5128=LINE('',#86300,#5988);
#5129=LINE('',#86303,#5989);
#5130=LINE('',#86304,#5990);
#5131=LINE('',#86306,#5991);
#5132=LINE('',#86316,#5992);
#5133=LINE('',#86323,#5993);
#5134=LINE('',#86325,#5994);
#5963=VECTOR('',#20814,0.237175);
#5964=VECTOR('',#20819,0.237175);
#5965=VECTOR('',#20822,0.237175);
#5966=VECTOR('',#20825,0.237175);
#5967=VECTOR('',#20828,0.237175);
#5968=VECTOR('',#20831,0.237175);
#5969=VECTOR('',#20834,0.237175);
#5970=VECTOR('',#20837,0.237175);
#5971=VECTOR('',#20840,0.237175);
#5972=VECTOR('',#20843,0.237175);
#5973=VECTOR('',#20846,0.237175);
#5974=VECTOR('',#20849,0.237175);
#5975=VECTOR('',#20852,0.237175);
#5976=VECTOR('',#20855,0.237175);
#5977=VECTOR('',#20858,0.237175);
#5978=VECTOR('',#20895,0.320138837486628);
#5979=VECTOR('',#20900,1.);
#5980=VECTOR('',#20901,1.);
#5981=VECTOR('',#20902,1.);
#5982=VECTOR('',#20905,1.);
#5983=VECTOR('',#20906,1.);
#5984=VECTOR('',#20909,1.);
#5985=VECTOR('',#20910,1.);
#5986=VECTOR('',#20913,0.1225);
#5987=VECTOR('',#20918,1.);
#5988=VECTOR('',#20919,1.);
#5989=VECTOR('',#20922,1.);
#5990=VECTOR('',#20923,1.);
#5991=VECTOR('',#20926,1.);
#5992=VECTOR('',#20939,0.5);
#5993=VECTOR('',#20950,0.2775);
#5994=VECTOR('',#20953,0.49);
#7425=VERTEX_POINT('',#77448);
#7426=VERTEX_POINT('',#77449);
#7427=VERTEX_POINT('',#77451);
#7428=VERTEX_POINT('',#77528);
#7429=VERTEX_POINT('',#77580);
#7430=VERTEX_POINT('',#77581);
#7431=VERTEX_POINT('',#77583);
#7432=VERTEX_POINT('',#77770);
#7433=VERTEX_POINT('',#77809);
#7434=VERTEX_POINT('',#77810);
#7435=VERTEX_POINT('',#78012);
#7436=VERTEX_POINT('',#78181);
#7437=VERTEX_POINT('',#78182);
#7438=VERTEX_POINT('',#78184);
#7439=VERTEX_POINT('',#78592);
#7440=VERTEX_POINT('',#78593);
#7441=VERTEX_POINT('',#78793);
#7442=VERTEX_POINT('',#79041);
#7443=VERTEX_POINT('',#79042);
#7444=VERTEX_POINT('',#79044);
#7445=VERTEX_POINT('',#79448);
#7446=VERTEX_POINT('',#79449);
#7447=VERTEX_POINT('',#79641);
#7448=VERTEX_POINT('',#79777);
#7449=VERTEX_POINT('',#79778);
#7450=VERTEX_POINT('',#79780);
#7451=VERTEX_POINT('',#80013);
#7452=VERTEX_POINT('',#80052);
#7453=VERTEX_POINT('',#80053);
#7454=VERTEX_POINT('',#80247);
#7455=VERTEX_POINT('',#80415);
#7456=VERTEX_POINT('',#80416);
#7457=VERTEX_POINT('',#80418);
#7458=VERTEX_POINT('',#80822);
#7459=VERTEX_POINT('',#80823);
#7460=VERTEX_POINT('',#81023);
#7461=VERTEX_POINT('',#81237);
#7462=VERTEX_POINT('',#81238);
#7463=VERTEX_POINT('',#81240);
#7464=VERTEX_POINT('',#81636);
#7465=VERTEX_POINT('',#81637);
#7466=VERTEX_POINT('',#81829);
#7467=VERTEX_POINT('',#82033);
#7468=VERTEX_POINT('',#82034);
#7469=VERTEX_POINT('',#82036);
#7470=VERTEX_POINT('',#82438);
#7471=VERTEX_POINT('',#82439);
#7472=VERTEX_POINT('',#82639);
#7473=VERTEX_POINT('',#82853);
#7474=VERTEX_POINT('',#82854);
#7475=VERTEX_POINT('',#82861);
#7476=VERTEX_POINT('',#82863);
#7477=VERTEX_POINT('',#82869);
#7478=VERTEX_POINT('',#82988);
#7479=VERTEX_POINT('',#83107);
#7480=VERTEX_POINT('',#83226);
#7481=VERTEX_POINT('',#83342);
#7482=VERTEX_POINT('',#83353);
#7483=VERTEX_POINT('',#83364);
#7484=VERTEX_POINT('',#83376);
#7485=VERTEX_POINT('',#83495);
#7486=VERTEX_POINT('',#83614);
#7487=VERTEX_POINT('',#83730);
#7488=VERTEX_POINT('',#83741);
#7489=VERTEX_POINT('',#83752);
#7490=VERTEX_POINT('',#83764);
#7491=VERTEX_POINT('',#83883);
#7492=VERTEX_POINT('',#83894);
#7493=VERTEX_POINT('',#83896);
#7494=VERTEX_POINT('',#83898);
#7495=VERTEX_POINT('',#83900);
#7496=VERTEX_POINT('',#83910);
#7497=VERTEX_POINT('',#84029);
#7498=VERTEX_POINT('',#84145);
#7499=VERTEX_POINT('',#84261);
#7500=VERTEX_POINT('',#84272);
#7501=VERTEX_POINT('',#84284);
#7502=VERTEX_POINT('',#84295);
#7503=VERTEX_POINT('',#84414);
#7504=VERTEX_POINT('',#84533);
#7505=VERTEX_POINT('',#84649);
#7506=VERTEX_POINT('',#84660);
#7507=VERTEX_POINT('',#84671);
#7508=VERTEX_POINT('',#84683);
#7509=VERTEX_POINT('',#84921);
#7510=VERTEX_POINT('',#85082);
#7511=VERTEX_POINT('',#85084);
#7512=VERTEX_POINT('',#85179);
#7513=VERTEX_POINT('',#85239);
#7514=VERTEX_POINT('',#85769);
#7515=VERTEX_POINT('',#85771);
#7516=VERTEX_POINT('',#86240);
#7517=VERTEX_POINT('',#86244);
#7518=VERTEX_POINT('',#86247);
#7519=VERTEX_POINT('',#86248);
#7520=VERTEX_POINT('',#86252);
#7521=VERTEX_POINT('',#86256);
#7522=VERTEX_POINT('',#86260);
#7523=VERTEX_POINT('',#86264);
#7524=VERTEX_POINT('',#86268);
#7525=VERTEX_POINT('',#86275);
#7526=VERTEX_POINT('',#86279);
#7527=VERTEX_POINT('',#86281);
#7528=VERTEX_POINT('',#86285);
#7529=VERTEX_POINT('',#86289);
#7530=VERTEX_POINT('',#86293);
#7531=VERTEX_POINT('',#86294);
#7532=VERTEX_POINT('',#86298);
#7533=VERTEX_POINT('',#86302);
#7534=VERTEX_POINT('',#86309);
#7535=VERTEX_POINT('',#86311);
#7536=VERTEX_POINT('',#86315);
#7537=VERTEX_POINT('',#86320);
#9690=EDGE_CURVE('',#7425,#7426,#5103,.T.);
#9691=EDGE_CURVE('',#7427,#7425,#1057,.T.);
#9692=EDGE_CURVE('',#7428,#7427,#2357,.T.);
#9693=EDGE_CURVE('',#7428,#7426,#1058,.T.);
#9694=EDGE_CURVE('',#7429,#7430,#5104,.T.);
#9695=EDGE_CURVE('',#7431,#7429,#1059,.F.);
#9696=EDGE_CURVE('',#7425,#7431,#1060,.T.);
#9697=EDGE_CURVE('',#7426,#7432,#1061,.T.);
#9698=EDGE_CURVE('',#7432,#7430,#1062,.T.);
#9699=EDGE_CURVE('',#7433,#7434,#5105,.T.);
#9700=EDGE_CURVE('',#7429,#7433,#1063,.F.);
#9701=EDGE_CURVE('',#7430,#7435,#1064,.T.);
#9702=EDGE_CURVE('',#7435,#7434,#1065,.T.);
#9703=EDGE_CURVE('',#7436,#7437,#5106,.T.);
#9704=EDGE_CURVE('',#7438,#7436,#1066,.F.);
#9705=EDGE_CURVE('',#7433,#7438,#1067,.F.);
#9706=EDGE_CURVE('',#7434,#7437,#1068,.T.);
#9707=EDGE_CURVE('',#7439,#7440,#5107,.T.);
#9708=EDGE_CURVE('',#7436,#7439,#1069,.F.);
#9709=EDGE_CURVE('',#7437,#7441,#1070,.T.);
#9710=EDGE_CURVE('',#7441,#7440,#1071,.T.);
#9711=EDGE_CURVE('',#7442,#7443,#5108,.T.);
#9712=EDGE_CURVE('',#7444,#7442,#1072,.F.);
#9713=EDGE_CURVE('',#7439,#7444,#1073,.F.);
#9714=EDGE_CURVE('',#7440,#7443,#1074,.T.);
#9715=EDGE_CURVE('',#7445,#7446,#5109,.T.);
#9716=EDGE_CURVE('',#7442,#7445,#1075,.F.);
#9717=EDGE_CURVE('',#7443,#7447,#1076,.T.);
#9718=EDGE_CURVE('',#7447,#7446,#1077,.T.);
#9719=EDGE_CURVE('',#7448,#7449,#5110,.T.);
#9720=EDGE_CURVE('',#7450,#7448,#1078,.F.);
#9721=EDGE_CURVE('',#7445,#7450,#1079,.F.);
#9722=EDGE_CURVE('',#7446,#7451,#1080,.T.);
#9723=EDGE_CURVE('',#7451,#7449,#1081,.T.);
#9724=EDGE_CURVE('',#7452,#7453,#5111,.T.);
#9725=EDGE_CURVE('',#7448,#7452,#1082,.F.);
#9726=EDGE_CURVE('',#7449,#7454,#1083,.T.);
#9727=EDGE_CURVE('',#7454,#7453,#1084,.T.);
#9728=EDGE_CURVE('',#7455,#7456,#5112,.T.);
#9729=EDGE_CURVE('',#7457,#7455,#1085,.F.);
#9730=EDGE_CURVE('',#7452,#7457,#1086,.F.);
#9731=EDGE_CURVE('',#7453,#7456,#1087,.T.);
#9732=EDGE_CURVE('',#7458,#7459,#5113,.T.);
#9733=EDGE_CURVE('',#7455,#7458,#1088,.F.);
#9734=EDGE_CURVE('',#7456,#7460,#1089,.T.);
#9735=EDGE_CURVE('',#7460,#7459,#1090,.T.);
#9736=EDGE_CURVE('',#7461,#7462,#5114,.T.);
#9737=EDGE_CURVE('',#7463,#7461,#1091,.F.);
#9738=EDGE_CURVE('',#7458,#7463,#1092,.F.);
#9739=EDGE_CURVE('',#7459,#7462,#1093,.T.);
#9740=EDGE_CURVE('',#7464,#7465,#5115,.T.);
#9741=EDGE_CURVE('',#7461,#7464,#1094,.F.);
#9742=EDGE_CURVE('',#7462,#7466,#1095,.T.);
#9743=EDGE_CURVE('',#7466,#7465,#1096,.T.);
#9744=EDGE_CURVE('',#7467,#7468,#5116,.T.);
#9745=EDGE_CURVE('',#7469,#7467,#1097,.F.);
#9746=EDGE_CURVE('',#7464,#7469,#1098,.F.);
#9747=EDGE_CURVE('',#7465,#7468,#1099,.T.);
#9748=EDGE_CURVE('',#7470,#7471,#5117,.T.);
#9749=EDGE_CURVE('',#7467,#7470,#1100,.F.);
#9750=EDGE_CURVE('',#7468,#7472,#1101,.T.);
#9751=EDGE_CURVE('',#7472,#7471,#1102,.F.);
#9752=EDGE_CURVE('',#7473,#7474,#1103,.T.);
#9753=EDGE_CURVE('',#7474,#7475,#2358,.T.);
#9754=EDGE_CURVE('',#7475,#7476,#1104,.T.);
#9755=EDGE_CURVE('',#7476,#7477,#1105,.T.);
#9756=EDGE_CURVE('',#7477,#7478,#1106,.T.);
#9757=EDGE_CURVE('',#7478,#7479,#1107,.T.);
#9758=EDGE_CURVE('',#7479,#7480,#1108,.T.);
#9759=EDGE_CURVE('',#7480,#7481,#1109,.T.);
#9760=EDGE_CURVE('',#7481,#7482,#1110,.T.);
#9761=EDGE_CURVE('',#7482,#7483,#1111,.T.);
#9762=EDGE_CURVE('',#7483,#7484,#1112,.T.);
#9763=EDGE_CURVE('',#7484,#7485,#1113,.T.);
#9764=EDGE_CURVE('',#7485,#7486,#1114,.T.);
#9765=EDGE_CURVE('',#7486,#7487,#1115,.T.);
#9766=EDGE_CURVE('',#7487,#7488,#1116,.T.);
#9767=EDGE_CURVE('',#7488,#7489,#1117,.T.);
#9768=EDGE_CURVE('',#7489,#7490,#1118,.T.);
#9769=EDGE_CURVE('',#7490,#7491,#1119,.T.);
#9770=EDGE_CURVE('',#7491,#7492,#2359,.T.);
#9771=EDGE_CURVE('',#7493,#7492,#2360,.T.);
#9772=EDGE_CURVE('',#7494,#7493,#2361,.T.);
#9773=EDGE_CURVE('',#7494,#7495,#1120,.T.);
#9774=EDGE_CURVE('',#7495,#7496,#1121,.T.);
#9775=EDGE_CURVE('',#7496,#7497,#1122,.T.);
#9776=EDGE_CURVE('',#7497,#7498,#1123,.T.);
#9777=EDGE_CURVE('',#7498,#7499,#1124,.T.);
#9778=EDGE_CURVE('',#7499,#7500,#1125,.T.);
#9779=EDGE_CURVE('',#7500,#7501,#1126,.T.);
#9780=EDGE_CURVE('',#7501,#7502,#1127,.T.);
#9781=EDGE_CURVE('',#7502,#7503,#1128,.T.);
#9782=EDGE_CURVE('',#7503,#7504,#1129,.T.);
#9783=EDGE_CURVE('',#7504,#7505,#1130,.T.);
#9784=EDGE_CURVE('',#7505,#7506,#1131,.T.);
#9785=EDGE_CURVE('',#7506,#7507,#1132,.T.);
#9786=EDGE_CURVE('',#7507,#7508,#1133,.T.);
#9787=EDGE_CURVE('',#7508,#7473,#1134,.T.);
#9788=EDGE_CURVE('',#7471,#7509,#1135,.F.);
#9789=EDGE_CURVE('',#7510,#7509,#2362,.T.);
#9790=EDGE_CURVE('',#7511,#7510,#1136,.T.);
#9791=EDGE_CURVE('',#7470,#7511,#1137,.F.);
#9792=EDGE_CURVE('',#7512,#7494,#2363,.T.);
#9793=EDGE_CURVE('',#7512,#7510,#1138,.T.);
#9794=EDGE_CURVE('',#7509,#7513,#1139,.T.);
#9795=EDGE_CURVE('',#7513,#7494,#1140,.T.);
#9796=EDGE_CURVE('',#7492,#7512,#1141,.T.);
#9797=EDGE_CURVE('',#7427,#7475,#1142,.T.);
#9798=EDGE_CURVE('',#7475,#7514,#2364,.T.);
#9799=EDGE_CURVE('',#7514,#7515,#2365,.T.);
#9800=EDGE_CURVE('',#7515,#7428,#1143,.T.);
#9801=EDGE_CURVE('',#7515,#7474,#1144,.T.);
#9802=EDGE_CURVE('',#7516,#7516,#2366,.T.);
#9803=EDGE_CURVE('',#7516,#7493,#2367,.T.);
#9804=EDGE_CURVE('',#7517,#7517,#2368,.T.);
#9805=EDGE_CURVE('',#7518,#7519,#280,.T.);
#9806=EDGE_CURVE('',#7520,#7518,#281,.T.);
#9807=EDGE_CURVE('',#7521,#7520,#282,.T.);
#9808=EDGE_CURVE('',#7522,#7521,#283,.T.);
#9809=EDGE_CURVE('',#7523,#7522,#284,.T.);
#9810=EDGE_CURVE('',#7524,#7523,#285,.T.);
#9811=EDGE_CURVE('',#7519,#7524,#286,.T.);
#9812=EDGE_CURVE('',#7519,#7525,#5118,.T.);
#9813=EDGE_CURVE('',#7525,#7525,#2369,.T.);
#9814=EDGE_CURVE('',#7523,#7526,#5119,.T.);
#9815=EDGE_CURVE('',#7526,#7527,#5120,.T.);
#9816=EDGE_CURVE('',#7524,#7527,#5121,.T.);
#9817=EDGE_CURVE('',#7522,#7528,#5122,.T.);
#9818=EDGE_CURVE('',#7528,#7526,#5123,.T.);
#9819=EDGE_CURVE('',#7521,#7529,#5124,.T.);
#9820=EDGE_CURVE('',#7529,#7528,#5125,.T.);
#9821=EDGE_CURVE('',#7530,#7531,#5126,.T.);
#9822=EDGE_CURVE('',#7531,#7531,#2370,.T.);
#9823=EDGE_CURVE('',#7520,#7532,#5127,.T.);
#9824=EDGE_CURVE('',#7532,#7529,#5128,.T.);
#9825=EDGE_CURVE('',#7518,#7533,#5129,.T.);
#9826=EDGE_CURVE('',#7533,#7532,#5130,.T.);
#9827=EDGE_CURVE('',#7527,#7533,#5131,.T.);
#9828=EDGE_CURVE('',#7534,#7534,#2371,.T.);
#9829=EDGE_CURVE('',#7534,#7535,#2372,.T.);
#9830=EDGE_CURVE('',#7535,#7535,#2373,.T.);
#9831=EDGE_CURVE('',#7535,#7536,#5132,.T.);
#9832=EDGE_CURVE('',#7536,#7536,#2374,.T.);
#9833=EDGE_CURVE('',#7537,#7537,#2375,.T.);
#9834=EDGE_CURVE('',#7514,#7537,#5133,.T.);
#9835=EDGE_CURVE('',#7536,#7517,#5134,.T.);
#14137=ORIENTED_EDGE('',*,*,#9690,.F.);
#14138=ORIENTED_EDGE('',*,*,#9691,.F.);
#14139=ORIENTED_EDGE('',*,*,#9692,.F.);
#14140=ORIENTED_EDGE('',*,*,#9693,.T.);
#14141=ORIENTED_EDGE('',*,*,#9694,.F.);
#14142=ORIENTED_EDGE('',*,*,#9695,.F.);
#14143=ORIENTED_EDGE('',*,*,#9696,.F.);
#14144=ORIENTED_EDGE('',*,*,#9690,.T.);
#14145=ORIENTED_EDGE('',*,*,#9697,.T.);
#14146=ORIENTED_EDGE('',*,*,#9698,.T.);
#14147=ORIENTED_EDGE('',*,*,#9699,.F.);
#14148=ORIENTED_EDGE('',*,*,#9700,.F.);
#14149=ORIENTED_EDGE('',*,*,#9694,.T.);
#14150=ORIENTED_EDGE('',*,*,#9701,.T.);
#14151=ORIENTED_EDGE('',*,*,#9702,.T.);
#14152=ORIENTED_EDGE('',*,*,#9703,.F.);
#14153=ORIENTED_EDGE('',*,*,#9704,.F.);
#14154=ORIENTED_EDGE('',*,*,#9705,.F.);
#14155=ORIENTED_EDGE('',*,*,#9699,.T.);
#14156=ORIENTED_EDGE('',*,*,#9706,.T.);
#14157=ORIENTED_EDGE('',*,*,#9707,.F.);
#14158=ORIENTED_EDGE('',*,*,#9708,.F.);
#14159=ORIENTED_EDGE('',*,*,#9703,.T.);
#14160=ORIENTED_EDGE('',*,*,#9709,.T.);
#14161=ORIENTED_EDGE('',*,*,#9710,.T.);
#14162=ORIENTED_EDGE('',*,*,#9711,.F.);
#14163=ORIENTED_EDGE('',*,*,#9712,.F.);
#14164=ORIENTED_EDGE('',*,*,#9713,.F.);
#14165=ORIENTED_EDGE('',*,*,#9707,.T.);
#14166=ORIENTED_EDGE('',*,*,#9714,.T.);
#14167=ORIENTED_EDGE('',*,*,#9715,.F.);
#14168=ORIENTED_EDGE('',*,*,#9716,.F.);
#14169=ORIENTED_EDGE('',*,*,#9711,.T.);
#14170=ORIENTED_EDGE('',*,*,#9717,.T.);
#14171=ORIENTED_EDGE('',*,*,#9718,.T.);
#14172=ORIENTED_EDGE('',*,*,#9719,.F.);
#14173=ORIENTED_EDGE('',*,*,#9720,.F.);
#14174=ORIENTED_EDGE('',*,*,#9721,.F.);
#14175=ORIENTED_EDGE('',*,*,#9715,.T.);
#14176=ORIENTED_EDGE('',*,*,#9722,.T.);
#14177=ORIENTED_EDGE('',*,*,#9723,.T.);
#14178=ORIENTED_EDGE('',*,*,#9724,.F.);
#14179=ORIENTED_EDGE('',*,*,#9725,.F.);
#14180=ORIENTED_EDGE('',*,*,#9719,.T.);
#14181=ORIENTED_EDGE('',*,*,#9726,.T.);
#14182=ORIENTED_EDGE('',*,*,#9727,.T.);
#14183=ORIENTED_EDGE('',*,*,#9728,.F.);
#14184=ORIENTED_EDGE('',*,*,#9729,.F.);
#14185=ORIENTED_EDGE('',*,*,#9730,.F.);
#14186=ORIENTED_EDGE('',*,*,#9724,.T.);
#14187=ORIENTED_EDGE('',*,*,#9731,.T.);
#14188=ORIENTED_EDGE('',*,*,#9732,.F.);
#14189=ORIENTED_EDGE('',*,*,#9733,.F.);
#14190=ORIENTED_EDGE('',*,*,#9728,.T.);
#14191=ORIENTED_EDGE('',*,*,#9734,.T.);
#14192=ORIENTED_EDGE('',*,*,#9735,.T.);
#14193=ORIENTED_EDGE('',*,*,#9736,.F.);
#14194=ORIENTED_EDGE('',*,*,#9737,.F.);
#14195=ORIENTED_EDGE('',*,*,#9738,.F.);
#14196=ORIENTED_EDGE('',*,*,#9732,.T.);
#14197=ORIENTED_EDGE('',*,*,#9739,.T.);
#14198=ORIENTED_EDGE('',*,*,#9740,.F.);
#14199=ORIENTED_EDGE('',*,*,#9741,.F.);
#14200=ORIENTED_EDGE('',*,*,#9736,.T.);
#14201=ORIENTED_EDGE('',*,*,#9742,.T.);
#14202=ORIENTED_EDGE('',*,*,#9743,.T.);
#14203=ORIENTED_EDGE('',*,*,#9744,.F.);
#14204=ORIENTED_EDGE('',*,*,#9745,.F.);
#14205=ORIENTED_EDGE('',*,*,#9746,.F.);
#14206=ORIENTED_EDGE('',*,*,#9740,.T.);
#14207=ORIENTED_EDGE('',*,*,#9747,.T.);
#14208=ORIENTED_EDGE('',*,*,#9748,.F.);
#14209=ORIENTED_EDGE('',*,*,#9749,.F.);
#14210=ORIENTED_EDGE('',*,*,#9744,.T.);
#14211=ORIENTED_EDGE('',*,*,#9750,.T.);
#14212=ORIENTED_EDGE('',*,*,#9751,.T.);
#14213=ORIENTED_EDGE('',*,*,#9752,.T.);
#14214=ORIENTED_EDGE('',*,*,#9753,.T.);
#14215=ORIENTED_EDGE('',*,*,#9754,.T.);
#14216=ORIENTED_EDGE('',*,*,#9755,.T.);
#14217=ORIENTED_EDGE('',*,*,#9756,.T.);
#14218=ORIENTED_EDGE('',*,*,#9757,.T.);
#14219=ORIENTED_EDGE('',*,*,#9758,.T.);
#14220=ORIENTED_EDGE('',*,*,#9759,.T.);
#14221=ORIENTED_EDGE('',*,*,#9760,.T.);
#14222=ORIENTED_EDGE('',*,*,#9761,.T.);
#14223=ORIENTED_EDGE('',*,*,#9762,.T.);
#14224=ORIENTED_EDGE('',*,*,#9763,.T.);
#14225=ORIENTED_EDGE('',*,*,#9764,.T.);
#14226=ORIENTED_EDGE('',*,*,#9765,.T.);
#14227=ORIENTED_EDGE('',*,*,#9766,.T.);
#14228=ORIENTED_EDGE('',*,*,#9767,.T.);
#14229=ORIENTED_EDGE('',*,*,#9768,.T.);
#14230=ORIENTED_EDGE('',*,*,#9769,.T.);
#14231=ORIENTED_EDGE('',*,*,#9770,.T.);
#14232=ORIENTED_EDGE('',*,*,#9771,.F.);
#14233=ORIENTED_EDGE('',*,*,#9772,.F.);
#14234=ORIENTED_EDGE('',*,*,#9773,.T.);
#14235=ORIENTED_EDGE('',*,*,#9774,.T.);
#14236=ORIENTED_EDGE('',*,*,#9775,.T.);
#14237=ORIENTED_EDGE('',*,*,#9776,.T.);
#14238=ORIENTED_EDGE('',*,*,#9777,.T.);
#14239=ORIENTED_EDGE('',*,*,#9778,.T.);
#14240=ORIENTED_EDGE('',*,*,#9779,.T.);
#14241=ORIENTED_EDGE('',*,*,#9780,.T.);
#14242=ORIENTED_EDGE('',*,*,#9781,.T.);
#14243=ORIENTED_EDGE('',*,*,#9782,.T.);
#14244=ORIENTED_EDGE('',*,*,#9783,.T.);
#14245=ORIENTED_EDGE('',*,*,#9784,.T.);
#14246=ORIENTED_EDGE('',*,*,#9785,.T.);
#14247=ORIENTED_EDGE('',*,*,#9786,.T.);
#14248=ORIENTED_EDGE('',*,*,#9787,.T.);
#14249=ORIENTED_EDGE('',*,*,#9748,.T.);
#14250=ORIENTED_EDGE('',*,*,#9788,.T.);
#14251=ORIENTED_EDGE('',*,*,#9789,.F.);
#14252=ORIENTED_EDGE('',*,*,#9790,.F.);
#14253=ORIENTED_EDGE('',*,*,#9791,.F.);
#14254=ORIENTED_EDGE('',*,*,#9792,.F.);
#14255=ORIENTED_EDGE('',*,*,#9793,.T.);
#14256=ORIENTED_EDGE('',*,*,#9789,.T.);
#14257=ORIENTED_EDGE('',*,*,#9794,.T.);
#14258=ORIENTED_EDGE('',*,*,#9795,.T.);
#14259=ORIENTED_EDGE('',*,*,#9793,.F.);
#14260=ORIENTED_EDGE('',*,*,#9796,.F.);
#14261=ORIENTED_EDGE('',*,*,#9770,.F.);
#14262=ORIENTED_EDGE('',*,*,#9769,.F.);
#14263=ORIENTED_EDGE('',*,*,#9768,.F.);
#14264=ORIENTED_EDGE('',*,*,#9767,.F.);
#14265=ORIENTED_EDGE('',*,*,#9766,.F.);
#14266=ORIENTED_EDGE('',*,*,#9765,.F.);
#14267=ORIENTED_EDGE('',*,*,#9764,.F.);
#14268=ORIENTED_EDGE('',*,*,#9763,.F.);
#14269=ORIENTED_EDGE('',*,*,#9762,.F.);
#14270=ORIENTED_EDGE('',*,*,#9761,.F.);
#14271=ORIENTED_EDGE('',*,*,#9760,.F.);
#14272=ORIENTED_EDGE('',*,*,#9759,.F.);
#14273=ORIENTED_EDGE('',*,*,#9758,.F.);
#14274=ORIENTED_EDGE('',*,*,#9757,.F.);
#14275=ORIENTED_EDGE('',*,*,#9756,.F.);
#14276=ORIENTED_EDGE('',*,*,#9755,.F.);
#14277=ORIENTED_EDGE('',*,*,#9754,.F.);
#14278=ORIENTED_EDGE('',*,*,#9797,.F.);
#14279=ORIENTED_EDGE('',*,*,#9691,.T.);
#14280=ORIENTED_EDGE('',*,*,#9696,.T.);
#14281=ORIENTED_EDGE('',*,*,#9695,.T.);
#14282=ORIENTED_EDGE('',*,*,#9700,.T.);
#14283=ORIENTED_EDGE('',*,*,#9705,.T.);
#14284=ORIENTED_EDGE('',*,*,#9704,.T.);
#14285=ORIENTED_EDGE('',*,*,#9708,.T.);
#14286=ORIENTED_EDGE('',*,*,#9713,.T.);
#14287=ORIENTED_EDGE('',*,*,#9712,.T.);
#14288=ORIENTED_EDGE('',*,*,#9716,.T.);
#14289=ORIENTED_EDGE('',*,*,#9721,.T.);
#14290=ORIENTED_EDGE('',*,*,#9720,.T.);
#14291=ORIENTED_EDGE('',*,*,#9725,.T.);
#14292=ORIENTED_EDGE('',*,*,#9730,.T.);
#14293=ORIENTED_EDGE('',*,*,#9729,.T.);
#14294=ORIENTED_EDGE('',*,*,#9733,.T.);
#14295=ORIENTED_EDGE('',*,*,#9738,.T.);
#14296=ORIENTED_EDGE('',*,*,#9737,.T.);
#14297=ORIENTED_EDGE('',*,*,#9741,.T.);
#14298=ORIENTED_EDGE('',*,*,#9746,.T.);
#14299=ORIENTED_EDGE('',*,*,#9745,.T.);
#14300=ORIENTED_EDGE('',*,*,#9749,.T.);
#14301=ORIENTED_EDGE('',*,*,#9791,.T.);
#14302=ORIENTED_EDGE('',*,*,#9790,.T.);
#14303=ORIENTED_EDGE('',*,*,#9798,.T.);
#14304=ORIENTED_EDGE('',*,*,#9799,.T.);
#14305=ORIENTED_EDGE('',*,*,#9800,.T.);
#14306=ORIENTED_EDGE('',*,*,#9692,.T.);
#14307=ORIENTED_EDGE('',*,*,#9797,.T.);
#14308=ORIENTED_EDGE('',*,*,#9795,.F.);
#14309=ORIENTED_EDGE('',*,*,#9794,.F.);
#14310=ORIENTED_EDGE('',*,*,#9788,.F.);
#14311=ORIENTED_EDGE('',*,*,#9751,.F.);
#14312=ORIENTED_EDGE('',*,*,#9750,.F.);
#14313=ORIENTED_EDGE('',*,*,#9747,.F.);
#14314=ORIENTED_EDGE('',*,*,#9743,.F.);
#14315=ORIENTED_EDGE('',*,*,#9742,.F.);
#14316=ORIENTED_EDGE('',*,*,#9739,.F.);
#14317=ORIENTED_EDGE('',*,*,#9735,.F.);
#14318=ORIENTED_EDGE('',*,*,#9734,.F.);
#14319=ORIENTED_EDGE('',*,*,#9731,.F.);
#14320=ORIENTED_EDGE('',*,*,#9727,.F.);
#14321=ORIENTED_EDGE('',*,*,#9726,.F.);
#14322=ORIENTED_EDGE('',*,*,#9723,.F.);
#14323=ORIENTED_EDGE('',*,*,#9722,.F.);
#14324=ORIENTED_EDGE('',*,*,#9718,.F.);
#14325=ORIENTED_EDGE('',*,*,#9717,.F.);
#14326=ORIENTED_EDGE('',*,*,#9714,.F.);
#14327=ORIENTED_EDGE('',*,*,#9710,.F.);
#14328=ORIENTED_EDGE('',*,*,#9709,.F.);
#14329=ORIENTED_EDGE('',*,*,#9706,.F.);
#14330=ORIENTED_EDGE('',*,*,#9702,.F.);
#14331=ORIENTED_EDGE('',*,*,#9701,.F.);
#14332=ORIENTED_EDGE('',*,*,#9698,.F.);
#14333=ORIENTED_EDGE('',*,*,#9697,.F.);
#14334=ORIENTED_EDGE('',*,*,#9693,.F.);
#14335=ORIENTED_EDGE('',*,*,#9800,.F.);
#14336=ORIENTED_EDGE('',*,*,#9801,.T.);
#14337=ORIENTED_EDGE('',*,*,#9752,.F.);
#14338=ORIENTED_EDGE('',*,*,#9787,.F.);
#14339=ORIENTED_EDGE('',*,*,#9786,.F.);
#14340=ORIENTED_EDGE('',*,*,#9785,.F.);
#14341=ORIENTED_EDGE('',*,*,#9784,.F.);
#14342=ORIENTED_EDGE('',*,*,#9783,.F.);
#14343=ORIENTED_EDGE('',*,*,#9782,.F.);
#14344=ORIENTED_EDGE('',*,*,#9781,.F.);
#14345=ORIENTED_EDGE('',*,*,#9780,.F.);
#14346=ORIENTED_EDGE('',*,*,#9779,.F.);
#14347=ORIENTED_EDGE('',*,*,#9778,.F.);
#14348=ORIENTED_EDGE('',*,*,#9777,.F.);
#14349=ORIENTED_EDGE('',*,*,#9776,.F.);
#14350=ORIENTED_EDGE('',*,*,#9775,.F.);
#14351=ORIENTED_EDGE('',*,*,#9774,.F.);
#14352=ORIENTED_EDGE('',*,*,#9773,.F.);
#14353=ORIENTED_EDGE('',*,*,#9802,.T.);
#14354=ORIENTED_EDGE('',*,*,#9803,.T.);
#14355=ORIENTED_EDGE('',*,*,#9771,.T.);
#14356=ORIENTED_EDGE('',*,*,#9796,.T.);
#14357=ORIENTED_EDGE('',*,*,#9792,.T.);
#14358=ORIENTED_EDGE('',*,*,#9772,.T.);
#14359=ORIENTED_EDGE('',*,*,#9803,.F.);
#14360=ORIENTED_EDGE('',*,*,#9804,.F.);
#14361=ORIENTED_EDGE('',*,*,#9802,.F.);
#14362=ORIENTED_EDGE('',*,*,#9805,.F.);
#14363=ORIENTED_EDGE('',*,*,#9806,.F.);
#14364=ORIENTED_EDGE('',*,*,#9807,.F.);
#14365=ORIENTED_EDGE('',*,*,#9808,.F.);
#14366=ORIENTED_EDGE('',*,*,#9809,.F.);
#14367=ORIENTED_EDGE('',*,*,#9810,.F.);
#14368=ORIENTED_EDGE('',*,*,#9811,.F.);
#14369=ORIENTED_EDGE('',*,*,#9812,.T.);
#14370=ORIENTED_EDGE('',*,*,#9813,.F.);
#14371=ORIENTED_EDGE('',*,*,#9812,.F.);
#14372=ORIENTED_EDGE('',*,*,#9810,.T.);
#14373=ORIENTED_EDGE('',*,*,#9814,.T.);
#14374=ORIENTED_EDGE('',*,*,#9815,.T.);
#14375=ORIENTED_EDGE('',*,*,#9816,.F.);
#14376=ORIENTED_EDGE('',*,*,#9809,.T.);
#14377=ORIENTED_EDGE('',*,*,#9817,.T.);
#14378=ORIENTED_EDGE('',*,*,#9818,.T.);
#14379=ORIENTED_EDGE('',*,*,#9814,.F.);
#14380=ORIENTED_EDGE('',*,*,#9808,.T.);
#14381=ORIENTED_EDGE('',*,*,#9819,.T.);
#14382=ORIENTED_EDGE('',*,*,#9820,.T.);
#14383=ORIENTED_EDGE('',*,*,#9817,.F.);
#14384=ORIENTED_EDGE('',*,*,#9821,.T.);
#14385=ORIENTED_EDGE('',*,*,#9822,.F.);
#14386=ORIENTED_EDGE('',*,*,#9821,.F.);
#14387=ORIENTED_EDGE('',*,*,#9807,.T.);
#14388=ORIENTED_EDGE('',*,*,#9823,.T.);
#14389=ORIENTED_EDGE('',*,*,#9824,.T.);
#14390=ORIENTED_EDGE('',*,*,#9819,.F.);
#14391=ORIENTED_EDGE('',*,*,#9806,.T.);
#14392=ORIENTED_EDGE('',*,*,#9825,.T.);
#14393=ORIENTED_EDGE('',*,*,#9826,.T.);
#14394=ORIENTED_EDGE('',*,*,#9823,.F.);
#14395=ORIENTED_EDGE('',*,*,#9805,.T.);
#14396=ORIENTED_EDGE('',*,*,#9811,.T.);
#14397=ORIENTED_EDGE('',*,*,#9816,.T.);
#14398=ORIENTED_EDGE('',*,*,#9827,.T.);
#14399=ORIENTED_EDGE('',*,*,#9825,.F.);
#14400=ORIENTED_EDGE('',*,*,#9820,.F.);
#14401=ORIENTED_EDGE('',*,*,#9824,.F.);
#14402=ORIENTED_EDGE('',*,*,#9826,.F.);
#14403=ORIENTED_EDGE('',*,*,#9827,.F.);
#14404=ORIENTED_EDGE('',*,*,#9815,.F.);
#14405=ORIENTED_EDGE('',*,*,#9818,.F.);
#14406=ORIENTED_EDGE('',*,*,#9822,.T.);
#14407=ORIENTED_EDGE('',*,*,#9828,.T.);
#14408=ORIENTED_EDGE('',*,*,#9829,.T.);
#14409=ORIENTED_EDGE('',*,*,#9830,.T.);
#14410=ORIENTED_EDGE('',*,*,#9829,.F.);
#14411=ORIENTED_EDGE('',*,*,#9830,.F.);
#14412=ORIENTED_EDGE('',*,*,#9831,.T.);
#14413=ORIENTED_EDGE('',*,*,#9832,.T.);
#14414=ORIENTED_EDGE('',*,*,#9831,.F.);
#14415=ORIENTED_EDGE('',*,*,#9828,.F.);
#14416=ORIENTED_EDGE('',*,*,#9813,.T.);
#14417=ORIENTED_EDGE('',*,*,#9833,.F.);
#14418=ORIENTED_EDGE('',*,*,#9801,.F.);
#14419=ORIENTED_EDGE('',*,*,#9799,.F.);
#14420=ORIENTED_EDGE('',*,*,#9834,.T.);
#14421=ORIENTED_EDGE('',*,*,#9833,.T.);
#14422=ORIENTED_EDGE('',*,*,#9834,.F.);
#14423=ORIENTED_EDGE('',*,*,#9798,.F.);
#14424=ORIENTED_EDGE('',*,*,#9753,.F.);
#14425=ORIENTED_EDGE('',*,*,#9832,.F.);
#14426=ORIENTED_EDGE('',*,*,#9835,.T.);
#14427=ORIENTED_EDGE('',*,*,#9804,.T.);
#14428=ORIENTED_EDGE('',*,*,#9835,.F.);
#14725=PLANE('',#17205);
#14726=PLANE('',#17207);
#14727=PLANE('',#17213);
#14728=PLANE('',#17217);
#14729=PLANE('',#17218);
#14730=PLANE('',#17219);
#14731=PLANE('',#17222);
#14732=PLANE('',#17223);
#14733=PLANE('',#17224);
#14734=PLANE('',#17225);
#14735=PLANE('',#17232);
#14736=PLANE('',#17233);
#15565=ADVANCED_FACE('',(#3209),#1581,.T.);
#15566=ADVANCED_FACE('',(#3210),#1582,.T.);
#15567=ADVANCED_FACE('',(#3211),#1583,.T.);
#15568=ADVANCED_FACE('',(#3212),#1584,.T.);
#15569=ADVANCED_FACE('',(#3213),#1585,.T.);
#15570=ADVANCED_FACE('',(#3214),#1586,.T.);
#15571=ADVANCED_FACE('',(#3215),#1587,.T.);
#15572=ADVANCED_FACE('',(#3216),#1588,.T.);
#15573=ADVANCED_FACE('',(#3217),#1589,.T.);
#15574=ADVANCED_FACE('',(#3218),#1590,.T.);
#15575=ADVANCED_FACE('',(#3219),#1591,.T.);
#15576=ADVANCED_FACE('',(#3220),#1592,.T.);
#15577=ADVANCED_FACE('',(#3221),#1593,.T.);
#15578=ADVANCED_FACE('',(#3222),#1594,.T.);
#15579=ADVANCED_FACE('',(#3223),#1595,.T.);
#15580=ADVANCED_FACE('',(#3224),#1596,.T.);
#15581=ADVANCED_FACE('',(#3225),#1597,.T.);
#15582=ADVANCED_FACE('',(#3226),#14725,.F.);
#15583=ADVANCED_FACE('',(#3227),#258,.F.);
#15584=ADVANCED_FACE('',(#3228),#14726,.T.);
#15585=ADVANCED_FACE('',(#3229),#259,.F.);
#15586=ADVANCED_FACE('',(#3230),#159,.F.);
#15587=ADVANCED_FACE('',(#3231,#1749),#14727,.T.);
#15588=ADVANCED_FACE('',(#3232),#1344,.F.);
#15589=ADVANCED_FACE('',(#3233),#14728,.F.);
#15590=ADVANCED_FACE('',(#3234),#14729,.F.);
#15591=ADVANCED_FACE('',(#3235),#14730,.F.);
#15592=ADVANCED_FACE('',(#3236),#1345,.F.);
#15593=ADVANCED_FACE('',(#3237),#14731,.F.);
#15594=ADVANCED_FACE('',(#3238),#14732,.F.);
#15595=ADVANCED_FACE('',(#3239),#14733,.F.);
#15596=ADVANCED_FACE('',(#3240,#1750),#14734,.F.);
#15597=ADVANCED_FACE('',(#3241),#160,.T.);
#15598=ADVANCED_FACE('',(#3242),#1598,.T.);
#15599=ADVANCED_FACE('',(#3243,#1751),#14735,.T.);
#15600=ADVANCED_FACE('',(#3244),#14736,.T.);
#15601=ADVANCED_FACE('',(#3245),#1346,.T.);
#15602=ADVANCED_FACE('',(#3246),#1347,.T.);
#15629=CLOSED_SHELL('',(#15565,#15566,#15567,#15568,#15569,#15570,#15571,
#15572,#15573,#15574,#15575,#15576,#15577,#15578,#15579,#15580,#15581,#15582,
#15583,#15584,#15585,#15586,#15587,#15588,#15589,#15590,#15591,#15592,#15593,
#15594,#15595,#15596,#15597,#15598,#15599,#15600,#15601,#15602));
#17181=AXIS2_PLACEMENT_3D('',#77446,#20810,#20811);
#17182=AXIS2_PLACEMENT_3D('',#77447,#20812,#20813);
#17183=AXIS2_PLACEMENT_3D('',#77529,#20815,#20816);
#17184=AXIS2_PLACEMENT_3D('',#77579,#20817,#20818);
#17185=AXIS2_PLACEMENT_3D('',#77808,#20820,#20821);
#17186=AXIS2_PLACEMENT_3D('',#78180,#20823,#20824);
#17187=AXIS2_PLACEMENT_3D('',#78591,#20826,#20827);
#17188=AXIS2_PLACEMENT_3D('',#79040,#20829,#20830);
#17189=AXIS2_PLACEMENT_3D('',#79447,#20832,#20833);
#17190=AXIS2_PLACEMENT_3D('',#79776,#20835,#20836);
#17191=AXIS2_PLACEMENT_3D('',#80051,#20838,#20839);
#17192=AXIS2_PLACEMENT_3D('',#80414,#20841,#20842);
#17193=AXIS2_PLACEMENT_3D('',#80821,#20844,#20845);
#17194=AXIS2_PLACEMENT_3D('',#81236,#20847,#20848);
#17195=AXIS2_PLACEMENT_3D('',#81635,#20850,#20851);
#17196=AXIS2_PLACEMENT_3D('',#82032,#20853,#20854);
#17197=AXIS2_PLACEMENT_3D('',#82437,#20856,#20857);
#17198=AXIS2_PLACEMENT_3D('',#82852,#20859,#20860);
#17199=AXIS2_PLACEMENT_3D('',#82862,#20861,#20862);
#17200=AXIS2_PLACEMENT_3D('',#83895,#20863,#20864);
#17201=AXIS2_PLACEMENT_3D('',#83897,#20865,#20866);
#17202=AXIS2_PLACEMENT_3D('',#83899,#20867,#20868);
#17203=AXIS2_PLACEMENT_3D('',#84920,#20869,#20870);
#17204=AXIS2_PLACEMENT_3D('',#85083,#20871,#20872);
#17205=AXIS2_PLACEMENT_3D('',#85178,#20873,#20874);
#17206=AXIS2_PLACEMENT_3D('',#85180,#20875,#20876);
#17207=AXIS2_PLACEMENT_3D('',#85768,#20877,#20878);
#17208=AXIS2_PLACEMENT_3D('',#85770,#20879,#20880);
#17209=AXIS2_PLACEMENT_3D('',#85772,#20881,#20882);
#17210=AXIS2_PLACEMENT_3D('',#86239,#20883,#20884);
#17211=AXIS2_PLACEMENT_3D('',#86241,#20885,#20886);
#17212=AXIS2_PLACEMENT_3D('',#86242,#20887,#20888);
#17213=AXIS2_PLACEMENT_3D('',#86243,#20889,#20890);
#17214=AXIS2_PLACEMENT_3D('',#86245,#20891,#20892);
#17215=AXIS2_PLACEMENT_3D('',#86246,#20893,#20894);
#17216=AXIS2_PLACEMENT_3D('',#86277,#20896,#20897);
#17217=AXIS2_PLACEMENT_3D('',#86278,#20898,#20899);
#17218=AXIS2_PLACEMENT_3D('',#86284,#20903,#20904);
#17219=AXIS2_PLACEMENT_3D('',#86288,#20907,#20908);
#17220=AXIS2_PLACEMENT_3D('',#86292,#20911,#20912);
#17221=AXIS2_PLACEMENT_3D('',#86296,#20914,#20915);
#17222=AXIS2_PLACEMENT_3D('',#86297,#20916,#20917);
#17223=AXIS2_PLACEMENT_3D('',#86301,#20920,#20921);
#17224=AXIS2_PLACEMENT_3D('',#86305,#20924,#20925);
#17225=AXIS2_PLACEMENT_3D('',#86307,#20927,#20928);
#17226=AXIS2_PLACEMENT_3D('',#86308,#20929,#20930);
#17227=AXIS2_PLACEMENT_3D('',#86310,#20931,#20932);
#17228=AXIS2_PLACEMENT_3D('',#86312,#20933,#20934);
#17229=AXIS2_PLACEMENT_3D('',#86313,#20935,#20936);
#17230=AXIS2_PLACEMENT_3D('',#86314,#20937,#20938);
#17231=AXIS2_PLACEMENT_3D('',#86317,#20940,#20941);
#17232=AXIS2_PLACEMENT_3D('',#86318,#20942,#20943);
#17233=AXIS2_PLACEMENT_3D('',#86319,#20944,#20945);
#17234=AXIS2_PLACEMENT_3D('',#86321,#20946,#20947);
#17235=AXIS2_PLACEMENT_3D('',#86322,#20948,#20949);
#17236=AXIS2_PLACEMENT_3D('',#86324,#20951,#20952);
#20810=DIRECTION('axis',(0.,0.,1.));
#20811=DIRECTION('refdir',(1.,0.,0.));
#20812=DIRECTION('center_axis',(0.,0.,1.));
#20813=DIRECTION('ref_axis',(0.17681385355385,-0.984244309707421,0.));
#20814=DIRECTION('',(0.,0.,-1.));
#20815=DIRECTION('center_axis',(0.,0.,-1.));
#20816=DIRECTION('ref_axis',(1.,9.72557910080329E-14,0.));
#20817=DIRECTION('center_axis',(0.,0.,1.));
#20818=DIRECTION('ref_axis',(0.17681385355385,-0.984244309707421,0.));
#20819=DIRECTION('',(0.,0.,-1.));
#20820=DIRECTION('center_axis',(0.,0.,1.));
#20821=DIRECTION('ref_axis',(0.17681385355385,-0.984244309707421,0.));
#20822=DIRECTION('',(0.,0.,-1.));
#20823=DIRECTION('center_axis',(0.,0.,1.));
#20824=DIRECTION('ref_axis',(0.17681385355385,-0.984244309707421,0.));
#20825=DIRECTION('',(0.,0.,-1.));
#20826=DIRECTION('center_axis',(0.,0.,1.));
#20827=DIRECTION('ref_axis',(0.17681385355385,-0.984244309707421,0.));
#20828=DIRECTION('',(0.,0.,-1.));
#20829=DIRECTION('center_axis',(0.,0.,1.));
#20830=DIRECTION('ref_axis',(0.17681385355385,-0.984244309707421,0.));
#20831=DIRECTION('',(0.,0.,-1.));
#20832=DIRECTION('center_axis',(0.,0.,1.));
#20833=DIRECTION('ref_axis',(0.17681385355385,-0.984244309707421,0.));
#20834=DIRECTION('',(0.,0.,-1.));
#20835=DIRECTION('center_axis',(0.,0.,1.));
#20836=DIRECTION('ref_axis',(0.17681385355385,-0.984244309707421,0.));
#20837=DIRECTION('',(0.,0.,-1.));
#20838=DIRECTION('center_axis',(0.,0.,1.));
#20839=DIRECTION('ref_axis',(0.17681385355385,-0.984244309707421,0.));
#20840=DIRECTION('',(0.,0.,-1.));
#20841=DIRECTION('center_axis',(0.,0.,1.));
#20842=DIRECTION('ref_axis',(0.17681385355385,-0.984244309707421,0.));
#20843=DIRECTION('',(0.,0.,-1.));
#20844=DIRECTION('center_axis',(0.,0.,1.));
#20845=DIRECTION('ref_axis',(0.17681385355385,-0.984244309707421,0.));
#20846=DIRECTION('',(0.,0.,-1.));
#20847=DIRECTION('center_axis',(0.,0.,1.));
#20848=DIRECTION('ref_axis',(0.17681385355385,-0.984244309707421,0.));
#20849=DIRECTION('',(0.,0.,-1.));
#20850=DIRECTION('center_axis',(0.,0.,1.));
#20851=DIRECTION('ref_axis',(0.17681385355385,-0.984244309707421,0.));
#20852=DIRECTION('',(0.,0.,-1.));
#20853=DIRECTION('center_axis',(0.,0.,1.));
#20854=DIRECTION('ref_axis',(0.17681385355385,-0.984244309707421,0.));
#20855=DIRECTION('',(0.,0.,-1.));
#20856=DIRECTION('center_axis',(0.,0.,1.));
#20857=DIRECTION('ref_axis',(0.17681385355385,-0.984244309707421,0.));
#20858=DIRECTION('',(0.,0.,-1.));
#20859=DIRECTION('center_axis',(0.,0.,1.));
#20860=DIRECTION('ref_axis',(1.,0.,0.));
#20861=DIRECTION('center_axis',(0.,0.,1.));
#20862=DIRECTION('ref_axis',(1.,0.,0.));
#20863=DIRECTION('center_axis',(-0.00688311457455106,0.0538278304439539,
0.998526508112554));
#20864=DIRECTION('ref_axis',(-0.982071861916797,-0.188476423288724,0.00339055977177));
#20865=DIRECTION('center_axis',(0.,0.,1.));
#20866=DIRECTION('ref_axis',(1.,0.,0.));
#20867=DIRECTION('center_axis',(0.,0.,1.));
#20868=DIRECTION('ref_axis',(1.,0.,0.));
#20869=DIRECTION('center_axis',(0.,0.,1.));
#20870=DIRECTION('ref_axis',(-0.501290049117399,-0.865279311353205,0.));
#20871=DIRECTION('center_axis',(0.,0.,1.));
#20872=DIRECTION('ref_axis',(1.,9.72557910080329E-14,0.));
#20873=DIRECTION('center_axis',(0.,0.,1.));
#20874=DIRECTION('ref_axis',(1.,0.,0.));
#20875=DIRECTION('center_axis',(0.,0.,1.));
#20876=DIRECTION('ref_axis',(1.,0.,0.));
#20877=DIRECTION('center_axis',(0.,0.,1.));
#20878=DIRECTION('ref_axis',(1.,0.,0.));
#20879=DIRECTION('center_axis',(0.,0.,1.));
#20880=DIRECTION('ref_axis',(1.,0.,0.));
#20881=DIRECTION('center_axis',(0.,0.,1.));
#20882=DIRECTION('ref_axis',(1.,0.,0.));
#20883=DIRECTION('center_axis',(0.,0.,1.));
#20884=DIRECTION('ref_axis',(1.,0.,0.));
#20885=DIRECTION('center_axis',(0.,0.,-1.));
#20886=DIRECTION('ref_axis',(1.,0.,0.));
#20887=DIRECTION('center_axis',(-1.22464679914735E-16,1.,0.));
#20888=DIRECTION('ref_axis',(-1.,-1.22464679914735E-16,0.));
#20889=DIRECTION('center_axis',(0.,0.,-1.));
#20890=DIRECTION('ref_axis',(-1.,0.,0.));
#20891=DIRECTION('center_axis',(0.,0.,1.));
#20892=DIRECTION('ref_axis',(1.,0.,0.));
#20893=DIRECTION('center_axis',(0.,0.,1.));
#20894=DIRECTION('ref_axis',(1.,0.,0.));
#20895=DIRECTION('',(-0.86602540378444,-1.06057523872491E-16,0.499999999999998));
#20896=DIRECTION('center_axis',(0.,0.,-1.));
#20897=DIRECTION('ref_axis',(1.,0.,0.));
#20898=DIRECTION('center_axis',(-0.5,-0.866025403784439,0.));
#20899=DIRECTION('ref_axis',(-0.866025403784439,0.5,0.));
#20900=DIRECTION('',(0.,0.,-1.));
#20901=DIRECTION('',(-0.866025403784439,0.5,0.));
#20902=DIRECTION('',(0.,0.,-1.));
#20903=DIRECTION('center_axis',(0.5,-0.866025403784439,0.));
#20904=DIRECTION('ref_axis',(-0.866025403784439,-0.5,0.));
#20905=DIRECTION('',(0.,0.,-1.));
#20906=DIRECTION('',(-0.866025403784439,-0.5,0.));
#20907=DIRECTION('center_axis',(1.,-3.84592537276713E-16,0.));
#20908=DIRECTION('ref_axis',(-3.84592537276713E-16,-1.,0.));
#20909=DIRECTION('',(0.,0.,-1.));
#20910=DIRECTION('',(-3.84592537276713E-16,-1.,0.));
#20911=DIRECTION('center_axis',(0.,0.,1.));
#20912=DIRECTION('ref_axis',(1.,0.,0.));
#20913=DIRECTION('',(-0.855621686410732,-1.04783435954396E-16,0.517601709564076));
#20914=DIRECTION('center_axis',(0.,0.,-1.));
#20915=DIRECTION('ref_axis',(1.,0.,0.));
#20916=DIRECTION('center_axis',(0.5,0.866025403784439,0.));
#20917=DIRECTION('ref_axis',(0.866025403784439,-0.5,0.));
#20918=DIRECTION('',(0.,0.,-1.));
#20919=DIRECTION('',(0.866025403784439,-0.5,0.));
#20920=DIRECTION('center_axis',(-0.5,0.866025403784439,0.));
#20921=DIRECTION('ref_axis',(0.866025403784439,0.5,0.));
#20922=DIRECTION('',(0.,0.,-1.));
#20923=DIRECTION('',(0.866025403784439,0.5,0.));
#20924=DIRECTION('center_axis',(-1.,-1.92296268638356E-16,0.));
#20925=DIRECTION('ref_axis',(-1.92296268638356E-16,1.,0.));
#20926=DIRECTION('',(-1.92296268638356E-16,1.,0.));
#20927=DIRECTION('center_axis',(0.,0.,-1.));
#20928=DIRECTION('ref_axis',(-1.,0.,0.));
#20929=DIRECTION('center_axis',(0.,0.,1.));
#20930=DIRECTION('ref_axis',(1.,0.,0.));
#20931=DIRECTION('center_axis',(0.,0.,-1.));
#20932=DIRECTION('ref_axis',(-1.,1.22464679914735E-16,0.));
#20933=DIRECTION('center_axis',(1.22464679914735E-16,-1.,0.));
#20934=DIRECTION('ref_axis',(-1.,-1.22464679914735E-16,0.));
#20935=DIRECTION('center_axis',(0.,0.,1.));
#20936=DIRECTION('ref_axis',(-1.,1.22464679914735E-16,0.));
#20937=DIRECTION('center_axis',(0.,0.,1.));
#20938=DIRECTION('ref_axis',(1.,0.,0.));
#20939=DIRECTION('',(0.,0.,-1.));
#20940=DIRECTION('center_axis',(0.,0.,1.));
#20941=DIRECTION('ref_axis',(1.,0.,0.));
#20942=DIRECTION('center_axis',(0.,0.,1.));
#20943=DIRECTION('ref_axis',(1.,0.,0.));
#20944=DIRECTION('center_axis',(0.,0.,-1.));
#20945=DIRECTION('ref_axis',(-1.,0.,0.));
#20946=DIRECTION('center_axis',(0.,0.,1.));
#20947=DIRECTION('ref_axis',(1.,0.,0.));
#20948=DIRECTION('center_axis',(0.,0.,1.));
#20949=DIRECTION('ref_axis',(1.,0.,0.));
#20950=DIRECTION('',(0.707106781186548,8.65956056235494E-17,-0.707106781186547));
#20951=DIRECTION('center_axis',(0.,0.,1.));
#20952=DIRECTION('ref_axis',(1.,0.,0.));
#20953=DIRECTION('',(0.707106781186548,8.65956056235494E-17,-0.707106781186547));
#77446=CARTESIAN_POINT('',(0.,0.,0.));
#77447=CARTESIAN_POINT('Origin',(0.,0.,-1.7456589891905));
#77448=CARTESIAN_POINT('',(-0.0419358257166342,0.233438144154858,-1.49810946104348));
#77449=CARTESIAN_POINT('',(-0.0419358257166344,0.233438144154858,-1.51783893213918));
#77450=CARTESIAN_POINT('',(-0.0419358257166344,0.233438144154858,-1.7456589891905));
#77451=CARTESIAN_POINT('',(-0.137697638232154,-0.193109660686064,-1.56079343935569));
#77452=CARTESIAN_POINT('Ctrl Pts',(-0.137697638232154,-0.193109660686064,
-1.56079343935569));
#77453=CARTESIAN_POINT('Ctrl Pts',(-0.126370765437366,-0.201186333944446,
-1.55985488745099));
#77454=CARTESIAN_POINT('Ctrl Pts',(-0.114290892516889,-0.208291353281666,
-1.5589163355463));
#77455=CARTESIAN_POINT('Ctrl Pts',(-0.101651101434149,-0.214287270275731,
-1.5579777836416));
#77456=CARTESIAN_POINT('Ctrl Pts',(-0.0883887572017104,-0.220578506787781,
-1.5569930048301));
#77457=CARTESIAN_POINT('Ctrl Pts',(-0.0745105783197592,-0.225647730152209,
-1.5560082260186));
#77458=CARTESIAN_POINT('Ctrl Pts',(-0.0602716607461343,-0.229388987390203,
-1.5550234472071));
#77459=CARTESIAN_POINT('Ctrl Pts',(-0.0467279065913889,-0.232947591335977,
-1.55408674664325));
#77460=CARTESIAN_POINT('Ctrl Pts',(-0.0328587864043571,-0.235304889593483,
-1.5531500460794));
#77461=CARTESIAN_POINT('Ctrl Pts',(-0.0188993798127954,-0.236420798720611,
-1.55221334551556));
#77462=CARTESIAN_POINT('Ctrl Pts',(-0.00493879338562826,-0.237536802163304,
-1.55127656578268));
#77463=CARTESIAN_POINT('Ctrl Pts',(0.00911124316326098,-0.23741117478722,
-1.5503397860498));
#77464=CARTESIAN_POINT('Ctrl Pts',(0.0230131566390361,-0.236055873145548,
-1.54940300631693));
#77465=CARTESIAN_POINT('Ctrl Pts',(0.0369446089546456,-0.234697691753676,
-1.54846423611083));
#77466=CARTESIAN_POINT('Ctrl Pts',(0.0507264729274663,-0.232104781046902,
-1.54752546590473));
#77467=CARTESIAN_POINT('Ctrl Pts',(0.064129947202506,-0.228340382974199,
-1.54658669569864));
#77468=CARTESIAN_POINT('Ctrl Pts',(0.0661586067379395,-0.227770629051548,
-1.54644460976695));
#77469=CARTESIAN_POINT('Ctrl Pts',(0.0681786309103138,-0.227174130570319,
-1.54630252383527));
#77470=CARTESIAN_POINT('Ctrl Pts',(0.0701892650732185,-0.226551203248805,
-1.54616043790358));
#77471=CARTESIAN_POINT('Ctrl Pts',(0.0836284579295186,-0.22238752167822,
-1.54521072747226));
#77472=CARTESIAN_POINT('Ctrl Pts',(0.0967391885512409,-0.217010454215219,
-1.54426101704094));
#77473=CARTESIAN_POINT('Ctrl Pts',(0.10929121432994,-0.21049325665039,-1.54331130660963));
#77474=CARTESIAN_POINT('Ctrl Pts',(0.121818655152384,-0.203988823958728,
-1.54236345632342));
#77475=CARTESIAN_POINT('Ctrl Pts',(0.133788802529112,-0.196349013696355,
-1.54141560603721));
#77476=CARTESIAN_POINT('Ctrl Pts',(0.144991705523557,-0.187694927886638,
-1.54046775575101));
#77477=CARTESIAN_POINT('Ctrl Pts',(0.156193459843084,-0.179041729412223,
-1.53952000265138));
#77478=CARTESIAN_POINT('Ctrl Pts',(0.166627440775333,-0.169374931443179,
-1.53857224955176));
#77479=CARTESIAN_POINT('Ctrl Pts',(0.176113728514314,-0.158858223752459,
-1.53762449645214));
#77480=CARTESIAN_POINT('Ctrl Pts',(0.185598801175167,-0.148342863124136,
-1.53667686474816));
#77481=CARTESIAN_POINT('Ctrl Pts',(0.194135879692125,-0.136978439371701,
-1.53572923304419));
#77482=CARTESIAN_POINT('Ctrl Pts',(0.201584340829336,-0.124962931133204,
-1.53478160134021));
#77483=CARTESIAN_POINT('Ctrl Pts',(0.209050214271248,-0.112919334181251,
-1.53383175435288));
#77484=CARTESIAN_POINT('Ctrl Pts',(0.215421989731213,-0.100222345577201,
-1.53288190736556));
#77485=CARTESIAN_POINT('Ctrl Pts',(0.220604506107634,-0.0870955366824668,
-1.53193206037823));
#77486=CARTESIAN_POINT('Ctrl Pts',(0.223561640495988,-0.0796054034783375,
-1.53139007942035));
#77487=CARTESIAN_POINT('Ctrl Pts',(0.226132462018965,-0.0719757125191499,
-1.53084809846247));
#77488=CARTESIAN_POINT('Ctrl Pts',(0.22830661995882,-0.0642500420854265,
-1.5303061175046));
#77489=CARTESIAN_POINT('Ctrl Pts',(0.2321046350015,-0.0507541446696043,
-1.52935933631951));
#77490=CARTESIAN_POINT('Ctrl Pts',(0.23471489071116,-0.0368738355829154,
-1.52841255513442));
#77491=CARTESIAN_POINT('Ctrl Pts',(0.236072645345789,-0.0228404628771269,
-1.52746577394934));
#77492=CARTESIAN_POINT('Ctrl Pts',(0.237427618165454,-0.00883584223389452,
-1.5265209325625));
#77493=CARTESIAN_POINT('Ctrl Pts',(0.237535031407606,0.00532040275172917,
-1.52557609117567));
#77494=CARTESIAN_POINT('Ctrl Pts',(0.236381263236701,0.0193875995322088,
-1.52463124978883));
#77495=CARTESIAN_POINT('Ctrl Pts',(0.235227703772985,0.0334522516722969,
-1.52368657931605));
#77496=CARTESIAN_POINT('Ctrl Pts',(0.232813433502387,0.047427051266188,
-1.52274190884326));
#77497=CARTESIAN_POINT('Ctrl Pts',(0.229176908063932,0.0610731154867347,
-1.52179723837048));
#77498=CARTESIAN_POINT('Ctrl Pts',(0.225541026574461,0.074716763288276,
-1.52085273517814));
#77499=CARTESIAN_POINT('Ctrl Pts',(0.220683552684347,0.0880309870194809,
-1.51990823198579));
#77500=CARTESIAN_POINT('Ctrl Pts',(0.214693137571915,0.100791057661516,
-1.51896372879345));
#77501=CARTESIAN_POINT('Ctrl Pts',(0.208688739205051,0.113580913771001,
-1.51801702087436));
#77502=CARTESIAN_POINT('Ctrl Pts',(0.201546517088136,0.125813294406853,
-1.51707031295527));
#77503=CARTESIAN_POINT('Ctrl Pts',(0.193401382393456,0.137287602911918,
-1.51612360503618));
#77504=CARTESIAN_POINT('Ctrl Pts',(0.188606837527871,0.144041829697759,
-1.51556633572599));
#77505=CARTESIAN_POINT('Ctrl Pts',(0.18346562526578,0.150533934177916,-1.5150090664158));
#77506=CARTESIAN_POINT('Ctrl Pts',(0.178011591305242,0.156728599770353,
-1.51445179710561));
#77507=CARTESIAN_POINT('Ctrl Pts',(0.168730151462301,0.167270414592069,
-1.51350346022024));
#77508=CARTESIAN_POINT('Ctrl Pts',(0.158478018770147,0.177020135394206,
-1.51255512333488));
#77509=CARTESIAN_POINT('Ctrl Pts',(0.147415180258664,0.185797592164984,
-1.51160678644951));
#77510=CARTESIAN_POINT('Ctrl Pts',(0.136374636156082,0.194557360147287,
-1.51066036070207));
#77511=CARTESIAN_POINT('Ctrl Pts',(0.12452723184534,0.202348185692752,-1.50971393495463));
#77512=CARTESIAN_POINT('Ctrl Pts',(0.112068452964966,0.209027850955415,
-1.5087675092072));
#77513=CARTESIAN_POINT('Ctrl Pts',(0.0996116721553255,0.215706444969941,
-1.50782123524234));
#77514=CARTESIAN_POINT('Ctrl Pts',(0.0865444213950397,0.221273796036656,
-1.50687496127748));
#77515=CARTESIAN_POINT('Ctrl Pts',(0.0730888892767603,0.225632433150222,
-1.50592868731262));
#77516=CARTESIAN_POINT('Ctrl Pts',(0.0596355491877476,0.229990360201932,
-1.50498256750445));
#77517=CARTESIAN_POINT('Ctrl Pts',(0.0457948524215321,0.233139724829233,
-1.50403644769627));
#77518=CARTESIAN_POINT('Ctrl Pts',(0.0318043181461604,0.23503290402039,
-1.5030903278881));
#77519=CARTESIAN_POINT('Ctrl Pts',(0.0177813457353162,0.236930472693883,
-1.502142014428));
#77520=CARTESIAN_POINT('Ctrl Pts',(0.00360867606594497,0.237565973563984,
-1.5011937009679));
#77521=CARTESIAN_POINT('Ctrl Pts',(-0.0104713284861235,0.23694373151602,
-1.50024538750779));
#77522=CARTESIAN_POINT('Ctrl Pts',(-0.0186270676159718,0.236583302384051,
-1.4996960839074));
#77523=CARTESIAN_POINT('Ctrl Pts',(-0.0267517235308848,0.235801856681092,
-1.49914678030702));
#77524=CARTESIAN_POINT('Ctrl Pts',(-0.0347993793595566,0.234608149519981,
-1.49859747670663));
#77525=CARTESIAN_POINT('Ctrl Pts',(-0.0371826285580409,0.234254642648476,
-1.49843480481891));
#77526=CARTESIAN_POINT('Ctrl Pts',(-0.0395618469931956,0.233864615836945,
-1.49827213293119));
#77527=CARTESIAN_POINT('Ctrl Pts',(-0.0419358257166342,0.233438144154858,
-1.49810946104348));
#77528=CARTESIAN_POINT('',(0.137702479013102,-0.193106208855765,-1.5608));
#77529=CARTESIAN_POINT('Origin',(0.,0.,-1.5608));
#77530=CARTESIAN_POINT('Ctrl Pts',(0.137702479013101,-0.193106208855765,
-1.5608));
#77531=CARTESIAN_POINT('Ctrl Pts',(0.149478942681546,-0.184708507659302,
-1.55982940334437));
#77532=CARTESIAN_POINT('Ctrl Pts',(0.160499517164105,-0.175219427018632,
-1.55885880668873));
#77533=CARTESIAN_POINT('Ctrl Pts',(0.17056779482257,-0.164798689298082,
-1.5578882100331));
#77534=CARTESIAN_POINT('Ctrl Pts',(0.180628695633146,-0.154385586666636,
-1.55691832451636));
#77535=CARTESIAN_POINT('Ctrl Pts',(0.189738136346402,-0.14304273078033,
-1.55594843899963));
#77536=CARTESIAN_POINT('Ctrl Pts',(0.197736432649809,-0.130966727942357,
-1.55497855348289));
#77537=CARTESIAN_POINT('Ctrl Pts',(0.205744047618538,-0.118876655579501,
-1.5540075379707));
#77538=CARTESIAN_POINT('Ctrl Pts',(0.212637498410565,-0.10605237729402,
-1.5530365224585));
#77539=CARTESIAN_POINT('Ctrl Pts',(0.218300389818104,-0.0927195795410208,
-1.5520655069463));
#77540=CARTESIAN_POINT('Ctrl Pts',(0.223966545314624,-0.079379096767229,
-1.55109393174105));
#77541=CARTESIAN_POINT('Ctrl Pts',(0.228400465487478,-0.0655302442710616,
-1.55012235653579));
#77542=CARTESIAN_POINT('Ctrl Pts',(0.231534592040504,-0.0514170527513709,
-1.54915078133053));
#77543=CARTESIAN_POINT('Ctrl Pts',(0.234677425683833,-0.0372646525938184,
-1.54817650693846));
#77544=CARTESIAN_POINT('Ctrl Pts',(0.236513140568815,-0.0228472191527624,
-1.54720223254639));
#77545=CARTESIAN_POINT('Ctrl Pts',(0.237025582884283,-0.00841746300057407,
-1.54622795815432));
#77546=CARTESIAN_POINT('Ctrl Pts',(0.2372503976443,-0.00208695111944139,
-1.54580053196989));
#77547=CARTESIAN_POINT('Ctrl Pts',(0.237221203791196,0.00424591693677301,
-1.54537310578545));
#77548=CARTESIAN_POINT('Ctrl Pts',(0.236939796631132,0.0105599904070905,
-1.54494567960102));
#77549=CARTESIAN_POINT('Ctrl Pts',(0.236321990332825,0.0244220199199111,
-1.54400730053225));
#77550=CARTESIAN_POINT('Ctrl Pts',(0.234480871056891,0.0382861540118555,
-1.54306892146348));
#77551=CARTESIAN_POINT('Ctrl Pts',(0.231423179372956,0.0519162082004513,
-1.54213054239472));
#77552=CARTESIAN_POINT('Ctrl Pts',(0.228372420405316,0.0655153589139597,
-1.54119429091648));
#77553=CARTESIAN_POINT('Ctrl Pts',(0.224110660071987,0.0788806421642751,
-1.54025803943824));
#77554=CARTESIAN_POINT('Ctrl Pts',(0.218696210916371,0.0917820677247033,
-1.53932178796));
#77555=CARTESIAN_POINT('Ctrl Pts',(0.213283688291701,0.104678902791277,
-1.53838586961213));
#77556=CARTESIAN_POINT('Ctrl Pts',(0.206719564054125,0.117111399699901,
-1.53744995126426));
#77557=CARTESIAN_POINT('Ctrl Pts',(0.199111287314113,0.128866892137262,
-1.53651403291638));
#77558=CARTESIAN_POINT('Ctrl Pts',(0.191505257362885,0.140618913077796,
-1.53557839095316));
#77559=CARTESIAN_POINT('Ctrl Pts',(0.182856162507269,0.151693616802622,
-1.53464274898993));
#77560=CARTESIAN_POINT('Ctrl Pts',(0.173314975293426,0.161907072001316,
-1.5337071070267));
#77561=CARTESIAN_POINT('Ctrl Pts',(0.163751335877573,0.172144561374605,
-1.53276926332255));
#77562=CARTESIAN_POINT('Ctrl Pts',(0.153292029975829,0.181516161201482,
-1.53183141961839));
#77563=CARTESIAN_POINT('Ctrl Pts',(0.142124653048296,0.189875126388112,
-1.53089357591424));
#77564=CARTESIAN_POINT('Ctrl Pts',(0.134971352613422,0.195229489341259,
-1.53029283701017));
#77565=CARTESIAN_POINT('Ctrl Pts',(0.127528224370449,0.200169177942891,
-1.5296920981061));
#77566=CARTESIAN_POINT('Ctrl Pts',(0.119850226191402,0.204665346130872,
-1.52909135920203));
#77567=CARTESIAN_POINT('Ctrl Pts',(0.107714278591147,0.211772050281987,
-1.52814182317829));
#77568=CARTESIAN_POINT('Ctrl Pts',(0.0949040243045732,0.217819023637601,
-1.52719228715455));
#77569=CARTESIAN_POINT('Ctrl Pts',(0.0816285163303515,0.222685351890746,
-1.52624275113081));
#77570=CARTESIAN_POINT('Ctrl Pts',(0.0683792569347776,0.227542058350124,
-1.52529509254717));
#77571=CARTESIAN_POINT('Ctrl Pts',(0.0546673184985617,0.23122240437951,
-1.52434743396353));
#77572=CARTESIAN_POINT('Ctrl Pts',(0.0407235335477553,0.233652679078124,
-1.52339977537989));
#77573=CARTESIAN_POINT('Ctrl Pts',(0.0267801846357797,0.236082877779142,
-1.52245214643066));
#77574=CARTESIAN_POINT('Ctrl Pts',(0.0126058125709699,0.237262888211552,
-1.52150451748144));
#77575=CARTESIAN_POINT('Ctrl Pts',(-0.00155735652436486,0.237169886928455,
-1.52055688853221));
#77576=CARTESIAN_POINT('Ctrl Pts',(-0.0150981261894554,0.237080972579943,
-1.51965090306787));
#77577=CARTESIAN_POINT('Ctrl Pts',(-0.0286279485024635,0.23582882808328,
-1.51874491760353));
#77578=CARTESIAN_POINT('Ctrl Pts',(-0.0419358257166344,0.233438144154858,
-1.51783893213918));
#77579=CARTESIAN_POINT('Origin',(0.,0.,-1.7456589891905));
#77580=CARTESIAN_POINT('',(-0.0419358227397264,0.233438144689642,-1.39796759050954));
#77581=CARTESIAN_POINT('',(-0.0420041065163025,0.233814670441123,-1.41782827198422));
#77582=CARTESIAN_POINT('',(-0.0419358257166344,0.233438144154858,-1.7456589891905));
#77583=CARTESIAN_POINT('',(-0.237174982656716,9.07016348682755E-5,-1.47594101081397));
#77584=CARTESIAN_POINT('Ctrl Pts',(-0.0419358227397264,0.233438144689642,
-1.39796759050954));
#77585=CARTESIAN_POINT('Ctrl Pts',(-0.0385115227848158,0.234053300520784,
-1.3982158823771));
#77586=CARTESIAN_POINT('Ctrl Pts',(-0.0350737264621262,0.234593103052235,
-1.39846590841708));
#77587=CARTESIAN_POINT('Ctrl Pts',(-0.0228340253071061,0.236239849252627,
-1.39935797186273));
#77588=CARTESIAN_POINT('Ctrl Pts',(-0.0139839628830158,0.236928465946922,
-1.40000675194027));
#77589=CARTESIAN_POINT('Ctrl Pts',(0.0062048354393095,0.237364093489822,
-1.40147949715167));
#77590=CARTESIAN_POINT('Ctrl Pts',(0.0175304436519194,0.236797283269903,
-1.40230066413439));
#77591=CARTESIAN_POINT('Ctrl Pts',(0.0304816933296712,0.235214390114697,
-1.40320649359698));
#77592=CARTESIAN_POINT('Ctrl Pts',(0.0321878590607497,0.234986989220831,
-1.40332513900844));
#77593=CARTESIAN_POINT('Ctrl Pts',(0.0348481363742243,0.234602903491431,
-1.40350890508603));
#77594=CARTESIAN_POINT('Ctrl Pts',(0.0358039822502094,0.23445893003607,
-1.40357468449152));
#77595=CARTESIAN_POINT('Ctrl Pts',(0.0375012861816143,0.234192653166615,
-1.40369101608473));
#77596=CARTESIAN_POINT('Ctrl Pts',(0.03824305479765,0.234072668300515,-1.4037416921443));
#77597=CARTESIAN_POINT('Ctrl Pts',(0.040041031267924,0.233773061292673,
-1.40386414144227));
#77598=CARTESIAN_POINT('Ctrl Pts',(0.0410966092933508,0.233589805398562,
-1.40393571119502));
#77599=CARTESIAN_POINT('Ctrl Pts',(0.0444106392871122,0.232991305735389,
-1.40415950614305));
#77600=CARTESIAN_POINT('Ctrl Pts',(0.0466644010411356,0.23255039896938,
-1.40431038321784));
#77601=CARTESIAN_POINT('Ctrl Pts',(0.058794893214838,0.229993828917358,
-1.40511706439754));
#77602=CARTESIAN_POINT('Ctrl Pts',(0.0685363003703231,0.227281372891614,
-1.40574574024272));
#77603=CARTESIAN_POINT('Ctrl Pts',(0.0957465208308804,0.217795275175144,
-1.40752101448389));
#77604=CARTESIAN_POINT('Ctrl Pts',(0.112624314419017,0.209565956220392,
-1.40865116116187));
#77605=CARTESIAN_POINT('Ctrl Pts',(0.131626835676394,0.197335897561624,
-1.4101021456057));
#77606=CARTESIAN_POINT('Ctrl Pts',(0.134842071643729,0.195152999699572,
-1.41035421447998));
#77607=CARTESIAN_POINT('Ctrl Pts',(0.139525226924441,0.191802500136539,
-1.41073212287856));
#77608=CARTESIAN_POINT('Ctrl Pts',(0.141035360131173,0.190694821285337,
-1.41085569667013));
#77609=CARTESIAN_POINT('Ctrl Pts',(0.143714122362353,0.188680731328749,
-1.41107808339702));
#77610=CARTESIAN_POINT('Ctrl Pts',(0.14488770220306,0.187781045162446,-1.41117663131866));
#77611=CARTESIAN_POINT('Ctrl Pts',(0.147367584262801,0.185842838114168,
-1.41138731591022));
#77612=CARTESIAN_POINT('Ctrl Pts',(0.148671486572401,0.184801391238574,
-1.41149956519719));
#77613=CARTESIAN_POINT('Ctrl Pts',(0.152183327575941,0.181935207476623,
-1.41180599082377));
#77614=CARTESIAN_POINT('Ctrl Pts',(0.154369314046198,0.180084142960229,
-1.41200121847907));
#77615=CARTESIAN_POINT('Ctrl Pts',(0.15915197844672,0.175883170235995,-1.41243866022511));
#77616=CARTESIAN_POINT('Ctrl Pts',(0.161731172222493,0.173514459201455,
-1.4126816093225));
#77617=CARTESIAN_POINT('Ctrl Pts',(0.169798748114308,0.165769075430633,
-1.41346461481212));
#77618=CARTESIAN_POINT('Ctrl Pts',(0.175078348686338,0.160182876665333,
-1.41401272850317));
#77619=CARTESIAN_POINT('Ctrl Pts',(0.185812558339347,0.147659544691448,
-1.4152040761576));
#77620=CARTESIAN_POINT('Ctrl Pts',(0.191170327439097,0.140653986999804,
-1.4158486058659));
#77621=CARTESIAN_POINT('Ctrl Pts',(0.202534132182428,0.123942686382771,
-1.41732258603659));
#77622=CARTESIAN_POINT('Ctrl Pts',(0.208255764826146,0.114067779206743,
-1.41814923792898));
#77623=CARTESIAN_POINT('Ctrl Pts',(0.213999403889504,0.102270239278141,
-1.41906020408607));
#77624=CARTESIAN_POINT('Ctrl Pts',(0.2147364161444,0.100713547837493,-1.41917892625864));
#77625=CARTESIAN_POINT('Ctrl Pts',(0.215860613511241,0.0982706006451665,
-1.41936278546606));
#77626=CARTESIAN_POINT('Ctrl Pts',(0.216259429639905,0.097389807432605,
-1.41942858225961));
#77627=CARTESIAN_POINT('Ctrl Pts',(0.216958546654219,0.0958203217273344,
-1.41954492055797));
#77628=CARTESIAN_POINT('Ctrl Pts',(0.217260966693063,0.0951326305599371,
-1.41959558619686));
#77629=CARTESIAN_POINT('Ctrl Pts',(0.217986477397933,0.0934613431893207,
-1.41971798250195));
#77630=CARTESIAN_POINT('Ctrl Pts',(0.218406182192277,0.0924763033946822,
-1.41978951003484));
#77631=CARTESIAN_POINT('Ctrl Pts',(0.219703950920165,0.0893723401339488,
-1.42001308787452));
#77632=CARTESIAN_POINT('Ctrl Pts',(0.220557988058772,0.0872434300490766,
-1.42016379314305));
#77633=CARTESIAN_POINT('Ctrl Pts',(0.224996491361345,0.0756973298365073,
-1.42096872802044));
#77634=CARTESIAN_POINT('Ctrl Pts',(0.228009349873586,0.066070334627584,
-1.42159594882526));
#77635=CARTESIAN_POINT('Ctrl Pts',(0.234822507878949,0.0381783565535167,
-1.42336486101796));
#77636=CARTESIAN_POINT('Ctrl Pts',(0.237095305635452,0.0196204699282895,
-1.42449008134364));
#77637=CARTESIAN_POINT('Ctrl Pts',(0.237189437135739,-0.00297073851907267,
-1.42593975158081));
#77638=CARTESIAN_POINT('Ctrl Pts',(0.237106803290778,-0.00692930719472698,
-1.4261964496161));
#77639=CARTESIAN_POINT('Ctrl Pts',(0.236838594622866,-0.0127678475325734,
-1.42657993949217));
#77640=CARTESIAN_POINT('Ctrl Pts',(0.236729576540385,-0.0146507707299379,
-1.42670436332119));
#77641=CARTESIAN_POINT('Ctrl Pts',(0.236494965440406,-0.0180083828251615,
-1.42692766604776));
#77642=CARTESIAN_POINT('Ctrl Pts',(0.236378002591804,-0.0194835892956288,
-1.42702627070875));
#77643=CARTESIAN_POINT('Ctrl Pts',(0.23610054808405,-0.022611234457552,
-1.42723642030768));
#77644=CARTESIAN_POINT('Ctrl Pts',(0.23593649625322,-0.0242632689964275,
-1.42734807164072));
#77645=CARTESIAN_POINT('Ctrl Pts',(0.235446490425838,-0.0287212459295221,
-1.42765118190855));
#77646=CARTESIAN_POINT('Ctrl Pts',(0.235087737544856,-0.0315232339904567,
-1.42784365431889));
#77647=CARTESIAN_POINT('Ctrl Pts',(0.232319170964273,-0.0504556805905314,
-1.42915797094521));
#77648=CARTESIAN_POINT('Ctrl Pts',(0.22830150962364,-0.0663039106971981,
-1.43033089979363));
#77649=CARTESIAN_POINT('Ctrl Pts',(0.217737196604775,-0.0951303715589203,
-1.43257014431758));
#77650=CARTESIAN_POINT('Ctrl Pts',(0.211561906303192,-0.108170705424929,
-1.43362711178));
#77651=CARTESIAN_POINT('Ctrl Pts',(0.203112941795011,-0.122482820693217,
-1.43478809538256));
#77652=CARTESIAN_POINT('Ctrl Pts',(0.20195760122813,-0.124378602178046,
-1.43494185233243));
#77653=CARTESIAN_POINT('Ctrl Pts',(0.200213137941164,-0.127152652478288,
-1.43516649137864));
#77654=CARTESIAN_POINT('Ctrl Pts',(0.199644525764759,-0.128043590530309,
-1.43523858411618));
#77655=CARTESIAN_POINT('Ctrl Pts',(0.198618812406788,-0.129627299380353,
-1.43536659551601));
#77656=CARTESIAN_POINT('Ctrl Pts',(0.198164010562332,-0.13032150385923,
-1.43542265703305));
#77657=CARTESIAN_POINT('Ctrl Pts',(0.197145964434181,-0.131857785336601,
-1.43554660767136));
#77658=CARTESIAN_POINT('Ctrl Pts',(0.196580960679258,-0.13269865424826,
-1.43561437949057));
#77659=CARTESIAN_POINT('Ctrl Pts',(0.194887550087053,-0.135184325819797,
-1.43581458801289));
#77660=CARTESIAN_POINT('Ctrl Pts',(0.193743731047786,-0.136818589556655,
-1.43594604936458));
#77661=CARTESIAN_POINT('Ctrl Pts',(0.191037537522976,-0.140583133819324,
-1.4362489661089));
#77662=CARTESIAN_POINT('Ctrl Pts',(0.189459897267262,-0.142702161204216,
-1.43641954723445));
#77663=CARTESIAN_POINT('Ctrl Pts',(0.183754910419155,-0.15010344700502,
-1.43701733590484));
#77664=CARTESIAN_POINT('Ctrl Pts',(0.179439185425535,-0.155236925469464,
-1.43743566835982));
#77665=CARTESIAN_POINT('Ctrl Pts',(0.164359446309655,-0.171703422856967,
-1.43881571772802));
#77666=CARTESIAN_POINT('Ctrl Pts',(0.152695044690636,-0.182154633961043,
-1.43975884068888));
#77667=CARTESIAN_POINT('Ctrl Pts',(0.134475040986205,-0.195491237786616,
-1.44117824261699));
#77668=CARTESIAN_POINT('Ctrl Pts',(0.128684851892426,-0.199350334193594,
-1.44162202884404));
#77669=CARTESIAN_POINT('Ctrl Pts',(0.120693385116736,-0.204183186490165,
-1.44223054843731));
#77670=CARTESIAN_POINT('Ctrl Pts',(0.118634482409945,-0.205386284264406,
-1.44238697158936));
#77671=CARTESIAN_POINT('Ctrl Pts',(0.115193077608888,-0.207328220908325,
-1.44264804090642));
#77672=CARTESIAN_POINT('Ctrl Pts',(0.11382073544532,-0.20808478151291,-1.44275204771688));
#77673=CARTESIAN_POINT('Ctrl Pts',(0.111108015260505,-0.209545416652104,
-1.44295749532978));
#77674=CARTESIAN_POINT('Ctrl Pts',(0.109768191839825,-0.210250366401893,
-1.44305889893902));
#77675=CARTESIAN_POINT('Ctrl Pts',(0.106541729213029,-0.211908727354906,
-1.44330297863427));
#77676=CARTESIAN_POINT('Ctrl Pts',(0.104648941718163,-0.212849823320916,
-1.44344607596967));
#77677=CARTESIAN_POINT('Ctrl Pts',(0.0979208303261277,-0.216083611620292,
-1.44395455925712));
#77678=CARTESIAN_POINT('Ctrl Pts',(0.0930210722525494,-0.218237687910149,
-1.44432460087382));
#77679=CARTESIAN_POINT('Ctrl Pts',(0.0804665399451123,-0.223257411443849,
-1.44527264343318));
#77680=CARTESIAN_POINT('Ctrl Pts',(0.0727291138993964,-0.225896413281411,
-1.44585699716101));
#77681=CARTESIAN_POINT('Ctrl Pts',(0.0484925840948999,-0.232788348119927,
-1.44768090076866));
#77682=CARTESIAN_POINT('Ctrl Pts',(0.0316597436471689,-0.235668460739882,
-1.44894206829237));
#77683=CARTESIAN_POINT('Ctrl Pts',(0.0113577316712747,-0.236926048203879,
-1.45037926527418));
#77684=CARTESIAN_POINT('Ctrl Pts',(0.008047870637609,-0.237061563419197,
-1.45061078116697));
#77685=CARTESIAN_POINT('Ctrl Pts',(0.0034640937090203,-0.237153113473312,
-1.45092659849045));
#77686=CARTESIAN_POINT('Ctrl Pts',(0.00219190498361422,-0.237168283945298,
-1.4510137385851));
#77687=CARTESIAN_POINT('Ctrl Pts',(6.82070392426777E-5,-0.23717651841754,
-1.45115828139573));
#77688=CARTESIAN_POINT('Ctrl Pts',(-0.000783241418594574,-0.237175235129772,
-1.45121598484313));
#77689=CARTESIAN_POINT('Ctrl Pts',(-0.00253457421257168,-0.237163164059402,
-1.45133414100589));
#77690=CARTESIAN_POINT('Ctrl Pts',(-0.00343443356706208,-0.237151839940067,
-1.45139456418305));
#77691=CARTESIAN_POINT('Ctrl Pts',(-0.00579312183182301,-0.237108729181641,
-1.45155224232815));
#77692=CARTESIAN_POINT('Ctrl Pts',(-0.00725178649765415,-0.237068600983041,
-1.4516490503791));
#77693=CARTESIAN_POINT('Ctrl Pts',(-0.0140361093464927,-0.236819284811098,
-1.45209642249942));
#77694=CARTESIAN_POINT('Ctrl Pts',(-0.0193545418351217,-0.236444068392913,
-1.45243886043213));
#77695=CARTESIAN_POINT('Ctrl Pts',(-0.0360037235606818,-0.234703823142002,
-1.45349739019527));
#77696=CARTESIAN_POINT('Ctrl Pts',(-0.047251593670237,-0.232700396680081,
-1.45419335349711));
#77697=CARTESIAN_POINT('Ctrl Pts',(-0.0719890195642776,-0.226425821165901,
-1.45575911049224));
#77698=CARTESIAN_POINT('Ctrl Pts',(-0.0853274533528092,-0.221743623405162,
-1.45662900645784));
#77699=CARTESIAN_POINT('Ctrl Pts',(-0.101021615892802,-0.214607611641924,
-1.45773989316845));
#77700=CARTESIAN_POINT('Ctrl Pts',(-0.103847197587359,-0.213254664530967,
-1.45794345037883));
#77701=CARTESIAN_POINT('Ctrl Pts',(-0.108351474897206,-0.210987175704623,
-1.45827420285073));
#77702=CARTESIAN_POINT('Ctrl Pts',(-0.110047411805366,-0.210107584881623,
-1.45840019625464));
#77703=CARTESIAN_POINT('Ctrl Pts',(-0.113040872083618,-0.208508853497178,
-1.45862529097428));
#77704=CARTESIAN_POINT('Ctrl Pts',(-0.114342636695129,-0.207797839284336,
-1.45872410203686));
#77705=CARTESIAN_POINT('Ctrl Pts',(-0.117076446692352,-0.206271185741886,
-1.45893361942195));
#77706=CARTESIAN_POINT('Ctrl Pts',(-0.118506825851804,-0.205452740129825,
-1.45904442214966));
#77707=CARTESIAN_POINT('Ctrl Pts',(-0.122313682920159,-0.203221521548993,
-1.45934255654036));
#77708=CARTESIAN_POINT('Ctrl Pts',(-0.124674119595853,-0.201782027524024,
-1.45953084382207));
#77709=CARTESIAN_POINT('Ctrl Pts',(-0.138785438436959,-0.192834216910929,
-1.46067787415787));
#77710=CARTESIAN_POINT('Ctrl Pts',(-0.149878585889672,-0.184344031316412,
-1.46167306143995));
#77711=CARTESIAN_POINT('Ctrl Pts',(-0.170603941412359,-0.165368594017367,
-1.46371534232905));
#77712=CARTESIAN_POINT('Ctrl Pts',(-0.180170453569703,-0.154890629509906,
-1.46475874418413));
#77713=CARTESIAN_POINT('Ctrl Pts',(-0.19126534308864,-0.140309897044045,
-1.46606185369443));
#77714=CARTESIAN_POINT('Ctrl Pts',(-0.193697931935111,-0.136932154204561,
-1.46635432140335));
#77715=CARTESIAN_POINT('Ctrl Pts',(-0.196820056118584,-0.132347135583678,
-1.46673724577035));
#77716=CARTESIAN_POINT('Ctrl Pts',(-0.197589560264613,-0.131195520859702,
-1.46683227518843));
#77717=CARTESIAN_POINT('Ctrl Pts',(-0.198785307029542,-0.129371618726384,
-1.46698089979822));
#77718=CARTESIAN_POINT('Ctrl Pts',(-0.199218314282917,-0.128703835701187,
-1.46703492340966));
#77719=CARTESIAN_POINT('Ctrl Pts',(-0.200109503315686,-0.12731417164089,
-1.46714651567243));
#77720=CARTESIAN_POINT('Ctrl Pts',(-0.20056715391065,-0.126591976111283,
-1.46720404508168));
#77721=CARTESIAN_POINT('Ctrl Pts',(-0.20168420389995,-0.124807951455004,
-1.46734505789291));
#77722=CARTESIAN_POINT('Ctrl Pts',(-0.202339146342763,-0.123743334678699,
-1.46742825589117));
#77723=CARTESIAN_POINT('Ctrl Pts',(-0.204755126852568,-0.119745656667404,
-1.46773732509588));
#77724=CARTESIAN_POINT('Ctrl Pts',(-0.206461149029418,-0.11677962629092,
-1.4679599684805));
#77725=CARTESIAN_POINT('Ctrl Pts',(-0.210756962966191,-0.108922455065835,
-1.46853532621668));
#77726=CARTESIAN_POINT('Ctrl Pts',(-0.213240883127421,-0.103975633730006,
-1.46888333159881));
#77727=CARTESIAN_POINT('Ctrl Pts',(-0.222858481493534,-0.0830241386476146,
-1.47031717910625));
#77728=CARTESIAN_POINT('Ctrl Pts',(-0.228380644288481,-0.0663416267354367,
-1.47136820539355));
#77729=CARTESIAN_POINT('Ctrl Pts',(-0.233441074249819,-0.0424792295932923,
-1.47290221919543));
#77730=CARTESIAN_POINT('Ctrl Pts',(-0.234573873129283,-0.0356974047384165,
-1.47334089467773));
#77731=CARTESIAN_POINT('Ctrl Pts',(-0.235699166942779,-0.0265236168339529,
-1.47394318760822));
#77732=CARTESIAN_POINT('Ctrl Pts',(-0.235952472644799,-0.0241667030348894,
-1.47409869549489));
#77733=CARTESIAN_POINT('Ctrl Pts',(-0.236314112713833,-0.0202500336210339,
-1.47435857727544));
#77734=CARTESIAN_POINT('Ctrl Pts',(-0.236442430454597,-0.0186922607503921,
-1.47446232187662));
#77735=CARTESIAN_POINT('Ctrl Pts',(-0.236656367354034,-0.0157384966995887,
-1.47465981115459));
#77736=CARTESIAN_POINT('Ctrl Pts',(-0.236745054315237,-0.0143427891428809,
-1.47475345538074));
#77737=CARTESIAN_POINT('Ctrl Pts',(-0.236902105175347,-0.0114699448769709,
-1.47494691258588));
#77738=CARTESIAN_POINT('Ctrl Pts',(-0.236969008503276,-0.00999279284550699,
-1.47504676705725));
#77739=CARTESIAN_POINT('Ctrl Pts',(-0.237125281952006,-0.0056428633784824,
-1.47534199169133));
#77740=CARTESIAN_POINT('Ctrl Pts',(-0.237176246592844,-0.00276908247686686,
-1.47553853944128));
#77741=CARTESIAN_POINT('Ctrl Pts',(-0.23717497685085,0.000104789305429084,
-1.4757366710682));
#77742=CARTESIAN_POINT('Ctrl Pts',(-0.0419358257166342,0.233438144154858,
-1.49810946104348));
#77743=CARTESIAN_POINT('Ctrl Pts',(-0.0557685687745926,0.230953171083461,
-1.49716160148462));
#77744=CARTESIAN_POINT('Ctrl Pts',(-0.069422922806279,0.227226644879475,
-1.49621374192575));
#77745=CARTESIAN_POINT('Ctrl Pts',(-0.0826620679931504,0.222303763216226,
-1.49526588236689));
#77746=CARTESIAN_POINT('Ctrl Pts',(-0.0958768314395088,0.217389947729199,
-1.49431976842419));
#77747=CARTESIAN_POINT('Ctrl Pts',(-0.108677107711918,0.211284379769945,
-1.49337365448149));
#77748=CARTESIAN_POINT('Ctrl Pts',(-0.120840594102836,0.204082168358418,
-1.49242754053879));
#77749=CARTESIAN_POINT('Ctrl Pts',(-0.133004145272652,0.19687991859018,
-1.49148142155739));
#77750=CARTESIAN_POINT('Ctrl Pts',(-0.144530162094799,0.188581402075368,
-1.49053530257598));
#77751=CARTESIAN_POINT('Ctrl Pts',(-0.155221192718087,0.179327527045277,
-1.48958918359458));
#77752=CARTESIAN_POINT('Ctrl Pts',(-0.165912151595259,0.170073714116737,
-1.48864307096246));
#77753=CARTESIAN_POINT('Ctrl Pts',(-0.175767522195974,0.159865120916746,
-1.48769695833033));
#77754=CARTESIAN_POINT('Ctrl Pts',(-0.184624890693679,0.14888126262679,
-1.48675084569821));
#77755=CARTESIAN_POINT('Ctrl Pts',(-0.1935024630955,0.137872349850303,-1.48580257495683));
#77756=CARTESIAN_POINT('Ctrl Pts',(-0.201377010051896,0.126085326568405,
-1.48485430421546));
#77757=CARTESIAN_POINT('Ctrl Pts',(-0.208128362015914,0.113730231467155,
-1.48390603347408));
#77758=CARTESIAN_POINT('Ctrl Pts',(-0.210888119927161,0.108679825025362,
-1.48351840775194));
#77759=CARTESIAN_POINT('Ctrl Pts',(-0.213460739258607,0.103534776502822,
-1.48313078202979));
#77760=CARTESIAN_POINT('Ctrl Pts',(-0.215840324500079,0.0983104009995918,
-1.48274315630764));
#77761=CARTESIAN_POINT('Ctrl Pts',(-0.222182201605667,0.0843868201933717,
-1.48171008775016));
#77762=CARTESIAN_POINT('Ctrl Pts',(-0.227186699712206,0.0698174069716404,
-1.48067701919268));
#77763=CARTESIAN_POINT('Ctrl Pts',(-0.230742419362563,0.0548627062011248,
-1.47964395063519));
#77764=CARTESIAN_POINT('Ctrl Pts',(-0.234275250085543,0.040004272035841,
-1.47861753216082));
#77765=CARTESIAN_POINT('Ctrl Pts',(-0.236377637504013,0.0247660283467118,
-1.47759111368645));
#77766=CARTESIAN_POINT('Ctrl Pts',(-0.236987714546397,0.0094235757054001,
-1.47656469521208));
#77767=CARTESIAN_POINT('Ctrl Pts',(-0.237111281928992,0.0063160555337377,
-1.47635680041271));
#77768=CARTESIAN_POINT('Ctrl Pts',(-0.237173791934776,0.00320431095113047,
-1.47614890561334));
#77769=CARTESIAN_POINT('Ctrl Pts',(-0.237174982656716,9.07016348682755E-5,
-1.47594101081397));
#77770=CARTESIAN_POINT('',(-0.237174946895483,0.000158713971423185,-1.4956589891905));
#77771=CARTESIAN_POINT('Ctrl Pts',(-0.0419358257166344,0.233438144154858,
-1.51783893213918));
#77772=CARTESIAN_POINT('Ctrl Pts',(-0.0558810547429703,0.23093296362344,
-1.51688955647307));
#77773=CARTESIAN_POINT('Ctrl Pts',(-0.0695817208837182,0.227177409959992,
-1.51594018080695));
#77774=CARTESIAN_POINT('Ctrl Pts',(-0.0828077196110171,0.222249549375973,
-1.51499080514083));
#77775=CARTESIAN_POINT('Ctrl Pts',(-0.0909517775708719,0.219215163614881,
-1.51440621636157));
#77776=CARTESIAN_POINT('Ctrl Pts',(-0.0989161661920512,0.21573728046195,
-1.51382162758231));
#77777=CARTESIAN_POINT('Ctrl Pts',(-0.10665151759329,0.211842947534366,
-1.51323703880304));
#77778=CARTESIAN_POINT('Ctrl Pts',(-0.119218195906053,0.20551630164522,
-1.51228732898985));
#77779=CARTESIAN_POINT('Ctrl Pts',(-0.131260473127216,0.198047205927597,
-1.51133761917666));
#77780=CARTESIAN_POINT('Ctrl Pts',(-0.142563372296947,0.189545945628816,
-1.51038790936346));
#77781=CARTESIAN_POINT('Ctrl Pts',(-0.153844132760301,0.181061336536311,
-1.50944005972317));
#77782=CARTESIAN_POINT('Ctrl Pts',(-0.164387692340001,0.171549016985991,
-1.50849221008287));
#77783=CARTESIAN_POINT('Ctrl Pts',(-0.174006991136474,0.161163108869962,
-1.50754436044258));
#77784=CARTESIAN_POINT('Ctrl Pts',(-0.183625303303705,0.15077826601252,
-1.50659660802103));
#77785=CARTESIAN_POINT('Ctrl Pts',(-0.19231894469696,0.139520588804458,
-1.50564885559948));
#77786=CARTESIAN_POINT('Ctrl Pts',(-0.199937509431487,0.127581240577657,
-1.50470110317793));
#77787=CARTESIAN_POINT('Ctrl Pts',(-0.207555098166764,0.115643421877128,
-1.50375347217107));
#77788=CARTESIAN_POINT('Ctrl Pts',(-0.214097453328319,0.103024816868292,
-1.50280584116421));
#77789=CARTESIAN_POINT('Ctrl Pts',(-0.219458590204809,0.0899439148042685,
-1.50185821015735));
#77790=CARTESIAN_POINT('Ctrl Pts',(-0.224832259753346,0.0768324336561026,
-1.50090836388367));
#77791=CARTESIAN_POINT('Ctrl Pts',(-0.229018924614474,0.0632572854076371,
-1.49995851760998));
#77792=CARTESIAN_POINT('Ctrl Pts',(-0.231961665499544,0.0494546900068923,
-1.4990086713363));
#77793=CARTESIAN_POINT('Ctrl Pts',(-0.233640799728419,0.0415788996162779,
-1.49846668702556));
#77794=CARTESIAN_POINT('Ctrl Pts',(-0.234915868802463,0.0336292874429718,
-1.49792470271481));
#77795=CARTESIAN_POINT('Ctrl Pts',(-0.235783863370645,0.0256505438346448,
-1.49738271840406));
#77796=CARTESIAN_POINT('Ctrl Pts',(-0.236704054579574,0.0171920004337824,
-1.49680814199954));
#77797=CARTESIAN_POINT('Ctrl Pts',(-0.237169242852117,0.00868257718441503,
-1.49623356559502));
#77798=CARTESIAN_POINT('Ctrl Pts',(-0.237174946895483,0.000158713971423185,
-1.4956589891905));
#77799=CARTESIAN_POINT('Ctrl Pts',(-0.237447721697233,0.000156842808466644,
-1.49565885091385));
#77800=CARTESIAN_POINT('Ctrl Pts',(-0.236948243252312,-0.0697991706694208,
-1.49094869994426));
#77801=CARTESIAN_POINT('Ctrl Pts',(-0.167292428838403,-0.21916121968206,
-1.48095377550834));
#77802=CARTESIAN_POINT('Ctrl Pts',(0.0863349738534437,-0.266549188346143,
-1.46567407760609));
#77803=CARTESIAN_POINT('Ctrl Pts',(0.270673100350359,-0.0724268647347502,
-1.44981975720711));
#77804=CARTESIAN_POINT('Ctrl Pts',(0.207909186801171,0.187842407039071,
-1.43396543680812));
#77805=CARTESIAN_POINT('Ctrl Pts',(0.0380245598870128,0.247548846411421,
-1.42330160840049));
#77806=CARTESIAN_POINT('Ctrl Pts',(-0.0406278707645089,0.234064275081112,
-1.41792255345919));
#77807=CARTESIAN_POINT('Ctrl Pts',(-0.0420041065163025,0.233814670441123,
-1.41782827198422));
#77808=CARTESIAN_POINT('Origin',(0.,0.,-1.7456589891905));
#77809=CARTESIAN_POINT('',(-0.0419357855265134,0.233438151374779,-1.29797390460371));
#77810=CARTESIAN_POINT('',(-0.0419358330286197,0.233438142841301,-1.31793598285019));
#77811=CARTESIAN_POINT('',(-0.0419358257166344,0.233438144154858,-1.7456589891905));
#77812=CARTESIAN_POINT('Ctrl Pts',(-0.0419357855265143,0.233438151374779,
-1.29797390460371));
#77813=CARTESIAN_POINT('Ctrl Pts',(-0.0356815834665369,0.23456168184605,
-1.29837265202323));
#77814=CARTESIAN_POINT('Ctrl Pts',(-0.0293811282187784,0.235434073806115,
-1.29877694890039));
#77815=CARTESIAN_POINT('Ctrl Pts',(-0.0201633428806279,0.236334146715947,
-1.29937698695918));
#77816=CARTESIAN_POINT('Ctrl Pts',(-0.0172724797192631,0.236562992781477,
-1.29956636593925));
#77817=CARTESIAN_POINT('Ctrl Pts',(-0.0127051448028816,0.23684038826945,
-1.29986780838322));
#77818=CARTESIAN_POINT('Ctrl Pts',(-0.0110310500785527,0.236924261973956,
-1.29997877052277));
#77819=CARTESIAN_POINT('Ctrl Pts',(-0.00787985660688119,0.237048669258367,
-1.30018859169584));
#77820=CARTESIAN_POINT('Ctrl Pts',(-0.00640298786574809,0.237093157459478,
-1.30028732233165));
#77821=CARTESIAN_POINT('Ctrl Pts',(-0.00306545500570211,0.237162488796146,
-1.30051137526909));
#77822=CARTESIAN_POINT('Ctrl Pts',(-0.00120473916601999,0.237179238904851,
-1.3006369437093));
#77823=CARTESIAN_POINT('Ctrl Pts',(0.00361807646716839,0.237165900774792,
-1.30096418744831));
#77824=CARTESIAN_POINT('Ctrl Pts',(0.00657968127167582,0.237102217173144,
-1.30116688669007));
#77825=CARTESIAN_POINT('Ctrl Pts',(0.027774878239727,0.236249053690374,
-1.30263057284041));
#77826=CARTESIAN_POINT('Ctrl Pts',(0.0458617641182701,0.233412763704121,
-1.30395581274328));
#77827=CARTESIAN_POINT('Ctrl Pts',(0.0749562716701144,0.225336107315267,
-1.30615962450828));
#77828=CARTESIAN_POINT('Ctrl Pts',(0.0862147971548094,0.2212732937283,-1.30702959026431));
#77829=CARTESIAN_POINT('Ctrl Pts',(0.098966661662484,0.215549710688493,
-1.30800366101553));
#77830=CARTESIAN_POINT('Ctrl Pts',(0.100802737872338,0.214697197505889,
-1.30814360145063));
#77831=CARTESIAN_POINT('Ctrl Pts',(0.103546399557912,0.213380322656402,
-1.30835200494468));
#77832=CARTESIAN_POINT('Ctrl Pts',(0.104462220559208,0.212933472077213,
-1.30842144845986));
#77833=CARTESIAN_POINT('Ctrl Pts',(0.106118555756728,0.212112048962696,
-1.30854678531595));
#77834=CARTESIAN_POINT('Ctrl Pts',(0.106860005420303,0.211739482574178,
-1.30860279380196));
#77835=CARTESIAN_POINT('Ctrl Pts',(0.108535631801202,0.210886463897045,
-1.30872915460454));
#77836=CARTESIAN_POINT('Ctrl Pts',(0.109468587258053,0.210403689448779,
-1.30879936253886));
#77837=CARTESIAN_POINT('Ctrl Pts',(0.112332563545517,0.208897467363209,
-1.30901452664639));
#77838=CARTESIAN_POINT('Ctrl Pts',(0.114252732678571,0.207853483516654,
-1.30915827798821));
#77839=CARTESIAN_POINT('Ctrl Pts',(0.129007174107794,0.199565326307494,
-1.31026106335337));
#77840=CARTESIAN_POINT('Ctrl Pts',(0.141157186330558,0.191164686746783,
-1.31115991449037));
#77841=CARTESIAN_POINT('Ctrl Pts',(0.164616073204325,0.171481058161546,
-1.31303788325358));
#77842=CARTESIAN_POINT('Ctrl Pts',(0.175724626897241,0.160078031720973,
-1.31401453224822));
#77843=CARTESIAN_POINT('Ctrl Pts',(0.18741540607085,0.145381763767024,-1.31523117935613));
#77844=CARTESIAN_POINT('Ctrl Pts',(0.189179040879372,0.143079282111341,
-1.31542058442191));
#77845=CARTESIAN_POINT('Ctrl Pts',(0.191894691798205,0.13939590300908,-1.31572205901251));
#77846=CARTESIAN_POINT('Ctrl Pts',(0.192875077085216,0.138036208702767,
-1.31583302681193));
#77847=CARTESIAN_POINT('Ctrl Pts',(0.194692335142278,0.135458696095318,
-1.31604285297072));
#77848=CARTESIAN_POINT('Ctrl Pts',(0.1955324040131,0.134243221513283,-1.31614158286913));
#77849=CARTESIAN_POINT('Ctrl Pts',(0.197404592492912,0.131479540217701,
-1.3163656263443));
#77850=CARTESIAN_POINT('Ctrl Pts',(0.198429949392734,0.129926892808175,
-1.31649118597169));
#77851=CARTESIAN_POINT('Ctrl Pts',(0.201039825656098,0.125871922403272,
-1.31681839037012));
#77852=CARTESIAN_POINT('Ctrl Pts',(0.202595888025147,0.123351761769579,
-1.31702105867031));
#77853=CARTESIAN_POINT('Ctrl Pts',(0.213402310709098,0.10509366182779,-1.31848501906883));
#77854=CARTESIAN_POINT('Ctrl Pts',(0.22085394003321,0.0883658384830213,
-1.31981060071742));
#77855=CARTESIAN_POINT('Ctrl Pts',(0.229887277007946,0.0595529943387015,
-1.32201447970667));
#77856=CARTESIAN_POINT('Ctrl Pts',(0.232595298218134,0.04789785306129,-1.32288417717998));
#77857=CARTESIAN_POINT('Ctrl Pts',(0.234721481644093,0.0340867079382427,
-1.32385799502002));
#77858=CARTESIAN_POINT('Ctrl Pts',(0.235003848364171,0.0320822308787528,
-1.32399793030747));
#77859=CARTESIAN_POINT('Ctrl Pts',(0.235389737772768,0.0290635558902885,
-1.32420632775149));
#77860=CARTESIAN_POINT('Ctrl Pts',(0.235512433664742,0.0280519627778268,
-1.3242757702817));
#77861=CARTESIAN_POINT('Ctrl Pts',(0.235723211632927,0.0262151995384508,
-1.32440110607555));
#77862=CARTESIAN_POINT('Ctrl Pts',(0.235813485932486,0.0253903345766434,
-1.32445711447523));
#77863=CARTESIAN_POINT('Ctrl Pts',(0.23600823123509,0.0235201794212471,
-1.32458347597471));
#77864=CARTESIAN_POINT('Ctrl Pts',(0.236110089081015,0.0224746521514455,
-1.32465368468257));
#77865=CARTESIAN_POINT('Ctrl Pts',(0.23640245663755,0.0192518967614226,
-1.32486885449985));
#77866=CARTESIAN_POINT('Ctrl Pts',(0.236569828329751,0.0170726151586642,
-1.32501261067615));
#77867=CARTESIAN_POINT('Ctrl Pts',(0.237864193052071,-0.00350225378583714,
-1.3263560205701));
#77868=CARTESIAN_POINT('Ctrl Pts',(0.236873663798885,-0.0219706016214408,
-1.32746154678167));
#77869=CARTESIAN_POINT('Ctrl Pts',(0.232010587234733,-0.0502905722377621,
-1.32923121290721));
#77870=CARTESIAN_POINT('Ctrl Pts',(0.229608381542239,-0.0603159563745694,
-1.3298720899765));
#77871=CARTESIAN_POINT('Ctrl Pts',(0.22536368248678,-0.0740244365331746,
-1.33079226410555));
#77872=CARTESIAN_POINT('Ctrl Pts',(0.22406591743754,-0.0778644213959656,
-1.3310549027869));
#77873=CARTESIAN_POINT('Ctrl Pts',(0.222015098974196,-0.08345596963305,
-1.33144557234544));
#77874=CARTESIAN_POINT('Ctrl Pts',(0.221338258356063,-0.0852348407468056,
-1.33157110218501));
#77875=CARTESIAN_POINT('Ctrl Pts',(0.220096481854711,-0.088383908571288,
-1.33179564201375));
#77876=CARTESIAN_POINT('Ctrl Pts',(0.219539968033937,-0.0897573333198564,
-1.33189436618155));
#77877=CARTESIAN_POINT('Ctrl Pts',(0.218336419208842,-0.0926494113637381,
-1.33210398376296));
#77878=CARTESIAN_POINT('Ctrl Pts',(0.217686329143207,-0.0941666992343994,
-1.33221497620264));
#77879=CARTESIAN_POINT('Ctrl Pts',(0.215899189980714,-0.0982203965159218,
-1.33251432423628));
#77880=CARTESIAN_POINT('Ctrl Pts',(0.214733332043485,-0.100743741718888,
-1.33270365015046));
#77881=CARTESIAN_POINT('Ctrl Pts',(0.207736208029548,-0.115214530628078,
-1.33380724406798));
#77882=CARTESIAN_POINT('Ctrl Pts',(0.200953900236698,-0.126673377471663,
-1.33475435316393));
#77883=CARTESIAN_POINT('Ctrl Pts',(0.185694362214561,-0.14811947391486,
-1.33666491128915));
#77884=CARTESIAN_POINT('Ctrl Pts',(0.177277843696724,-0.158096004707518,
-1.33762422415913));
#77885=CARTESIAN_POINT('Ctrl Pts',(0.164064856101045,-0.171368502915784,
-1.33896807698471));
#77886=CARTESIAN_POINT('Ctrl Pts',(0.159900698971384,-0.175260431693226,
-1.33937159561583));
#77887=CARTESIAN_POINT('Ctrl Pts',(0.154476371922974,-0.179975686919883,
-1.33986863855301));
#77888=CARTESIAN_POINT('Ctrl Pts',(0.15334349266036,-0.180941899260514,
-1.33997094605253));
#77889=CARTESIAN_POINT('Ctrl Pts',(0.151506698747924,-0.18247882542219,
-1.34013432430975));
#77890=CARTESIAN_POINT('Ctrl Pts',(0.1508085030203,-0.183056267249122,-1.34019585659972));
#77891=CARTESIAN_POINT('Ctrl Pts',(0.14945111682113,-0.184165854448735,
-1.34031435641435));
#77892=CARTESIAN_POINT('Ctrl Pts',(0.148792360823586,-0.184698488493589,
-1.34037135636453));
#77893=CARTESIAN_POINT('Ctrl Pts',(0.147310739668852,-0.185883374963248,
-1.34049845419781));
#77894=CARTESIAN_POINT('Ctrl Pts',(0.146486357613181,-0.186533724148596,
-1.34056842003342));
#77895=CARTESIAN_POINT('Ctrl Pts',(0.143554273847945,-0.188815397866359,
-1.34081473039456));
#77896=CARTESIAN_POINT('Ctrl Pts',(0.14142333486013,-0.190416716207678,
-1.34098914443833));
#77897=CARTESIAN_POINT('Ctrl Pts',(0.124879274300976,-0.202417959823925,
-1.34231233260961));
#77898=CARTESIAN_POINT('Ctrl Pts',(0.109363508111551,-0.211205235718552,
-1.34337951637296));
#77899=CARTESIAN_POINT('Ctrl Pts',(0.0854046120766593,-0.221419021527631,
-1.34498397526705));
#77900=CARTESIAN_POINT('Ctrl Pts',(0.0776355624248473,-0.224261087058582,
-1.34549757559088));
#77901=CARTESIAN_POINT('Ctrl Pts',(0.066228833926949,-0.227770003344585,
-1.34625536969454));
#77902=CARTESIAN_POINT('Ctrl Pts',(0.0626988273682074,-0.228766885251032,
-1.34649033735879));
#77903=CARTESIAN_POINT('Ctrl Pts',(0.0562717487439546,-0.230421977725582,
-1.34692001570409));
#77904=CARTESIAN_POINT('Ctrl Pts',(0.0533826951552514,-0.23110838173588,
-1.34711383349519));
#77905=CARTESIAN_POINT('Ctrl Pts',(0.0488295217204145,-0.232100231310048,
-1.34742072270118));
#77906=CARTESIAN_POINT('Ctrl Pts',(0.0471736614122442,-0.232442433703559,
-1.34753262292408));
#77907=CARTESIAN_POINT('Ctrl Pts',(0.0440660050542402,-0.233050092550856,
-1.34774324859984));
#77908=CARTESIAN_POINT('Ctrl Pts',(0.0426151082761807,-0.233319760880015,
-1.34784183488974));
#77909=CARTESIAN_POINT('Ctrl Pts',(0.0393505874012215,-0.233895049812903,
-1.34806425908346));
#77910=CARTESIAN_POINT('Ctrl Pts',(0.0375357521951193,-0.234193146851851,
-1.34818832849976));
#77911=CARTESIAN_POINT('Ctrl Pts',(0.032172644630773,-0.23501012839468,
-1.34855629164672));
#77912=CARTESIAN_POINT('Ctrl Pts',(0.0286159991199586,-0.235469661897079,
-1.34880201926783));
#77913=CARTESIAN_POINT('Ctrl Pts',(0.00614476469676354,-0.237856427884637,
-1.35036605240399));
#77914=CARTESIAN_POINT('Ctrl Pts',(-0.0129308310718226,-0.237583616622203,
-1.35175308476257));
#77915=CARTESIAN_POINT('Ctrl Pts',(-0.0418664844139423,-0.233673028299149,
-1.35388211840228));
#77916=CARTESIAN_POINT('Ctrl Pts',(-0.0518705825065041,-0.231657871601777,
-1.35462109642587));
#77917=CARTESIAN_POINT('Ctrl Pts',(-0.0639408871745872,-0.228405032857378,
-1.35549520514729));
#77918=CARTESIAN_POINT('Ctrl Pts',(-0.066158235293999,-0.227772660724465,
-1.35565501665582));
#77919=CARTESIAN_POINT('Ctrl Pts',(-0.0693935479898279,-0.226798737678322,
-1.35588672705042));
#77920=CARTESIAN_POINT('Ctrl Pts',(-0.0704189012452659,-0.226482472554529,
-1.35595994380997));
#77921=CARTESIAN_POINT('Ctrl Pts',(-0.0721587491312422,-0.225932866995077,
-1.35608376691195));
#77922=CARTESIAN_POINT('Ctrl Pts',(-0.0728743261634547,-0.225703075099686,
-1.35613457271426));
#77923=CARTESIAN_POINT('Ctrl Pts',(-0.0745065750487541,-0.225170341908694,
-1.35625017869265));
#77924=CARTESIAN_POINT('Ctrl Pts',(-0.0754225027486349,-0.224865201314728,
-1.35631485027713));
#77925=CARTESIAN_POINT('Ctrl Pts',(-0.077961009318451,-0.224002244260091,
-1.35649359863398));
#77926=CARTESIAN_POINT('Ctrl Pts',(-0.0795794744509733,-0.22343238814436,
-1.35660700428359));
#77927=CARTESIAN_POINT('Ctrl Pts',(-0.0909210014600033,-0.219300199747203,
-1.35739871354855));
#77928=CARTESIAN_POINT('Ctrl Pts',(-0.100409034682874,-0.215121561267084,
-1.35804573589368));
#77929=CARTESIAN_POINT('Ctrl Pts',(-0.111254590787385,-0.209470524493601,
-1.35880037274307));
#77930=CARTESIAN_POINT('Ctrl Pts',(-0.112904367507583,-0.208585925957488,
-1.35891558519284));
#77931=CARTESIAN_POINT('Ctrl Pts',(-0.121632093978949,-0.20377229263534,
-1.35952815769962));
#77932=CARTESIAN_POINT('Ctrl Pts',(-0.128515798566275,-0.199502385177493,
-1.36002235270214));
#77933=CARTESIAN_POINT('Ctrl Pts',(-0.141427876311033,-0.190547050241054,
-1.36099272085092));
#77934=CARTESIAN_POINT('Ctrl Pts',(-0.147474841390952,-0.185906376444795,
-1.36146765496924));
#77935=CARTESIAN_POINT('Ctrl Pts',(-0.157181338721424,-0.177685235778625,
-1.36227695095893));
#77936=CARTESIAN_POINT('Ctrl Pts',(-0.160967273026642,-0.174262868422231,
-1.36260568339115));
#77937=CARTESIAN_POINT('Ctrl Pts',(-0.166134703692136,-0.169279515983874,
-1.36307533320037));
#77938=CARTESIAN_POINT('Ctrl Pts',(-0.167610665108986,-0.167818231405802,
-1.36321201742534));
#77939=CARTESIAN_POINT('Ctrl Pts',(-0.170124435174203,-0.165263213163865,
-1.36344937490728));
#77940=CARTESIAN_POINT('Ctrl Pts',(-0.171171372744094,-0.164178604096371,
-1.36354964165154));
#77941=CARTESIAN_POINT('Ctrl Pts',(-0.173163692109138,-0.16207482406146,
-1.36374323387447));
#77942=CARTESIAN_POINT('Ctrl Pts',(-0.174110595073983,-0.161057174321265,
-1.36383648813062));
#77943=CARTESIAN_POINT('Ctrl Pts',(-0.176582349273387,-0.158353472756012,
-1.36408326493934));
#77944=CARTESIAN_POINT('Ctrl Pts',(-0.178091968086203,-0.156653754142891,
-1.36423741703766));
#77945=CARTESIAN_POINT('Ctrl Pts',(-0.183521678072306,-0.150360372009771,
-1.36480479692139));
#77946=CARTESIAN_POINT('Ctrl Pts',(-0.187290082216158,-0.145639492109189,
-1.36522403431857));
#77947=CARTESIAN_POINT('Ctrl Pts',(-0.200632579960041,-0.127549351721758,
-1.3668082445995));
#77948=CARTESIAN_POINT('Ctrl Pts',(-0.208988026649325,-0.113340841070711,
-1.36801339816816));
#77949=CARTESIAN_POINT('Ctrl Pts',(-0.218682357394607,-0.0920764815813074,
-1.36971514978385));
#77950=CARTESIAN_POINT('Ctrl Pts',(-0.221280623977151,-0.085644318545201,
-1.37021710475253));
#77951=CARTESIAN_POINT('Ctrl Pts',(-0.224919421688914,-0.0753593957652675,
-1.37099160631891));
#77952=CARTESIAN_POINT('Ctrl Pts',(-0.226151046528502,-0.0715785820053708,
-1.37127051310378));
#77953=CARTESIAN_POINT('Ctrl Pts',(-0.227664673022354,-0.0665020548682916,
-1.3716357744557));
#77954=CARTESIAN_POINT('Ctrl Pts',(-0.228031652133885,-0.0652326028274289,
-1.37172635288591));
#77955=CARTESIAN_POINT('Ctrl Pts',(-0.228622564107025,-0.0631225813856818,
-1.37187557599183));
#77956=CARTESIAN_POINT('Ctrl Pts',(-0.228852512332779,-0.0622837440740553,
-1.37193455229684));
#77957=CARTESIAN_POINT('Ctrl Pts',(-0.229307913214832,-0.0605858912948844,
-1.37205319678235));
#77958=CARTESIAN_POINT('Ctrl Pts',(-0.229533165143973,-0.0597268402924974,
-1.37211285343147));
#77959=CARTESIAN_POINT('Ctrl Pts',(-0.230102745793748,-0.0575037908385168,
-1.37226631851309));
#77960=CARTESIAN_POINT('Ctrl Pts',(-0.230439779837097,-0.0561379345016123,
-1.37235972209924));
#77961=CARTESIAN_POINT('Ctrl Pts',(-0.231768403757476,-0.0505398997054712,
-1.3727392295504));
#77962=CARTESIAN_POINT('Ctrl Pts',(-0.232655778509416,-0.0462835688121242,
-1.3730200682004));
#77963=CARTESIAN_POINT('Ctrl Pts',(-0.235907615415331,-0.0282127848867452,
-1.37418923518371));
#77964=CARTESIAN_POINT('Ctrl Pts',(-0.2371624653087,-0.0142266276722643,
-1.37503872842268));
#77965=CARTESIAN_POINT('Ctrl Pts',(-0.23718716775891,0.0136027218036718,
-1.37674851656479));
#77966=CARTESIAN_POINT('Ctrl Pts',(-0.235992727765574,0.0273888476668221,
-1.37760563568916));
#77967=CARTESIAN_POINT('Ctrl Pts',(-0.233124288714224,0.0437356559762051,
-1.37868215379816));
#77968=CARTESIAN_POINT('Ctrl Pts',(-0.232594510634388,0.0464707881844598,
-1.37886425701086));
#77969=CARTESIAN_POINT('Ctrl Pts',(-0.231674030153142,0.0508119425741966,
-1.37915676692936));
#77970=CARTESIAN_POINT('Ctrl Pts',(-0.231314495548988,0.0524243614375532,
-1.37926618278226));
#77971=CARTESIAN_POINT('Ctrl Pts',(-0.23060061972385,0.0554754893528476,
-1.37947475347017));
#77972=CARTESIAN_POINT('Ctrl Pts',(-0.23024958230856,0.0569148962185885,
-1.37957379812391));
#77973=CARTESIAN_POINT('Ctrl Pts',(-0.229417443049485,0.060193276384009,
-1.37980091132009));
#77974=CARTESIAN_POINT('Ctrl Pts',(-0.228927678215585,0.062029924060232,
-1.37992925311125));
#77975=CARTESIAN_POINT('Ctrl Pts',(-0.2273282766491,0.0677506604950433,
-1.38033257786884));
#77976=CARTESIAN_POINT('Ctrl Pts',(-0.2261415070581,0.0716122383843702,
-1.38061001753718));
#77977=CARTESIAN_POINT('Ctrl Pts',(-0.221732005447868,0.0847549672293667,
-1.38157275132017));
#77978=CARTESIAN_POINT('Ctrl Pts',(-0.218031984731433,0.0938642587194592,
-1.38227265924416));
#77979=CARTESIAN_POINT('Ctrl Pts',(-0.211315873395721,0.107842070651639,
-1.38339454517707));
#77980=CARTESIAN_POINT('Ctrl Pts',(-0.208669935687468,0.11287677027982,
-1.38380896285301));
#77981=CARTESIAN_POINT('Ctrl Pts',(-0.199345160363129,0.129169465143316,
-1.38517916920891));
#77982=CARTESIAN_POINT('Ctrl Pts',(-0.191915117017114,0.139971040875455,
-1.3861363832532));
#77983=CARTESIAN_POINT('Ctrl Pts',(-0.182189411815351,0.151868985162163,
-1.3872105756967));
#77984=CARTESIAN_POINT('Ctrl Pts',(-0.180722215689246,0.153612018211657,
-1.3873684485579));
#77985=CARTESIAN_POINT('Ctrl Pts',(-0.178530673670137,0.156140704372718,
-1.38759789906506));
#77986=CARTESIAN_POINT('Ctrl Pts',(-0.177825821422167,0.156942978017678,
-1.38767075978209));
#77987=CARTESIAN_POINT('Ctrl Pts',(-0.176563199469565,0.15836068631454,
-1.38779958333208));
#77988=CARTESIAN_POINT('Ctrl Pts',(-0.176007588422428,0.158977983578156,
-1.38785569687315));
#77989=CARTESIAN_POINT('Ctrl Pts',(-0.174773130939952,0.160335090865518,
-1.38797910570813));
#77990=CARTESIAN_POINT('Ctrl Pts',(-0.174092819169678,0.161073520688348,
-1.38804629044477));
#77991=CARTESIAN_POINT('Ctrl Pts',(-0.172077662852082,0.163233146174379,
-1.38824296496984));
#77992=CARTESIAN_POINT('Ctrl Pts',(-0.170729922179254,0.164642267773295,
-1.38837153032768));
#77993=CARTESIAN_POINT('Ctrl Pts',(-0.160675323670463,0.174898536419804,
-1.38931052972371));
#77994=CARTESIAN_POINT('Ctrl Pts',(-0.151302082296147,0.183067800070646,
-1.39007706394631));
#77995=CARTESIAN_POINT('Ctrl Pts',(-0.12700778539669,0.201094815634018,
-1.39193486728141));
#77996=CARTESIAN_POINT('Ctrl Pts',(-0.111532908806243,0.210072455227272,
-1.39301956879735));
#77997=CARTESIAN_POINT('Ctrl Pts',(-0.0924504341320403,0.218435120028361,
-1.39436378176224));
#77998=CARTESIAN_POINT('Ctrl Pts',(-0.0896796213965928,0.219587223322597,
-1.3945589588842));
#77999=CARTESIAN_POINT('Ctrl Pts',(-0.0851459530671215,0.221372201549348,
-1.39487873152857));
#78000=CARTESIAN_POINT('Ctrl Pts',(-0.0833960972814792,0.22203732921867,
-1.39500225239986));
#78001=CARTESIAN_POINT('Ctrl Pts',(-0.0802503654460852,0.223190603902801,
-1.39522457474318));
#78002=CARTESIAN_POINT('Ctrl Pts',(-0.0788574372384819,0.223686546863685,
-1.39532311168139));
#78003=CARTESIAN_POINT('Ctrl Pts',(-0.075882460446758,0.224714526803235,
-1.39553380579502));
#78004=CARTESIAN_POINT('Ctrl Pts',(-0.0742992573673935,0.225242949873987,
-1.39564607589331));
#78005=CARTESIAN_POINT('Ctrl Pts',(-0.0699825768934366,0.226633258658918,
-1.39595264325985));
#78006=CARTESIAN_POINT('Ctrl Pts',(-0.067238917008975,0.227462352465796,
-1.39614799367707));
#78007=CARTESIAN_POINT('Ctrl Pts',(-0.0611085656142311,0.229194251556927,
-1.39658576016739));
#78008=CARTESIAN_POINT('Ctrl Pts',(-0.057715581113362,0.23007210007809,
-1.39682891304125));
#78009=CARTESIAN_POINT('Ctrl Pts',(-0.0502043344891319,0.23183883889443,
-1.39736916411075));
#78010=CARTESIAN_POINT('Ctrl Pts',(-0.0460799619130002,0.232693673874856,
-1.39766710396681));
#78011=CARTESIAN_POINT('Ctrl Pts',(-0.0419358227397264,0.233438144689642,
-1.39796759050954));
#78012=CARTESIAN_POINT('',(-0.236838115873986,0.000105245926622949,-1.39566205967354));
#78013=CARTESIAN_POINT('Ctrl Pts',(-0.0420041065163025,0.233814670441123,
-1.41782827198422));
#78014=CARTESIAN_POINT('Ctrl Pts',(-0.117770216984918,0.220073149264774,
-1.41263777999286));
#78015=CARTESIAN_POINT('Ctrl Pts',(-0.215515586929785,0.143319562669835,
-1.40524805039436));
#78016=CARTESIAN_POINT('Ctrl Pts',(-0.23696289445876,0.0329890296572519,
-1.39785832079586));
#78017=CARTESIAN_POINT('Ctrl Pts',(-0.236832944309853,0.000105455023683012,
-1.39565908318872));
#78018=CARTESIAN_POINT('Ctrl Pts',(-0.237174982301523,9.16257185350831E-5,
-1.39585594256495));
#78019=CARTESIAN_POINT('Ctrl Pts',(-0.237175795591863,-0.00201359239129307,
-1.39572069814429));
#78020=CARTESIAN_POINT('Ctrl Pts',(-0.237148579287857,-0.00411868598000703,
-1.39558469481686));
#78021=CARTESIAN_POINT('Ctrl Pts',(-0.237045465987812,-0.00804719088092806,
-1.39532926879552));
#78022=CARTESIAN_POINT('Ctrl Pts',(-0.236976540307452,-0.00987062676514676,
-1.39521006031992));
#78023=CARTESIAN_POINT('Ctrl Pts',(-0.236813981095099,-0.0131638744504354,
-1.39499348396549));
#78024=CARTESIAN_POINT('Ctrl Pts',(-0.236727683409255,-0.0146339665759775,
-1.39489634447685));
#78025=CARTESIAN_POINT('Ctrl Pts',(-0.236532434782362,-0.0175030501932012,
-1.39470581431299));
#78026=CARTESIAN_POINT('Ctrl Pts',(-0.236424747294716,-0.0189020684782139,
-1.39461246665617));
#78027=CARTESIAN_POINT('Ctrl Pts',(-0.236170031794636,-0.0218671122183269,
-1.39441365117725));
#78028=CARTESIAN_POINT('Ctrl Pts',(-0.23601982691454,-0.0234327892487353,
-1.39430808836039));
#78029=CARTESIAN_POINT('Ctrl Pts',(-0.235599560070182,-0.0273981586514169,
-1.39403920592918));
#78030=CARTESIAN_POINT('Ctrl Pts',(-0.235308406271673,-0.0297953854104867,
-1.39387523499128));
#78031=CARTESIAN_POINT('Ctrl Pts',(-0.233995106208499,-0.0393829120711009,
-1.39321351841015));
#78032=CARTESIAN_POINT('Ctrl Pts',(-0.232679643410945,-0.0465283554801728,
-1.39270677819602));
#78033=CARTESIAN_POINT('Ctrl Pts',(-0.226771417425548,-0.0719945443090971,
-1.39085145013459));
#78034=CARTESIAN_POINT('Ctrl Pts',(-0.220323080727087,-0.0898114322158612,
-1.38945327950828));
#78035=CARTESIAN_POINT('Ctrl Pts',(-0.209863928409587,-0.11058151213702,
-1.38777817708755));
#78036=CARTESIAN_POINT('Ctrl Pts',(-0.207787332795316,-0.114435868906816,
-1.38746562333672));
#78037=CARTESIAN_POINT('Ctrl Pts',(-0.204158098086563,-0.120747164986921,
-1.38695338834692));
#78038=CARTESIAN_POINT('Ctrl Pts',(-0.202664906651683,-0.123236943953029,
-1.3867511984491));
#78039=CARTESIAN_POINT('Ctrl Pts',(-0.200503856833246,-0.126694764578667,
-1.38647088306876));
#78040=CARTESIAN_POINT('Ctrl Pts',(-0.199874007993179,-0.127686103590465,
-1.38639057583588));
#78041=CARTESIAN_POINT('Ctrl Pts',(-0.198779900430429,-0.129380219067176,
-1.38625349162518));
#78042=CARTESIAN_POINT('Ctrl Pts',(-0.198319220977252,-0.130085266592673,
-1.38619648823444));
#78043=CARTESIAN_POINT('Ctrl Pts',(-0.197337523094531,-0.131570370726676,
-1.3860765347672));
#78044=CARTESIAN_POINT('Ctrl Pts',(-0.196815621810583,-0.132349807561635,
-1.38601364345898));
#78045=CARTESIAN_POINT('Ctrl Pts',(-0.195370665223989,-0.134480337425429,
-1.38584185237002));
#78046=CARTESIAN_POINT('Ctrl Pts',(-0.194438210913681,-0.135825036305808,
-1.38573355588428));
#78047=CARTESIAN_POINT('Ctrl Pts',(-0.189359997957431,-0.142988880159454,
-1.38515668575407));
#78048=CARTESIAN_POINT('Ctrl Pts',(-0.184966395026557,-0.148628672811585,
-1.38470277128628));
#78049=CARTESIAN_POINT('Ctrl Pts',(-0.171025782779141,-0.164945692672423,
-1.3833615865507));
#78050=CARTESIAN_POINT('Ctrl Pts',(-0.160760697703925,-0.174965508282461,
-1.38249770756623));
#78051=CARTESIAN_POINT('Ctrl Pts',(-0.144191356434958,-0.188442089055549,
-1.38117532017615));
#78052=CARTESIAN_POINT('Ctrl Pts',(-0.138533517504667,-0.192639616371909,
-1.38073489731501));
#78053=CARTESIAN_POINT('Ctrl Pts',(-0.128693970697739,-0.199281649724844,
-1.37997814834188));
#78054=CARTESIAN_POINT('Ctrl Pts',(-0.124608921676507,-0.201861154109281,
-1.3796664932836));
#78055=CARTESIAN_POINT('Ctrl Pts',(-0.118695529821715,-0.205347245374128,
-1.37921713526175));
#78056=CARTESIAN_POINT('Ctrl Pts',(-0.116929702195988,-0.206357854953375,
-1.37908317397037));
#78057=CARTESIAN_POINT('Ctrl Pts',(-0.113839706381855,-0.20807391034005,
-1.37884902382019));
#78058=CARTESIAN_POINT('Ctrl Pts',(-0.112521422928308,-0.208789750992499,
-1.37874921160514));
#78059=CARTESIAN_POINT('Ctrl Pts',(-0.109960056442997,-0.210149294559195,
-1.37855539675321));
#78060=CARTESIAN_POINT('Ctrl Pts',(-0.108717887783892,-0.21079459373373,
-1.37846145563664));
#78061=CARTESIAN_POINT('Ctrl Pts',(-0.105394781135523,-0.212483741716781,
-1.37821023691871));
#78062=CARTESIAN_POINT('Ctrl Pts',(-0.103304107563149,-0.213507988314395,
-1.37805228603065));
#78063=CARTESIAN_POINT('Ctrl Pts',(-0.0953664499642538,-0.217252866477978,
-1.3774527689252));
#78064=CARTESIAN_POINT('Ctrl Pts',(-0.0894248714691551,-0.219765207759282,
-1.37700426445785));
#78065=CARTESIAN_POINT('Ctrl Pts',(-0.0683516447625824,-0.227679694220197,
-1.37541386197654));
#78066=CARTESIAN_POINT('Ctrl Pts',(-0.0527810137464234,-0.23178447326964,
-1.37423581249133));
#78067=CARTESIAN_POINT('Ctrl Pts',(-0.0301738899954698,-0.235346815644265,
-1.37256974293882));
#78068=CARTESIAN_POINT('Ctrl Pts',(-0.0233870183136434,-0.236117865204951,
-1.37207572631368));
#78069=CARTESIAN_POINT('Ctrl Pts',(-0.0139107578500921,-0.236781776307064,
-1.37140153904671));
#78070=CARTESIAN_POINT('Ctrl Pts',(-0.0112424714038401,-0.236923462113636,
-1.37121342717392));
#78071=CARTESIAN_POINT('Ctrl Pts',(-0.00656159139933815,-0.237092754332976,
-1.37088706128202));
#78072=CARTESIAN_POINT('Ctrl Pts',(-0.00455001009005155,-0.237139888496981,
-1.37074798185936));
#78073=CARTESIAN_POINT('Ctrl Pts',(-0.00152161308756375,-0.237172296994421,
-1.37054060383575));
#78074=CARTESIAN_POINT('Ctrl Pts',(-0.000505151697553854,-0.237176640261484,
-1.37047133843824));
#78075=CARTESIAN_POINT('Ctrl Pts',(0.00134100771431228,-0.237172660086146,
-1.37034618890469));
#78076=CARTESIAN_POINT('Ctrl Pts',(0.00217065689784853,-0.237166518062558,
-1.37029019138569));
#78077=CARTESIAN_POINT('Ctrl Pts',(0.00405295482133211,-0.237142704808126,
-1.37016368956015));
#78078=CARTESIAN_POINT('Ctrl Pts',(0.00510553519943075,-0.23712237874548,
-1.37009333139362));
#78079=CARTESIAN_POINT('Ctrl Pts',(0.00835567896387067,-0.23703796412398,
-1.36987716249979));
#78080=CARTESIAN_POINT('Ctrl Pts',(0.0105525843125146,-0.236950327318595,
-1.36973257317255));
#78081=CARTESIAN_POINT('Ctrl Pts',(0.0273038899655948,-0.236048648851461,
-1.36863958271983));
#78082=CARTESIAN_POINT('Ctrl Pts',(0.0417585545839553,-0.233924785151911,
-1.36774993578599));
#78083=CARTESIAN_POINT('Ctrl Pts',(0.0715141225821607,-0.226704509336095,
-1.36587224954963));
#78084=CARTESIAN_POINT('Ctrl Pts',(0.086674210281199,-0.221351982902229,
-1.36488651062116));
#78085=CARTESIAN_POINT('Ctrl Pts',(0.103792165335796,-0.213278045697669,
-1.36366019814956));
#78086=CARTESIAN_POINT('Ctrl Pts',(0.106384023197842,-0.211997115050351,
-1.36347138073069));
#78087=CARTESIAN_POINT('Ctrl Pts',(0.110438665317319,-0.209900176644186,
-1.36317064796775));
#78088=CARTESIAN_POINT('Ctrl Pts',(0.111917382467928,-0.20911547578414,
-1.36305982543613));
#78089=CARTESIAN_POINT('Ctrl Pts',(0.114685203164893,-0.207608928758897,
-1.36285015616172));
#78090=CARTESIAN_POINT('Ctrl Pts',(0.115976115328242,-0.206890559545931,
-1.36275143650084));
#78091=CARTESIAN_POINT('Ctrl Pts',(0.118879401727701,-0.205239222476864,
-1.3625272560819));
#78092=CARTESIAN_POINT('Ctrl Pts',(0.120487648312623,-0.20429923362212,
-1.36240154759485));
#78093=CARTESIAN_POINT('Ctrl Pts',(0.125371833381066,-0.201366792257235,
-1.36201498170954));
#78094=CARTESIAN_POINT('Ctrl Pts',(0.128610530848772,-0.199313848033501,
-1.36175195100742));
#78095=CARTESIAN_POINT('Ctrl Pts',(0.147408743599202,-0.186749074880236,
-1.36018431420591));
#78096=CARTESIAN_POINT('Ctrl Pts',(0.161722856494158,-0.174499367397765,
-1.35881371746332));
#78097=CARTESIAN_POINT('Ctrl Pts',(0.181297658453648,-0.153250026796478,
-1.35670728516821));
#78098=CARTESIAN_POINT('Ctrl Pts',(0.187672041552431,-0.145374193498671,
-1.35597377334996));
#78099=CARTESIAN_POINT('Ctrl Pts',(0.194852651797957,-0.135239436809794,
-1.35510534651962));
#78100=CARTESIAN_POINT('Ctrl Pts',(0.196153871236581,-0.133345119725638,
-1.35494607119793));
#78101=CARTESIAN_POINT('Ctrl Pts',(0.198021123735284,-0.130540273619924,
-1.35471499893364));
#78102=CARTESIAN_POINT('Ctrl Pts',(0.198608801361587,-0.129644408345657,
-1.35464189361358));
#78103=CARTESIAN_POINT('Ctrl Pts',(0.199598156337058,-0.128113702891585,
-1.35451820835669));
#78104=CARTESIAN_POINT('Ctrl Pts',(0.200002914161758,-0.127480897653863,
-1.35446742993155));
#78105=CARTESIAN_POINT('Ctrl Pts',(0.200921251712227,-0.126030012967184,
-1.35435181902011));
#78106=CARTESIAN_POINT('Ctrl Pts',(0.201432848084865,-0.125210707821098,
-1.35428711566809));
#78107=CARTESIAN_POINT('Ctrl Pts',(0.202840876952476,-0.122924828870483,
-1.35410813463067));
#78108=CARTESIAN_POINT('Ctrl Pts',(0.203726414729484,-0.12145156762085,
-1.35399453117514));
#78109=CARTESIAN_POINT('Ctrl Pts',(0.210226453817895,-0.110366337578196,
-1.35315173395839));
#78110=CARTESIAN_POINT('Ctrl Pts',(0.215174792269841,-0.100378106010538,
-1.35245881617375));
#78111=CARTESIAN_POINT('Ctrl Pts',(0.222782022996827,-0.0818491244441361,
-1.35122523740475));
#78112=CARTESIAN_POINT('Ctrl Pts',(0.225694831281892,-0.0734367244527316,
-1.3506829883356));
#78113=CARTESIAN_POINT('Ctrl Pts',(0.230261477039953,-0.0573798313792536,
-1.34965285573392));
#78114=CARTESIAN_POINT('Ctrl Pts',(0.232023358021294,-0.0497789178323422,
-1.34916719705328));
#78115=CARTESIAN_POINT('Ctrl Pts',(0.234035136962451,-0.038626802490816,
-1.34844661960073));
#78116=CARTESIAN_POINT('Ctrl Pts',(0.234584790326267,-0.0351347325073054,
-1.34821989688206));
#78117=CARTESIAN_POINT('Ctrl Pts',(0.235440978611729,-0.02877239247986,
-1.34780391957597));
#78118=CARTESIAN_POINT('Ctrl Pts',(0.235773551713395,-0.0259062949418869,
-1.34761547137768));
#78119=CARTESIAN_POINT('Ctrl Pts',(0.236216212096634,-0.0213700714723223,
-1.34731519281886));
#78120=CARTESIAN_POINT('Ctrl Pts',(0.236361054432868,-0.0197035661360794,
-1.34720444959608));
#78121=CARTESIAN_POINT('Ctrl Pts',(0.236600606918957,-0.0165624993218356,
-1.34699484829193));
#78122=CARTESIAN_POINT('Ctrl Pts',(0.236699189686879,-0.0150883070682883,
-1.34689611638911));
#78123=CARTESIAN_POINT('Ctrl Pts',(0.23689101747421,-0.0117517399937514,
-1.3466717958064));
#78124=CARTESIAN_POINT('Ctrl Pts',(0.236976084545565,-0.00988901217047821,
-1.34654595812243));
#78125=CARTESIAN_POINT('Ctrl Pts',(0.237169259861288,-0.00418344827775827,
-1.34615856922182));
#78126=CARTESIAN_POINT('Ctrl Pts',(0.237205904563023,-0.000338989302938372,
-1.34589483111555));
#78127=CARTESIAN_POINT('Ctrl Pts',(0.236871841173798,0.0222671988442763,
-1.34432720994275));
#78128=CARTESIAN_POINT('Ctrl Pts',(0.234368863128452,0.040927873908069,
-1.34295747228143));
#78129=CARTESIAN_POINT('Ctrl Pts',(0.227174308725929,0.0688924206830977,
-1.34085223027819));
#78130=CARTESIAN_POINT('Ctrl Pts',(0.224029002892859,0.0785199187998523,
-1.34011901554371));
#78131=CARTESIAN_POINT('Ctrl Pts',(0.219426395991204,0.0900517411378575,
-1.3392508963785));
#78132=CARTESIAN_POINT('Ctrl Pts',(0.218543722445539,0.092173215703996,
-1.33909164955469));
#78133=CARTESIAN_POINT('Ctrl Pts',(0.217204453602668,0.0952646506539745,
-1.33886061031242));
#78134=CARTESIAN_POINT('Ctrl Pts',(0.216771921517342,0.0962448049618629,
-1.3387875100461));
#78135=CARTESIAN_POINT('Ctrl Pts',(0.216024834939209,0.0979071783471902,
-1.33866382986567));
#78136=CARTESIAN_POINT('Ctrl Pts',(0.215713662010635,0.0985908766693289,
-1.33861305152136));
#78137=CARTESIAN_POINT('Ctrl Pts',(0.214994913400916,0.10015039153322,-1.33849743543056));
#78138=CARTESIAN_POINT('Ctrl Pts',(0.21458522999125,0.101025209055305,-1.3384327268686));
#78139=CARTESIAN_POINT('Ctrl Pts',(0.213431628067686,0.103449872220064,
-1.33825372142323));
#78140=CARTESIAN_POINT('Ctrl Pts',(0.212676169725761,0.104994205427463,
-1.33814009902433));
#78141=CARTESIAN_POINT('Ctrl Pts',(0.206890292448835,0.116503146728735,
-1.3372952683115));
#78142=CARTESIAN_POINT('Ctrl Pts',(0.20117814328167,0.126111048115842,-1.33660053908841));
#78143=CARTESIAN_POINT('Ctrl Pts',(0.189763808172186,0.142548011093985,
-1.3353681695696));
#78144=CARTESIAN_POINT('Ctrl Pts',(0.184315403321145,0.14952615434846,-1.33482887280208));
#78145=CARTESIAN_POINT('Ctrl Pts',(0.173347475914995,0.16206053202378,-1.3338011356029));
#78146=CARTESIAN_POINT('Ctrl Pts',(0.167918253949125,0.167679485535629,
-1.33331482406106));
#78147=CARTESIAN_POINT('Ctrl Pts',(0.159641141388833,0.175440028456389,
-1.33259337360236));
#78148=CARTESIAN_POINT('Ctrl Pts',(0.157006486954748,0.177801739966896,
-1.33236645395149));
#78149=CARTESIAN_POINT('Ctrl Pts',(0.15212762339867,0.181982149874415,-1.33195014815748));
#78150=CARTESIAN_POINT('Ctrl Pts',(0.149901115409691,0.183820486064305,
-1.33176157038228));
#78151=CARTESIAN_POINT('Ctrl Pts',(0.146332174026146,0.186659248869644,
-1.33146113083248));
#78152=CARTESIAN_POINT('Ctrl Pts',(0.145011711086444,0.187686930153582,
-1.3313503581488));
#78153=CARTESIAN_POINT('Ctrl Pts',(0.142505016609965,0.189595579503373,
-1.3311407288982));
#78154=CARTESIAN_POINT('Ctrl Pts',(0.141321206011921,0.190479605438435,
-1.3310419988192));
#78155=CARTESIAN_POINT('Ctrl Pts',(0.138625310871336,0.192453834847101,
-1.33081772036805));
#78156=CARTESIAN_POINT('Ctrl Pts',(0.137108492871284,0.193537376751465,
-1.33069192341743));
#78157=CARTESIAN_POINT('Ctrl Pts',(0.133138619880586,0.196303172093216,
-1.33036360778821));
#78158=CARTESIAN_POINT('Ctrl Pts',(0.130666475369076,0.197957314342616,
-1.33016005360139));
#78159=CARTESIAN_POINT('Ctrl Pts',(0.110219399975613,0.211088802328886,
-1.32848306639413));
#78160=CARTESIAN_POINT('Ctrl Pts',(0.0908051149535009,0.220138292566319,
-1.32691880170839));
#78161=CARTESIAN_POINT('Ctrl Pts',(0.064329074535868,0.228374325356081,
-1.3249025942938));
#78162=CARTESIAN_POINT('Ctrl Pts',(0.0581337950144433,0.230029420994305,
-1.32443965199956));
#78163=CARTESIAN_POINT('Ctrl Pts',(0.0493729297070068,0.231993295038763,
-1.32380321942766));
#78164=CARTESIAN_POINT('Ctrl Pts',(0.0468580686445437,0.232514295676086,
-1.32362260612725));
#78165=CARTESIAN_POINT('Ctrl Pts',(0.0424176602872986,0.233359234992425,
-1.32330789890318));
#78166=CARTESIAN_POINT('Ctrl Pts',(0.0404956762459849,0.233700430637499,
-1.32317305426759));
#78167=CARTESIAN_POINT('Ctrl Pts',(0.0375786990151602,0.234181191834915,
-1.32297069405255));
#78168=CARTESIAN_POINT('Ctrl Pts',(0.0365867245435667,0.234338219052782,
-1.32290227740962));
#78169=CARTESIAN_POINT('Ctrl Pts',(0.034772901804239,0.234613544490767,
-1.32277794397236));
#78170=CARTESIAN_POINT('Ctrl Pts',(0.0339514116270074,0.234733831496263,
-1.32272192279748));
#78171=CARTESIAN_POINT('Ctrl Pts',(0.0320728370872758,0.2349988340294,-1.32259446548958));
#78172=CARTESIAN_POINT('Ctrl Pts',(0.0310153901569653,0.235140733511951,
-1.32252318561633));
#78173=CARTESIAN_POINT('Ctrl Pts',(0.027701533066287,0.235562678027431,
-1.32230116156725));
#78174=CARTESIAN_POINT('Ctrl Pts',(0.0254419549091784,0.235817425295826,
-1.32215173598909));
#78175=CARTESIAN_POINT('Ctrl Pts',(0.0100281099386102,0.237331056319137,
-1.32114362932619));
#78176=CARTESIAN_POINT('Ctrl Pts',(-0.0032094353065917,0.23752133059925,
-1.32033253787148));
#78177=CARTESIAN_POINT('Ctrl Pts',(-0.0249624680853009,0.236013991717859,
-1.31899503856155));
#78178=CARTESIAN_POINT('Ctrl Pts',(-0.0334885117149788,0.234955656011327,
-1.31846975277959));
#78179=CARTESIAN_POINT('Ctrl Pts',(-0.0419358330286197,0.233438142841301,
-1.31793598285019));
#78180=CARTESIAN_POINT('Origin',(0.,0.,-1.7456589891905));
#78181=CARTESIAN_POINT('',(-0.0419358257152316,0.23343814415511,-1.19832585242651));
#78182=CARTESIAN_POINT('',(-0.0419358439263085,0.233438140883593,-1.21800162451869));
#78183=CARTESIAN_POINT('',(-0.0419358257166344,0.233438144154858,-1.7456589891905));
#78184=CARTESIAN_POINT('',(-0.237174995128926,4.80686365711195E-5,-1.27615111301349));
#78185=CARTESIAN_POINT('Ctrl Pts',(-0.0419358257152316,0.23343814415511,
-1.19832585242651));
#78186=CARTESIAN_POINT('Ctrl Pts',(-0.0396781609992177,0.233843720691884,
-1.19847529274218));
#78187=CARTESIAN_POINT('Ctrl Pts',(-0.0374146269178974,0.234216542598402,
-1.19862326078251));
#78188=CARTESIAN_POINT('Ctrl Pts',(-0.0285556537828558,0.235543970926263,
-1.19919637462169));
#78189=CARTESIAN_POINT('Ctrl Pts',(-0.0219262080047059,0.236253341205789,
-1.19961236340081));
#78190=CARTESIAN_POINT('Ctrl Pts',(0.000180787645325519,0.237680105942458,
-1.2009818499977));
#78191=CARTESIAN_POINT('Ctrl Pts',(0.0156969032840805,0.237161270717864,
-1.20191685478394));
#78192=CARTESIAN_POINT('Ctrl Pts',(0.0380990898538144,0.234202844417619,
-1.20333619123462));
#78193=CARTESIAN_POINT('Ctrl Pts',(0.0451005198850373,0.232955878672664,
-1.20378943582846));
#78194=CARTESIAN_POINT('Ctrl Pts',(0.0543769107165645,0.230869864715835,
-1.20440883861378));
#78195=CARTESIAN_POINT('Ctrl Pts',(0.0567106868691924,0.230307707554651,
-1.20456627927336));
#78196=CARTESIAN_POINT('Ctrl Pts',(0.0605563704476955,0.229319368069006,
-1.20482858574294));
#78197=CARTESIAN_POINT('Ctrl Pts',(0.062073328870888,0.228913407679896,
-1.20493279935709));
#78198=CARTESIAN_POINT('Ctrl Pts',(0.0650426259917649,0.228087095526861,
-1.20513830687406));
#78199=CARTESIAN_POINT('Ctrl Pts',(0.0664951993510447,0.227667860320054,
-1.20523956031059));
#78200=CARTESIAN_POINT('Ctrl Pts',(0.0699577076530744,0.22663256364463,
-1.20548269202567));
#78201=CARTESIAN_POINT('Ctrl Pts',(0.0719636244782297,0.226003619488697,
-1.20562498324758));
#78202=CARTESIAN_POINT('Ctrl Pts',(0.0789697688816637,0.223704152810454,
-1.20612718131918));
#78203=CARTESIAN_POINT('Ctrl Pts',(0.0839221005964498,0.221893771513249,
-1.20649159192433));
#78204=CARTESIAN_POINT('Ctrl Pts',(0.096219655637753,0.216927684324084,
-1.20742101708266));
#78205=CARTESIAN_POINT('Ctrl Pts',(0.103472982827372,0.213563019050453,
-1.20799206242827));
#78206=CARTESIAN_POINT('Ctrl Pts',(0.124003784272244,0.202747499575129,
-1.20967050781545));
#78207=CARTESIAN_POINT('Ctrl Pts',(0.136751505430185,0.194377234375328,
-1.21079432348841));
#78208=CARTESIAN_POINT('Ctrl Pts',(0.152498099546546,0.181717375441858,
-1.21223908776855));
#78209=CARTESIAN_POINT('Ctrl Pts',(0.156287340208863,0.17846890581939,-1.21259138963));
#78210=CARTESIAN_POINT('Ctrl Pts',(0.161061041561957,0.174107722894649,
-1.21303844816714));
#78211=CARTESIAN_POINT('Ctrl Pts',(0.162141243888337,0.173102211390518,
-1.21313983170415));
#78212=CARTESIAN_POINT('Ctrl Pts',(0.163867309392779,0.171465160271841,
-1.2133020940107));
#78213=CARTESIAN_POINT('Ctrl Pts',(0.164519052923484,0.170839917960272,
-1.21336342353618));
#78214=CARTESIAN_POINT('Ctrl Pts',(0.165783615616239,0.169612827095649,
-1.21348251108903));
#78215=CARTESIAN_POINT('Ctrl Pts',(0.166396759807231,0.169011350738139,
-1.21354029273356));
#78216=CARTESIAN_POINT('Ctrl Pts',(0.16790662167669,0.167514039943685,-1.21368271905115));
#78217=CARTESIAN_POINT('Ctrl Pts',(0.168799468252138,0.166614305738228,
-1.21376706593619));
#78218=CARTESIAN_POINT('Ctrl Pts',(0.172162588837373,0.163170456603198,
-1.21408546098894));
#78219=CARTESIAN_POINT('Ctrl Pts',(0.174583046748999,0.16057807416605,-1.21431603071219));
#78220=CARTESIAN_POINT('Ctrl Pts',(0.180827942886438,0.153581397585631,
-1.21491789466115));
#78221=CARTESIAN_POINT('Ctrl Pts',(0.184549753430381,0.149088524521435,
-1.21528393254017));
#78222=CARTESIAN_POINT('Ctrl Pts',(0.198842250592816,0.130478517010214,
-1.21674085061775));
#78223=CARTESIAN_POINT('Ctrl Pts',(0.207988984039867,0.115340697901134,
-1.21779952652288));
#78224=CARTESIAN_POINT('Ctrl Pts',(0.218050138073271,0.0935252025029785,
-1.21931445631422));
#78225=CARTESIAN_POINT('Ctrl Pts',(0.220490833630498,0.0876162512605708,
-1.21972326080672));
#78226=CARTESIAN_POINT('Ctrl Pts',(0.223488593765181,0.0794368752657272,
-1.22029131915498));
#78227=CARTESIAN_POINT('Ctrl Pts',(0.224255306812717,0.0772458765030693,
-1.22044367973588));
#78228=CARTESIAN_POINT('Ctrl Pts',(0.225432292397446,0.0737171531548524,
-1.22068954780572));
#78229=CARTESIAN_POINT('Ctrl Pts',(0.225863112793076,0.0723864024691382,
-1.22078237794979));
#78230=CARTESIAN_POINT('Ctrl Pts',(0.226731882117881,0.0696195960241475,
-1.2209756485522));
#78231=CARTESIAN_POINT('Ctrl Pts',(0.227168015633163,0.0681830405171525,
-1.22107614331163));
#78232=CARTESIAN_POINT('Ctrl Pts',(0.228164627734883,0.0647846133648534,
-1.22131427371725));
#78233=CARTESIAN_POINT('Ctrl Pts',(0.228713478585986,0.0628194853493693,
-1.22145227851539));
#78234=CARTESIAN_POINT('Ctrl Pts',(0.230485094021345,0.0561451087257307,
-1.22192216362513));
#78235=CARTESIAN_POINT('Ctrl Pts',(0.231588217714727,0.0514056731071655,
-1.22225780712472));
#78236=CARTESIAN_POINT('Ctrl Pts',(0.233943604620991,0.0396608104487631,
-1.22309490510922));
#78237=CARTESIAN_POINT('Ctrl Pts',(0.235027791857391,0.0326268514051426,
-1.22360093432746));
#78238=CARTESIAN_POINT('Ctrl Pts',(0.237333114580107,0.0113560769014225,
-1.22514186521636));
#78239=CARTESIAN_POINT('Ctrl Pts',(0.237586244616119,-0.00295234577984794,
-1.22619448580137));
#78240=CARTESIAN_POINT('Ctrl Pts',(0.236038644205291,-0.0242411332845506,
-1.22773612715121));
#78241=CARTESIAN_POINT('Ctrl Pts',(0.235211990319785,-0.0312604157511371,
-1.228239924464));
#78242=CARTESIAN_POINT('Ctrl Pts',(0.233809942409609,-0.0398441548554468,
-1.22884277936169));
#78243=CARTESIAN_POINT('Ctrl Pts',(0.233530135095655,-0.0414526503106507,
-1.22895516511401));
#78244=CARTESIAN_POINT('Ctrl Pts',(0.233063559042569,-0.0439799579232817,
-1.22913069694454));
#78245=CARTESIAN_POINT('Ctrl Pts',(0.232887919902086,-0.0449007359914931,
-1.22919442812406));
#78246=CARTESIAN_POINT('Ctrl Pts',(0.232543988369845,-0.0466474491284448,
-1.22931487556662));
#78247=CARTESIAN_POINT('Ctrl Pts',(0.232376751692154,-0.0474735329551559,
-1.22937164375206));
#78248=CARTESIAN_POINT('Ctrl Pts',(0.231965421994281,-0.0494510762804358,
-1.22950709969876));
#78249=CARTESIAN_POINT('Ctrl Pts',(0.231717155560191,-0.0506016393946176,
-1.22958555358991));
#78250=CARTESIAN_POINT('Ctrl Pts',(0.230823825842356,-0.0545971764997261,
-1.2298569094147));
#78251=CARTESIAN_POINT('Ctrl Pts',(0.230134820968382,-0.0574321887449935,
-1.23004752217888));
#78252=CARTESIAN_POINT('Ctrl Pts',(0.22827411595513,-0.0645161081842341,
-1.23052061758942));
#78253=CARTESIAN_POINT('Ctrl Pts',(0.227035944427103,-0.0687465254732881,
-1.23080023310318));
#78254=CARTESIAN_POINT('Ctrl Pts',(0.222273633360089,-0.0834813442281059,
-1.23177167822095));
#78255=CARTESIAN_POINT('Ctrl Pts',(0.218132219259187,-0.0937713298240962,
-1.23244611814119));
#78256=CARTESIAN_POINT('Ctrl Pts',(0.207037229656744,-0.116583512461436,
-1.23400373231551));
#78257=CARTESIAN_POINT('Ctrl Pts',(0.19964055612945,-0.12883983746124,-1.2348887813357));
#78258=CARTESIAN_POINT('Ctrl Pts',(0.189542776674368,-0.142594647040605,
-1.23599567394002));
#78259=CARTESIAN_POINT('Ctrl Pts',(0.187859694490644,-0.144804805473468,
-1.23617727155203));
#78260=CARTESIAN_POINT('Ctrl Pts',(0.185115468171708,-0.148280031353603,
-1.23646916200283));
#78261=CARTESIAN_POINT('Ctrl Pts',(0.184079230590837,-0.149564504104685,
-1.23657847151481));
#78262=CARTESIAN_POINT('Ctrl Pts',(0.182087198706978,-0.151981672928404,
-1.23678696265033));
#78263=CARTESIAN_POINT('Ctrl Pts',(0.18113402392114,-0.153116432971608,
-1.23688603539549));
#78264=CARTESIAN_POINT('Ctrl Pts',(0.178932137356722,-0.155688457006322,
-1.23711338811316));
#78265=CARTESIAN_POINT('Ctrl Pts',(0.177676641527493,-0.157119750867539,
-1.23724194340613));
#78266=CARTESIAN_POINT('Ctrl Pts',(0.173692669004136,-0.16155275138188,
-1.23764665003713));
#78267=CARTESIAN_POINT('Ctrl Pts',(0.170904458612851,-0.164499535765807,
-1.23792528219711));
#78268=CARTESIAN_POINT('Ctrl Pts',(0.160691626878338,-0.174753187207367,
-1.23893046668008));
#78269=CARTESIAN_POINT('Ctrl Pts',(0.152863790928762,-0.181639996328916,
-1.23967383213728));
#78270=CARTESIAN_POINT('Ctrl Pts',(0.130141413392986,-0.199119037405477,
-1.24175106382711));
#78271=CARTESIAN_POINT('Ctrl Pts',(0.114436554812705,-0.208541362291877,
-1.24310518124741));
#78272=CARTESIAN_POINT('Ctrl Pts',(0.095781807183824,-0.216985628947662,
-1.24453562220305));
#78273=CARTESIAN_POINT('Ctrl Pts',(0.0937447002829357,-0.217873472025179,
-1.24468952566214));
#78274=CARTESIAN_POINT('Ctrl Pts',(0.0907201799775787,-0.219141387224933,
-1.24491434186391));
#78275=CARTESIAN_POINT('Ctrl Pts',(0.0897422860112767,-0.219543665039204,
-1.24498646761317));
#78276=CARTESIAN_POINT('Ctrl Pts',(0.0879920002586462,-0.220250033971538,
-1.24511451955892));
#78277=CARTESIAN_POINT('Ctrl Pts',(0.0872206674940196,-0.220556624928486,
-1.24517058888646));
#78278=CARTESIAN_POINT('Ctrl Pts',(0.0855045201920958,-0.221228351560247,
-1.24529453618946));
#78279=CARTESIAN_POINT('Ctrl Pts',(0.0845589617588538,-0.221591490332732,
-1.24536229706069));
#78280=CARTESIAN_POINT('Ctrl Pts',(0.0817455482092795,-0.222651341986079,
-1.24556242219509));
#78281=CARTESIAN_POINT('Ctrl Pts',(0.0798711502316693,-0.223330595177069,
-1.24569381248973));
#78282=CARTESIAN_POINT('Ctrl Pts',(0.0670709882815222,-0.227787403244509,
-1.24657938012724));
#78283=CARTESIAN_POINT('Ctrl Pts',(0.0558888660593665,-0.230785877723939,
-1.24729587153018));
#78284=CARTESIAN_POINT('Ctrl Pts',(0.0260674725651557,-0.23648644925664,
-1.2491625809012));
#78285=CARTESIAN_POINT('Ctrl Pts',(0.00725152689139191,-0.237808103174622,
-1.25030200564773));
#78286=CARTESIAN_POINT('Ctrl Pts',(-0.0144231909681409,-0.236753851291595,
-1.25170347451265));
#78287=CARTESIAN_POINT('Ctrl Pts',(-0.0173209390168144,-0.236559502945541,
-1.25189251951777));
#78288=CARTESIAN_POINT('Ctrl Pts',(-0.0220513610137182,-0.236154859415893,
-1.252204259333));
#78289=CARTESIAN_POINT('Ctrl Pts',(-0.0238864921757022,-0.23597630245453,
-1.25232596920424));
#78290=CARTESIAN_POINT('Ctrl Pts',(-0.0271867094215329,-0.235616303193861,
-1.25254632757373));
#78291=CARTESIAN_POINT('Ctrl Pts',(-0.0286525506330593,-0.235442542191863,
-1.25264473070611));
#78292=CARTESIAN_POINT('Ctrl Pts',(-0.0317905796184613,-0.235040821231997,
-1.2528565659177));
#78293=CARTESIAN_POINT('Ctrl Pts',(-0.0334621392098675,-0.234808674419038,
-1.25297012457245));
#78294=CARTESIAN_POINT('Ctrl Pts',(-0.0380523415256968,-0.23412117665255,
-1.25328401176368));
#78295=CARTESIAN_POINT('Ctrl Pts',(-0.0409650912407725,-0.233629120585648,
-1.2534854803568));
#78296=CARTESIAN_POINT('Ctrl Pts',(-0.0474481025143045,-0.232408973478222,
-1.25393921657003));
#78297=CARTESIAN_POINT('Ctrl Pts',(-0.0510122458592781,-0.231652761038222,
-1.25419230639155));
#78298=CARTESIAN_POINT('Ctrl Pts',(-0.0625175587552499,-0.228933264878961,
-1.25502127776127));
#78299=CARTESIAN_POINT('Ctrl Pts',(-0.070374328844154,-0.226641382848858,
-1.2556063129692));
#78300=CARTESIAN_POINT('Ctrl Pts',(-0.0942317461438074,-0.218321709650529,
-1.25743530348131));
#78301=CARTESIAN_POINT('Ctrl Pts',(-0.109711641892026,-0.210967685950249,
-1.25870104585965));
#78302=CARTESIAN_POINT('Ctrl Pts',(-0.127042903920494,-0.200306520281306,
-1.26013808603997));
#78303=CARTESIAN_POINT('Ctrl Pts',(-0.129783417054643,-0.198541856370272,
-1.26036580907024));
#78304=CARTESIAN_POINT('Ctrl Pts',(-0.133535341495015,-0.196015027913566,
-1.26067736169793));
#78305=CARTESIAN_POINT('Ctrl Pts',(-0.134578204515581,-0.195300500879943,
-1.26076393511293));
#78306=CARTESIAN_POINT('Ctrl Pts',(-0.136292950973946,-0.194105369206056,
-1.26090617988225));
#78307=CARTESIAN_POINT('Ctrl Pts',(-0.136968114323581,-0.193629539513505,
-1.26096215981674));
#78308=CARTESIAN_POINT('Ctrl Pts',(-0.138350642785387,-0.192644335562723,
-1.26107671087382));
#78309=CARTESIAN_POINT('Ctrl Pts',(-0.139057709045866,-0.192134572631307,
-1.26113525470778));
#78310=CARTESIAN_POINT('Ctrl Pts',(-0.14081623410786,-0.190851962547866,
-1.26128079903513));
#78311=CARTESIAN_POINT('Ctrl Pts',(-0.141864170670573,-0.190074303018333,
-1.26136747885913));
#78312=CARTESIAN_POINT('Ctrl Pts',(-0.144193762320322,-0.188315544821261,
-1.26156018525671));
#78313=CARTESIAN_POINT('Ctrl Pts',(-0.145471939960449,-0.187329924251805,
-1.26166592772791));
#78314=CARTESIAN_POINT('Ctrl Pts',(-0.154678679801214,-0.180079414286266,
-1.26242848356474));
#78315=CARTESIAN_POINT('Ctrl Pts',(-0.162210645187375,-0.17332582669859,
-1.26305741221355));
#78316=CARTESIAN_POINT('Ctrl Pts',(-0.182404828362225,-0.152745308568872,
-1.26483369041657));
#78317=CARTESIAN_POINT('Ctrl Pts',(-0.193889975237656,-0.137874131113492,
-1.26596458683913));
#78318=CARTESIAN_POINT('Ctrl Pts',(-0.205497308366332,-0.118481483010034,
-1.26741587165789));
#78319=CARTESIAN_POINT('Ctrl Pts',(-0.207406101536215,-0.115107392756048,
-1.26766732969837));
#78320=CARTESIAN_POINT('Ctrl Pts',(-0.210112323634053,-0.110037686700223,
-1.26804449435754));
#78321=CARTESIAN_POINT('Ctrl Pts',(-0.210973785933376,-0.10837685339845,
-1.26816794820959));
#78322=CARTESIAN_POINT('Ctrl Pts',(-0.212480665314051,-0.105385641370273,
-1.26839019750658));
#78323=CARTESIAN_POINT('Ctrl Pts',(-0.213133467195466,-0.10405907712203,
-1.26848872913115));
#78324=CARTESIAN_POINT('Ctrl Pts',(-0.214497006196713,-0.101221553519554,
-1.26869946330318));
#78325=CARTESIAN_POINT('Ctrl Pts',(-0.215204271930364,-0.0997090249692457,
-1.26881177926179));
#78326=CARTESIAN_POINT('Ctrl Pts',(-0.21708331623625,-0.095577437704139,
-1.26911860543523));
#78327=CARTESIAN_POINT('Ctrl Pts',(-0.218223601247948,-0.0929444532576411,
-1.26931417181783));
#78328=CARTESIAN_POINT('Ctrl Pts',(-0.225403679924603,-0.0755042268541385,
-1.27061029899731));
#78329=CARTESIAN_POINT('Ctrl Pts',(-0.229979335268381,-0.0601418153635036,
-1.27175967532887));
#78330=CARTESIAN_POINT('Ctrl Pts',(-0.234163398642582,-0.0382065364502483,
-1.27338802391003));
#78331=CARTESIAN_POINT('Ctrl Pts',(-0.235101642518382,-0.0319289118803864,
-1.27385205053657));
#78332=CARTESIAN_POINT('Ctrl Pts',(-0.236713328902362,-0.0170968632199078,
-1.27493628835472));
#78333=CARTESIAN_POINT('Ctrl Pts',(-0.237176733220839,-0.00852783387215598,
-1.27555340593406));
#78334=CARTESIAN_POINT('Ctrl Pts',(-0.237174995128926,4.80686365711195E-5,
-1.27615111301349));
#78335=CARTESIAN_POINT('Ctrl Pts',(-0.23717499508403,4.82896501978278E-5,
-1.27615112841727));
#78336=CARTESIAN_POINT('Ctrl Pts',(-0.237174613853761,0.00192070510180656,
-1.27628162842272));
#78337=CARTESIAN_POINT('Ctrl Pts',(-0.23715205948629,0.00379313235517636,
-1.27641117093985));
#78338=CARTESIAN_POINT('Ctrl Pts',(-0.237086814510887,0.00652386181438924,
-1.27659851217209));
#78339=CARTESIAN_POINT('Ctrl Pts',(-0.237061633173535,0.00738244688167251,
-1.27665718692539));
#78340=CARTESIAN_POINT('Ctrl Pts',(-0.237004606977172,0.00902268439812538,
-1.27676881879035));
#78341=CARTESIAN_POINT('Ctrl Pts',(-0.236973558060478,0.00980435659168084,
-1.27682181816431));
#78342=CARTESIAN_POINT('Ctrl Pts',(-0.236898555557878,0.0114831008895777,
-1.27693519244308));
#78343=CARTESIAN_POINT('Ctrl Pts',(-0.23685337313074,0.0123801024020447,
-1.27699549835875));
#78344=CARTESIAN_POINT('Ctrl Pts',(-0.236721772223277,0.0147273094283117,
-1.27715263780297));
#78345=CARTESIAN_POINT('Ctrl Pts',(-0.236627121583874,0.0161770417608945,
-1.27724902916325));
#78346=CARTESIAN_POINT('Ctrl Pts',(-0.236164586880043,0.022383736471244,
-1.27765921014127));
#78347=CARTESIAN_POINT('Ctrl Pts',(-0.2356665066264,0.0271302153687484,
-1.2779666075352));
#78348=CARTESIAN_POINT('Ctrl Pts',(-0.232710181682495,0.0489393220743692,
-1.27936324243328));
#78349=CARTESIAN_POINT('Ctrl Pts',(-0.228539638905983,0.065717688799441,
-1.28039621453562));
#78350=CARTESIAN_POINT('Ctrl Pts',(-0.220195779911241,0.0883954056428438,
-1.28189321490591));
#78351=CARTESIAN_POINT('Ctrl Pts',(-0.217521450463328,0.0947857440973023,
-1.28232659352862));
#78352=CARTESIAN_POINT('Ctrl Pts',(-0.212537664449414,0.105368452629825,
-1.28307255017715));
#78353=CARTESIAN_POINT('Ctrl Pts',(-0.210373963686022,0.10962463262242,
-1.28338064108519));
#78354=CARTESIAN_POINT('Ctrl Pts',(-0.207111324327873,0.11558972175671,
-1.28382577423364));
#78355=CARTESIAN_POINT('Ctrl Pts',(-0.206116510994967,0.117354454177868,
-1.28395917348986));
#78356=CARTESIAN_POINT('Ctrl Pts',(-0.204346486089286,0.120402413174954,
-1.28419268691012));
#78357=CARTESIAN_POINT('Ctrl Pts',(-0.203581476875947,0.121691452340644,
-1.28429243070438));
#78358=CARTESIAN_POINT('Ctrl Pts',(-0.202077128150336,0.124172387941331,
-1.2844863656046));
#78359=CARTESIAN_POINT('Ctrl Pts',(-0.201339331815747,0.125365150526535,
-1.28458049735977));
#78360=CARTESIAN_POINT('Ctrl Pts',(-0.19934155947504,0.128531733957456,
-1.28483284030694));
#78361=CARTESIAN_POINT('Ctrl Pts',(-0.198062884566006,0.130493513411497,
-1.28499173572442));
#78362=CARTESIAN_POINT('Ctrl Pts',(-0.193092080790156,0.137878459303881,
-1.28559991623431));
#78363=CARTESIAN_POINT('Ctrl Pts',(-0.189204848899054,0.143166099579953,
-1.28605640561929));
#78364=CARTESIAN_POINT('Ctrl Pts',(-0.17512245504322,0.160745064466465,
-1.28764880793862));
#78365=CARTESIAN_POINT('Ctrl Pts',(-0.163909452640218,0.17216396820272,
-1.28881982984788));
#78366=CARTESIAN_POINT('Ctrl Pts',(-0.14640858397937,0.186715653042787,
-1.29047664895832));
#78367=CARTESIAN_POINT('Ctrl Pts',(-0.140995762192899,0.190836094953807,
-1.29096859992884));
#78368=CARTESIAN_POINT('Ctrl Pts',(-0.133225045603013,0.196240083922836,
-1.29164029682386));
#78369=CARTESIAN_POINT('Ctrl Pts',(-0.131011441475805,0.197724775372766,
-1.2918279293152));
#78370=CARTESIAN_POINT('Ctrl Pts',(-0.127086746646118,0.200262259059966,
-1.29215355699167));
#78371=CARTESIAN_POINT('Ctrl Pts',(-0.12538645638855,0.2013311967805,-1.29229237270104));
#78372=CARTESIAN_POINT('Ctrl Pts',(-0.122805952756376,0.20290813302879,
-1.29249944676409));
#78373=CARTESIAN_POINT('Ctrl Pts',(-0.121935766244549,0.203432252820918,
-1.29256866778261));
#78374=CARTESIAN_POINT('Ctrl Pts',(-0.120348565082024,0.20437439237667,
-1.29269378803014));
#78375=CARTESIAN_POINT('Ctrl Pts',(-0.119632704711833,0.20479425135185,
-1.29274980005055));
#78376=CARTESIAN_POINT('Ctrl Pts',(-0.118002674916204,0.205738815585851,
-1.2928763991299));
#78377=CARTESIAN_POINT('Ctrl Pts',(-0.117087197006904,0.206261193462472,
-1.29294683925375));
#78378=CARTESIAN_POINT('Ctrl Pts',(-0.114246584818606,0.20785705854695,
-1.29316346424137));
#78379=CARTESIAN_POINT('Ctrl Pts',(-0.112309883359026,0.208909860661662,
-1.2933084205414));
#78380=CARTESIAN_POINT('Ctrl Pts',(-0.0974643434743828,0.216713848486018,
-1.29440108104783));
#78381=CARTESIAN_POINT('Ctrl Pts',(-0.0839711009534717,0.222290708842954,
-1.29529015439558));
#78382=CARTESIAN_POINT('Ctrl Pts',(-0.060820204530989,0.229447618452871,
-1.29677615038389));
#78383=CARTESIAN_POINT('Ctrl Pts',(-0.0514312966570702,0.231732338867738,
-1.29736850194418));
#78384=CARTESIAN_POINT('Ctrl Pts',(-0.0419357855265143,0.233438151374779,
-1.29797390460371));
#78385=CARTESIAN_POINT('Ctrl Pts',(-0.0419358330286197,0.233438142841301,
-1.31793598285019));
#78386=CARTESIAN_POINT('Ctrl Pts',(-0.0450441429985747,0.232879752655727,
-1.31773957474262));
#78387=CARTESIAN_POINT('Ctrl Pts',(-0.04814179629025,0.232259191105194,
-1.31754205121923));
#78388=CARTESIAN_POINT('Ctrl Pts',(-0.0577876136853906,0.230125446609451,
-1.31691982461284));
#78389=CARTESIAN_POINT('Ctrl Pts',(-0.0642831373476861,0.228396136166716,
-1.3164903219229));
#78390=CARTESIAN_POINT('Ctrl Pts',(-0.0728828678656407,0.225710692145085,
-1.31590261812276));
#78391=CARTESIAN_POINT('Ctrl Pts',(-0.0750595815023466,0.224996194635055,
-1.31575220065891));
#78392=CARTESIAN_POINT('Ctrl Pts',(-0.0786887843991768,0.223746398463105,
-1.31549844435571));
#78393=CARTESIAN_POINT('Ctrl Pts',(-0.0801470286781594,0.223228199869836,
-1.31539567109858));
#78394=CARTESIAN_POINT('Ctrl Pts',(-0.0830175950225842,0.222176368475757,
-1.31519170064363));
#78395=CARTESIAN_POINT('Ctrl Pts',(-0.0844301008704209,0.221643447179722,
-1.31509053112946));
#78396=CARTESIAN_POINT('Ctrl Pts',(-0.0875440662685072,0.220434500101537,
-1.31486566957707));
#78397=CARTESIAN_POINT('Ctrl Pts',(-0.0892429653781162,0.219752190382436,
-1.31474177220115));
#78398=CARTESIAN_POINT('Ctrl Pts',(-0.095123864715261,0.217310868621154,
-1.31430853688414));
#78399=CARTESIAN_POINT('Ctrl Pts',(-0.099262935789353,0.215451683609025,
-1.31399587239903));
#78400=CARTESIAN_POINT('Ctrl Pts',(-0.107841142029432,0.211298867914212,
-1.3133310339242));
#78401=CARTESIAN_POINT('Ctrl Pts',(-0.112266229694683,0.208981366202108,
-1.31297821762308));
#78402=CARTESIAN_POINT('Ctrl Pts',(-0.135252818582009,0.196002023127546,
-1.31109382928894));
#78403=CARTESIAN_POINT('Ctrl Pts',(-0.152378581360006,0.183004848574158,
-1.30949568664175));
#78404=CARTESIAN_POINT('Ctrl Pts',(-0.169827168311404,0.165593669404444,
-1.30775593115861));
#78405=CARTESIAN_POINT('Ctrl Pts',(-0.17207912029863,0.163252287469712,
-1.30752913127844));
#78406=CARTESIAN_POINT('Ctrl Pts',(-0.175114118411427,0.159964151903194,
-1.30722117380077));
#78407=CARTESIAN_POINT('Ctrl Pts',(-0.175938864106136,0.159056595656399,
-1.30713724564809));
#78408=CARTESIAN_POINT('Ctrl Pts',(-0.177323949862539,0.15750848087697,
-1.30699594322574));
#78409=CARTESIAN_POINT('Ctrl Pts',(-0.17788794223114,0.156871236513331,
-1.3069383058608));
#78410=CARTESIAN_POINT('Ctrl Pts',(-0.179052322504935,0.155541269988359,
-1.30681912308066));
#78411=CARTESIAN_POINT('Ctrl Pts',(-0.179652140987566,0.154848084179086,
-1.30675761760112));
#78412=CARTESIAN_POINT('Ctrl Pts',(-0.181247697066692,0.152982414132579,
-1.30659365795654));
#78413=CARTESIAN_POINT('Ctrl Pts',(-0.182236092275154,0.151803668288471,
-1.30649171863803));
#78414=CARTESIAN_POINT('Ctrl Pts',(-0.186798973782789,0.146253243879088,
-1.3060189085307));
#78415=CARTESIAN_POINT('Ctrl Pts',(-0.190228361183153,0.141764063963232,
-1.30565708234828));
#78416=CARTESIAN_POINT('Ctrl Pts',(-0.201045234314995,0.126504068229178,
-1.30447768072002));
#78417=CARTESIAN_POINT('Ctrl Pts',(-0.207703892625618,0.115245828996515,
-1.30368602951979));
#78418=CARTESIAN_POINT('Ctrl Pts',(-0.218233931378992,0.0935335708904622,
-1.30220210262495));
#78419=CARTESIAN_POINT('Ctrl Pts',(-0.222361564696137,0.0832458788099616,
-1.30151496832772));
#78420=CARTESIAN_POINT('Ctrl Pts',(-0.22700510615083,0.0688279064878478,
-1.30054389320636));
#78421=CARTESIAN_POINT('Ctrl Pts',(-0.228154499275156,0.0649162554910571,
-1.30027975831467));
#78422=CARTESIAN_POINT('Ctrl Pts',(-0.2296928062652,0.0591340236838122,
-1.29988730638604));
#78423=CARTESIAN_POINT('Ctrl Pts',(-0.230160879397401,0.0572851398640504,
-1.29976152481689));
#78424=CARTESIAN_POINT('Ctrl Pts',(-0.230952948371306,0.053989929567063,
-1.29953672963019));
#78425=CARTESIAN_POINT('Ctrl Pts',(-0.231285783794987,0.0525458171528234,
-1.29943800472394));
#78426=CARTESIAN_POINT('Ctrl Pts',(-0.231960053659516,0.0494896868279002,
-1.29922858992634));
#78427=CARTESIAN_POINT('Ctrl Pts',(-0.232298264732778,0.0478770462857149,
-1.29911780297253));
#78428=CARTESIAN_POINT('Ctrl Pts',(-0.233159353221392,0.0435471379775066,
-1.29881951843526));
#78429=CARTESIAN_POINT('Ctrl Pts',(-0.233651512436548,0.0408240962170101,
-1.298631062065));
#78430=CARTESIAN_POINT('Ctrl Pts',(-0.236157087266594,0.0254264570466844,
-1.29756011921402));
#78431=CARTESIAN_POINT('Ctrl Pts',(-0.237186487745343,0.0126154199031188,
-1.29664718680896));
#78432=CARTESIAN_POINT('Ctrl Pts',(-0.237163727982746,-0.0125906655638286,
-1.29481955572637));
#78433=CARTESIAN_POINT('Ctrl Pts',(-0.236183822465995,-0.0249471197383958,
-1.29390906147413));
#78434=CARTESIAN_POINT('Ctrl Pts',(-0.233208241266744,-0.0436988271985021,
-1.29254025055463));
#78435=CARTESIAN_POINT('Ctrl Pts',(-0.231899765624004,-0.0501815388615261,
-1.2920697584571));
#78436=CARTESIAN_POINT('Ctrl Pts',(-0.229938258470567,-0.0581632503069999,
-1.2915002685275));
#78437=CARTESIAN_POINT('Ctrl Pts',(-0.22953861792341,-0.0597209312621274,
-1.29138960360416));
#78438=CARTESIAN_POINT('Ctrl Pts',(-0.228882403554558,-0.062174708199118,
-1.29121615496909));
#78439=CARTESIAN_POINT('Ctrl Pts',(-0.228636346429202,-0.0630735298139263,
-1.29115280794653));
#78440=CARTESIAN_POINT('Ctrl Pts',(-0.22815722786432,-0.0647840496747016,
-1.29103264254622));
#78441=CARTESIAN_POINT('Ctrl Pts',(-0.227925122152485,-0.0655959787771291,
-1.2909757751496));
#78442=CARTESIAN_POINT('Ctrl Pts',(-0.227355984668928,-0.0675473817708406,
-1.29083948101293));
#78443=CARTESIAN_POINT('Ctrl Pts',(-0.227014711547396,-0.0686856130343581,
-1.29076029479745));
#78444=CARTESIAN_POINT('Ctrl Pts',(-0.225784335532602,-0.0726798554655385,
-1.29048336104323));
#78445=CARTESIAN_POINT('Ctrl Pts',(-0.224849733719117,-0.0755216976234497,
-1.29028803050334));
#78446=CARTESIAN_POINT('Ctrl Pts',(-0.22235377324437,-0.0826535862708674,
-1.28980035416054));
#78447=CARTESIAN_POINT('Ctrl Pts',(-0.220721824881644,-0.0869177590281617,
-1.28951110732223));
#78448=CARTESIAN_POINT('Ctrl Pts',(-0.211216182583872,-0.109757369678011,
-1.28796124740441));
#78449=CARTESIAN_POINT('Ctrl Pts',(-0.201120220918594,-0.127317224426492,
-1.28676008226972));
#78450=CARTESIAN_POINT('Ctrl Pts',(-0.185304495136652,-0.148155487006802,
-1.28510636895507));
#78451=CARTESIAN_POINT('Ctrl Pts',(-0.181507086894655,-0.152784071292551,
-1.28472277003582));
#78452=CARTESIAN_POINT('Ctrl Pts',(-0.176036867941301,-0.158959533811389,
-1.28418443151328));
#78453=CARTESIAN_POINT('Ctrl Pts',(-0.174510632909879,-0.160633591392015,
-1.28403565717631));
#78454=CARTESIAN_POINT('Ctrl Pts',(-0.172010745431868,-0.163297922573376,
-1.28379407810843));
#78455=CARTESIAN_POINT('Ctrl Pts',(-0.171051941766071,-0.164301981546365,
-1.28370190632642));
#78456=CARTESIAN_POINT('Ctrl Pts',(-0.169033394393446,-0.166378983989582,
-1.28350881842571));
#78457=CARTESIAN_POINT('Ctrl Pts',(-0.167972124823112,-0.167450350358176,
-1.2834078382839));
#78458=CARTESIAN_POINT('Ctrl Pts',(-0.165421373517851,-0.169976719491634,
-1.28316635265509));
#78459=CARTESIAN_POINT('Ctrl Pts',(-0.163922827664636,-0.171422349989504,
-1.28302544829807));
#78460=CARTESIAN_POINT('Ctrl Pts',(-0.15865988695442,-0.176367332347506,
-1.28253375689749));
#78461=CARTESIAN_POINT('Ctrl Pts',(-0.154801157888161,-0.179763706378,-1.28217871379119));
#78462=CARTESIAN_POINT('Ctrl Pts',(-0.144893338313225,-0.187928678431054,
-1.28127979746314));
#78463=CARTESIAN_POINT('Ctrl Pts',(-0.138716863633347,-0.192532802977061,
-1.28073039985551));
#78464=CARTESIAN_POINT('Ctrl Pts',(-0.124935431366625,-0.201798088856931,
-1.27953084557776));
#78465=CARTESIAN_POINT('Ctrl Pts',(-0.117269002870168,-0.206347526527299,
-1.27887925605728));
#78466=CARTESIAN_POINT('Ctrl Pts',(-0.0993585797783119,-0.215654877290188,
-1.27740724124203));
#78467=CARTESIAN_POINT('Ctrl Pts',(-0.0889926650755201,-0.220135221091236,
-1.27658961037133));
#78468=CARTESIAN_POINT('Ctrl Pts',(-0.0767226060801704,-0.22442945758325,
-1.27568711172987));
#78469=CARTESIAN_POINT('Ctrl Pts',(-0.0750927753327918,-0.224980032971189,
-1.27556853213438));
#78470=CARTESIAN_POINT('Ctrl Pts',(-0.0725383412970844,-0.225812097165995,
-1.27538485780239));
#78471=CARTESIAN_POINT('Ctrl Pts',(-0.0716178012997184,-0.226105738106755,
-1.27531910508714));
#78472=CARTESIAN_POINT('Ctrl Pts',(-0.0699784652905857,-0.226617649908129,
-1.27520281843302));
#78473=CARTESIAN_POINT('Ctrl Pts',(-0.0692604158059864,-0.226838135417788,
-1.27515216073012));
#78474=CARTESIAN_POINT('Ctrl Pts',(-0.0675160309834869,-0.227364713949789,
-1.27502975417674));
#78475=CARTESIAN_POINT('Ctrl Pts',(-0.0664886535288321,-0.227667271805715,
-1.2749582086996));
#78476=CARTESIAN_POINT('Ctrl Pts',(-0.0632527759030804,-0.228596449806423,
-1.27473447949377));
#78477=CARTESIAN_POINT('Ctrl Pts',(-0.0610371317592492,-0.229197993064283,
-1.27458364336766));
#78478=CARTESIAN_POINT('Ctrl Pts',(-0.0490308158085041,-0.232271221989006,
-1.27377719053391));
#78479=CARTESIAN_POINT('Ctrl Pts',(-0.039097545118008,-0.234148178577223,
-1.27314869165308));
#78480=CARTESIAN_POINT('Ctrl Pts',(-0.0105130346913182,-0.237678810716966,
-1.27137432567611));
#78481=CARTESIAN_POINT('Ctrl Pts',(0.00825210940212877,-0.237767937218976,
-1.27024491584511));
#78482=CARTESIAN_POINT('Ctrl Pts',(0.0307053456039303,-0.235211299498663,
-1.26879406032633));
#78483=CARTESIAN_POINT('Ctrl Pts',(0.0345664947360843,-0.234674941819115,
-1.26854123294892));
#78484=CARTESIAN_POINT('Ctrl Pts',(0.0402623746793533,-0.233740103541622,
-1.26816243328623));
#78485=CARTESIAN_POINT('Ctrl Pts',(0.0421085330731738,-0.233414579504707,
-1.26803874372369));
#78486=CARTESIAN_POINT('Ctrl Pts',(0.0454034487304112,-0.23279324154899,
-1.26781626218158));
#78487=CARTESIAN_POINT('Ctrl Pts',(0.0468536794602432,-0.232505696746309,
-1.26771773674122));
#78488=CARTESIAN_POINT('Ctrl Pts',(0.0499327580407142,-0.231865214733297,
-1.26750722331897));
#78489=CARTESIAN_POINT('Ctrl Pts',(0.0515607567142857,-0.231508631049575,
-1.26739512395608));
#78490=CARTESIAN_POINT('Ctrl Pts',(0.0559679587577904,-0.230494520891279,
-1.26708942877798));
#78491=CARTESIAN_POINT('Ctrl Pts',(0.0587391857584915,-0.229803923789111,
-1.26689478953184));
#78492=CARTESIAN_POINT('Ctrl Pts',(0.0648664927568811,-0.22815891249998,
-1.26645885599361));
#78493=CARTESIAN_POINT('Ctrl Pts',(0.0682152918508011,-0.227180155430401,
-1.26621683415158));
#78494=CARTESIAN_POINT('Ctrl Pts',(0.0788243320530306,-0.223823724309985,
-1.26543789013055));
#78495=CARTESIAN_POINT('Ctrl Pts',(0.0859913049501179,-0.221169192154312,
-1.26489300246711));
#78496=CARTESIAN_POINT('Ctrl Pts',(0.10074000545528,-0.214881165343914,
-1.26373518793276));
#78497=CARTESIAN_POINT('Ctrl Pts',(0.10828233387994,-0.211180943681267,
-1.26312162378104));
#78498=CARTESIAN_POINT('Ctrl Pts',(0.125204840653095,-0.201733546780958,
-1.26170747701845));
#78499=CARTESIAN_POINT('Ctrl Pts',(0.134414642907821,-0.195717720522456,
-1.26090902967387));
#78500=CARTESIAN_POINT('Ctrl Pts',(0.144830034500502,-0.187831179552273,
-1.25999558077016));
#78501=CARTESIAN_POINT('Ctrl Pts',(0.146468735455883,-0.186556160851772,
-1.25985155522803));
#78502=CARTESIAN_POINT('Ctrl Pts',(0.148905496880018,-0.184608293808231,
-1.25963717685695));
#78503=CARTESIAN_POINT('Ctrl Pts',(0.149716156998933,-0.183951465279907,
-1.25956582184369));
#78504=CARTESIAN_POINT('Ctrl Pts',(0.151175701040167,-0.182752845452011,
-1.25943732671426));
#78505=CARTESIAN_POINT('Ctrl Pts',(0.151826072585513,-0.182212894378135,
-1.25938006077436));
#78506=CARTESIAN_POINT('Ctrl Pts',(0.153169550020457,-0.181085325682063,
-1.25926177034901));
#78507=CARTESIAN_POINT('Ctrl Pts',(0.153862186401006,-0.180497185286605,
-1.25920078435919));
#78508=CARTESIAN_POINT('Ctrl Pts',(0.155690424684337,-0.17892659661308,
-1.25903975424156));
#78509=CARTESIAN_POINT('Ctrl Pts',(0.15682012772571,-0.177937301152442,
-1.25894019332116));
#78510=CARTESIAN_POINT('Ctrl Pts',(0.162315523802163,-0.173031919605993,
-1.25845515414894));
#78511=CARTESIAN_POINT('Ctrl Pts',(0.166544705055028,-0.168965228024774,
-1.25807957309652));
#78512=CARTESIAN_POINT('Ctrl Pts',(0.180245619459974,-0.154775844527607,
-1.25683694899645));
#78513=CARTESIAN_POINT('Ctrl Pts',(0.18898030055248,-0.143981032986993,
-1.25599881848316));
#78514=CARTESIAN_POINT('Ctrl Pts',(0.203600700860742,-0.1222716175674,-1.25438640198874));
#78515=CARTESIAN_POINT('Ctrl Pts',(0.20967216701723,-0.11153976975976,-1.25361792586346));
#78516=CARTESIAN_POINT('Ctrl Pts',(0.216050106899534,-0.0978873724638894,
-1.25264022120727));
#78517=CARTESIAN_POINT('Ctrl Pts',(0.217173676647155,-0.0953686506188229,
-1.25245990714688));
#78518=CARTESIAN_POINT('Ctrl Pts',(0.218897190885251,-0.0913165317726143,
-1.25216961265539));
#78519=CARTESIAN_POINT('Ctrl Pts',(0.219525551547244,-0.0897954405329999,
-1.252060596824));
#78520=CARTESIAN_POINT('Ctrl Pts',(0.220689712085365,-0.0868920542996715,
-1.25185236603007));
#78521=CARTESIAN_POINT('Ctrl Pts',(0.221228483257865,-0.0855110293747747,
-1.25175325671305));
#78522=CARTESIAN_POINT('Ctrl Pts',(0.222432020934401,-0.08233849582987,
-1.25152539224879));
#78523=CARTESIAN_POINT('Ctrl Pts',(0.223088146145137,-0.080543842167447,
-1.2513963568648));
#78524=CARTESIAN_POINT('Ctrl Pts',(0.225082609794726,-0.0748771176937524,
-1.25098839037956));
#78525=CARTESIAN_POINT('Ctrl Pts',(0.226342289373083,-0.0709783658551482,
-1.25070692020863));
#78526=CARTESIAN_POINT('Ctrl Pts',(0.230791318739979,-0.0558826402858122,
-1.2496134749995));
#78527=CARTESIAN_POINT('Ctrl Pts',(0.233255297860058,-0.0444904764475818,
-1.24877970102691));
#78528=CARTESIAN_POINT('Ctrl Pts',(0.236820128736334,-0.0190912640524416,
-1.24691593649711));
#78529=CARTESIAN_POINT('Ctrl Pts',(0.237534297317153,-0.00507220455330229,
-1.24588367890338));
#78530=CARTESIAN_POINT('Ctrl Pts',(0.236843006920982,0.0132787376186449,
-1.24457583536122));
#78531=CARTESIAN_POINT('Ctrl Pts',(0.236559347471268,0.0176242897715005,
-1.24426951620173));
#78532=CARTESIAN_POINT('Ctrl Pts',(0.236025883066952,0.0233611583744994,
-1.24387162037408));
#78533=CARTESIAN_POINT('Ctrl Pts',(0.235883105807222,0.0247612971223859,
-1.24377502529658));
#78534=CARTESIAN_POINT('Ctrl Pts',(0.235629920835171,0.0270427371355732,
-1.24361855944217));
#78535=CARTESIAN_POINT('Ctrl Pts',(0.235527013724967,0.027924811477552,
-1.24355829219037));
#78536=CARTESIAN_POINT('Ctrl Pts',(0.235313569349336,0.0296691828447669,
-1.24343958639284));
#78537=CARTESIAN_POINT('Ctrl Pts',(0.235203241316504,0.0305314862230657,
-1.24338113855616));
#78538=CARTESIAN_POINT('Ctrl Pts',(0.234913447447265,0.0327016109983514,
-1.2432345874128));
#78539=CARTESIAN_POINT('Ctrl Pts',(0.234727796429805,0.0340086009129097,
-1.24314682143507));
#78540=CARTESIAN_POINT('Ctrl Pts',(0.233940673480156,0.0392361273351585,
-1.24279753089698));
#78541=CARTESIAN_POINT('Ctrl Pts',(0.233251775092791,0.0431430896531191,
-1.24254041167414));
#78542=CARTESIAN_POINT('Ctrl Pts',(0.231095065483561,0.0538032444869224,
-1.24184514534651));
#78543=CARTESIAN_POINT('Ctrl Pts',(0.229429613166123,0.0605126784784325,
-1.24141448516452));
#78544=CARTESIAN_POINT('Ctrl Pts',(0.22284436955349,0.0828237140128339,
-1.23997794857061));
#78545=CARTESIAN_POINT('Ctrl Pts',(0.216606019691338,0.0979857082961548,
-1.23899106481429));
#78546=CARTESIAN_POINT('Ctrl Pts',(0.205951842108191,0.117785504292723,
-1.23757102034217));
#78547=CARTESIAN_POINT('Ctrl Pts',(0.202837902719818,0.123070555631066,
-1.23717827743808));
#78548=CARTESIAN_POINT('Ctrl Pts',(0.198286980784147,0.130151755539494,
-1.23662914227295));
#78549=CARTESIAN_POINT('Ctrl Pts',(0.197023377613028,0.132056784357728,
-1.23647904374724));
#78550=CARTESIAN_POINT('Ctrl Pts',(0.194946324922046,0.135092001240454,
-1.23623589007464));
#78551=CARTESIAN_POINT('Ctrl Pts',(0.194150094447349,0.136233839724119,
-1.23614348420485));
#78552=CARTESIAN_POINT('Ctrl Pts',(0.1924720882906,0.138595603983667,-1.23595036146244));
#78553=CARTESIAN_POINT('Ctrl Pts',(0.19158866078083,0.139814273573524,-1.23584958428538));
#78554=CARTESIAN_POINT('Ctrl Pts',(0.189465453198506,0.142685282077827,
-1.23560943094656));
#78555=CARTESIAN_POINT('Ctrl Pts',(0.18821558527278,0.144329971485164,-1.23546966757829));
#78556=CARTESIAN_POINT('Ctrl Pts',(0.183848325930768,0.149923596657927,
-1.23498660062116));
#78557=CARTESIAN_POINT('Ctrl Pts',(0.180627052215816,0.153789314269525,
-1.23463923941294));
#78558=CARTESIAN_POINT('Ctrl Pts',(0.172326718473209,0.163129422210018,
-1.23376502065946));
#78559=CARTESIAN_POINT('Ctrl Pts',(0.167107689350186,0.168471685231689,
-1.23323303037805));
#78560=CARTESIAN_POINT('Ctrl Pts',(0.155082334784136,0.179671643960712,
-1.23204733898518));
#78561=CARTESIAN_POINT('Ctrl Pts',(0.148177503900019,0.185407244343262,
-1.23139154838752));
#78562=CARTESIAN_POINT('Ctrl Pts',(0.13164387099311,0.197626426020707,-1.22989178108285));
#78563=CARTESIAN_POINT('Ctrl Pts',(0.1218294744188,0.203823334251217,-1.22905050540981));
#78564=CARTESIAN_POINT('Ctrl Pts',(0.110077478450933,0.210090237085562,
-1.22812580363861));
#78565=CARTESIAN_POINT('Ctrl Pts',(0.108545802984555,0.210885675348611,
-1.2280068309674));
#78566=CARTESIAN_POINT('Ctrl Pts',(0.106142131123382,0.212100835915446,
-1.22782268155167));
#78567=CARTESIAN_POINT('Ctrl Pts',(0.105276053468683,0.212532042866423,
-1.22775684157335));
#78568=CARTESIAN_POINT('Ctrl Pts',(0.103733073253316,0.213288523032304,
-1.2276404808205));
#78569=CARTESIAN_POINT('Ctrl Pts',(0.103057253835324,0.213615886579926,
-1.22758983533707));
#78570=CARTESIAN_POINT('Ctrl Pts',(0.101415461003773,0.214401557718059,
-1.22746756117304));
#78571=CARTESIAN_POINT('Ctrl Pts',(0.10044792823023,0.214856550997556,-1.22739613463144));
#78572=CARTESIAN_POINT('Ctrl Pts',(0.0974023185357063,0.216263713491801,
-1.22717316978657));
#78573=CARTESIAN_POINT('Ctrl Pts',(0.0953134632994689,0.217192426401864,
-1.22702296604742));
#78574=CARTESIAN_POINT('Ctrl Pts',(0.0840155051846943,0.222021142179964,
-1.22622336193045));
#78575=CARTESIAN_POINT('Ctrl Pts',(0.0745791271001816,0.225366349657924,
-1.22560057551634));
#78576=CARTESIAN_POINT('Ctrl Pts',(0.0472643139616395,0.233144910556682,
-1.22385045008607));
#78577=CARTESIAN_POINT('Ctrl Pts',(0.0290451990073976,0.236107592732624,
-1.22273960580836));
#78578=CARTESIAN_POINT('Ctrl Pts',(0.00649936194552893,0.237122635682033,
-1.22129384957588));
#78579=CARTESIAN_POINT('Ctrl Pts',(0.00232759538006935,0.23720026344767,
-1.22102368410162));
#78580=CARTESIAN_POINT('Ctrl Pts',(-0.003747372722769,0.237153033754965,
-1.22062532152382));
#78581=CARTESIAN_POINT('Ctrl Pts',(-0.00565059503424683,0.237115319300166,
-1.2204998148991));
#78582=CARTESIAN_POINT('Ctrl Pts',(-0.00903786662288286,0.237007392976922,
-1.22027509270159));
#78583=CARTESIAN_POINT('Ctrl Pts',(-0.0105221142464977,0.236946137970936,
-1.22017616094276));
#78584=CARTESIAN_POINT('Ctrl Pts',(-0.0136363831216303,0.236788293141701,
-1.21996756505058));
#78585=CARTESIAN_POINT('Ctrl Pts',(-0.0152661726847158,0.23668880508901,
-1.21985781552019));
#78586=CARTESIAN_POINT('Ctrl Pts',(-0.0195850273237711,0.236380375080471,
-1.21956537070213));
#78587=CARTESIAN_POINT('Ctrl Pts',(-0.0222717101378768,0.236142382693003,
-1.2193817812597));
#78588=CARTESIAN_POINT('Ctrl Pts',(-0.0306441885390416,0.235256581103655,
-1.21880423717975));
#78589=CARTESIAN_POINT('Ctrl Pts',(-0.0363085877279333,0.234449045685933,
-1.21840560443526));
#78590=CARTESIAN_POINT('Ctrl Pts',(-0.0419358439263085,0.233438140883593,
-1.21800162451869));
#78591=CARTESIAN_POINT('Origin',(0.,0.,-1.7456589891905));
#78592=CARTESIAN_POINT('',(-0.0419358102824307,0.233438146927523,-1.09805944304797));
#78593=CARTESIAN_POINT('',(-0.0419358257386354,0.233438144150905,-1.11763442355469));
#78594=CARTESIAN_POINT('',(-0.0419358257166344,0.233438144154858,-1.7456589891905));
#78595=CARTESIAN_POINT('Ctrl Pts',(-0.0419358102824291,0.233438146927524,
-1.09805944304797));
#78596=CARTESIAN_POINT('Ctrl Pts',(-0.0379568861939225,0.234152937581493,
-1.09835331162497));
#78597=CARTESIAN_POINT('Ctrl Pts',(-0.0339584290944791,0.23476622439805,
-1.09864841709242));
#78598=CARTESIAN_POINT('Ctrl Pts',(-0.0166710106798612,0.236966435425049,
-1.09992053886217));
#78599=CARTESIAN_POINT('Ctrl Pts',(-0.00327721598154022,0.237529675797298,
-1.10089800105867));
#78600=CARTESIAN_POINT('Ctrl Pts',(0.0119081045847333,0.236882831003429,
-1.10195430417511));
#78601=CARTESIAN_POINT('Ctrl Pts',(0.013721608450018,0.236784705040578,
-1.1020795840633));
#78602=CARTESIAN_POINT('Ctrl Pts',(0.0165082372712046,0.236601800926374,
-1.1022705740362));
#78603=CARTESIAN_POINT('Ctrl Pts',(0.0174822186028563,0.236531829185448,
-1.10233704370119));
#78604=CARTESIAN_POINT('Ctrl Pts',(0.0192867741586138,0.236390980700097,
-1.10245963342723));
#78605=CARTESIAN_POINT('Ctrl Pts',(0.0201174167927684,0.236321740400687,
-1.1025158365596));
#78606=CARTESIAN_POINT('Ctrl Pts',(0.0220304384324753,0.236152116036669,
-1.10264477469416));
#78607=CARTESIAN_POINT('Ctrl Pts',(0.0231125128605143,0.236048668689644,
-1.10271734038701));
#78608=CARTESIAN_POINT('Ctrl Pts',(0.026628246868269,0.235688153348297,
-1.10295203116607));
#78609=CARTESIAN_POINT('Ctrl Pts',(0.0290587371354134,0.235400849825394,
-1.10311259246941));
#78610=CARTESIAN_POINT('Ctrl Pts',(0.0494228640885475,0.232673418617775,
-1.10444699357168));
#78611=CARTESIAN_POINT('Ctrl Pts',(0.0670297559238366,0.228225179715533,
-1.10553318500805));
#78612=CARTESIAN_POINT('Ctrl Pts',(0.0917299520849377,0.218875764162056,
-1.10715993523477));
#78613=CARTESIAN_POINT('Ctrl Pts',(0.0993385556377833,0.215529163551474,
-1.1076758790892));
#78614=CARTESIAN_POINT('Ctrl Pts',(0.110040452574452,0.210134747229016,
-1.10843678363915));
#78615=CARTESIAN_POINT('Ctrl Pts',(0.113286288201231,0.208402802183751,
-1.10867242878256));
#78616=CARTESIAN_POINT('Ctrl Pts',(0.119082883116074,0.2051343591205,-1.10910322992232));
#78617=CARTESIAN_POINT('Ctrl Pts',(0.121647512319049,0.203623966678832,
-1.10929748570112));
#78618=CARTESIAN_POINT('Ctrl Pts',(0.125624725325469,0.201179702841588,
-1.10960491230329));
#78619=CARTESIAN_POINT('Ctrl Pts',(0.127056941588665,0.200278250924797,
-1.10971690494336));
#78620=CARTESIAN_POINT('Ctrl Pts',(0.129719692893389,0.198562230229268,
-1.10992761174361));
#78621=CARTESIAN_POINT('Ctrl Pts',(0.130952516365157,0.197751349645869,
-1.1100261856922));
#78622=CARTESIAN_POINT('Ctrl Pts',(0.133703042986597,0.195905211509962,
-1.11024845839622));
#78623=CARTESIAN_POINT('Ctrl Pts',(0.135216430907903,0.194863726957308,
-1.11037238729124));
#78624=CARTESIAN_POINT('Ctrl Pts',(0.13973810751901,0.19167395823162,-1.11074770132054));
#78625=CARTESIAN_POINT('Ctrl Pts',(0.142708298660339,0.189472910435648,
-1.11100107836532));
#78626=CARTESIAN_POINT('Ctrl Pts',(0.160571045103683,0.17557746715302,-1.11256830325633));
#78627=CARTESIAN_POINT('Ctrl Pts',(0.174068028101914,0.162205353187178,
-1.1139499374506));
#78628=CARTESIAN_POINT('Ctrl Pts',(0.192148652817416,0.13940694373149,-1.11607154335916));
#78629=CARTESIAN_POINT('Ctrl Pts',(0.197949400544702,0.131039976854892,
-1.11680872452397));
#78630=CARTESIAN_POINT('Ctrl Pts',(0.204383349933768,0.120352529290333,
-1.11768097305564));
#78631=CARTESIAN_POINT('Ctrl Pts',(0.205542467371631,0.118362072151934,
-1.11784061497889));
#78632=CARTESIAN_POINT('Ctrl Pts',(0.207198630536244,0.1154203555069,-1.11807212780044));
#78633=CARTESIAN_POINT('Ctrl Pts',(0.207718470588126,0.114482173501986,
-1.11814531351209));
#78634=CARTESIAN_POINT('Ctrl Pts',(0.208591700254312,0.112880680214559,
-1.11826910167038));
#78635=CARTESIAN_POINT('Ctrl Pts',(0.208948324474874,0.112219174556597,
-1.11831990327893));
#78636=CARTESIAN_POINT('Ctrl Pts',(0.209756020322366,0.110703771771564,
-1.11843552361632));
#78637=CARTESIAN_POINT('Ctrl Pts',(0.21020502784578,0.109848802891782,-1.11850021353258));
#78638=CARTESIAN_POINT('Ctrl Pts',(0.21143786020895,0.107466088345999,-1.11867906563629));
#78639=CARTESIAN_POINT('Ctrl Pts',(0.212210353842035,0.105932502167883,
-1.11879255542525));
#78640=CARTESIAN_POINT('Ctrl Pts',(0.217691925524666,0.0947496069830524,
-1.11960938515718));
#78641=CARTESIAN_POINT('Ctrl Pts',(0.221758207810503,0.0847975186055965,
-1.12027903004796));
#78642=CARTESIAN_POINT('Ctrl Pts',(0.225699193913305,0.0729044320733339,
-1.12105138176533));
#78643=CARTESIAN_POINT('Ctrl Pts',(0.226242790643945,0.071199593504161,
-1.1211614387327));
#78644=CARTESIAN_POINT('Ctrl Pts',(0.229057632932387,0.0620137408996998,
-1.12175163552292));
#78645=CARTESIAN_POINT('Ctrl Pts',(0.230977205426684,0.0544300674448357,
-1.12222913516895));
#78646=CARTESIAN_POINT('Ctrl Pts',(0.234018036185483,0.0393110316288712,
-1.12318153568289));
#78647=CARTESIAN_POINT('Ctrl Pts',(0.235157886907406,0.0317892094317245,
-1.12365559003462));
#78648=CARTESIAN_POINT('Ctrl Pts',(0.236289806934538,0.0207655661354777,
-1.12436066678052));
#78649=CARTESIAN_POINT('Ctrl Pts',(0.236568941063478,0.0172978577153588,
-1.12458390541195));
#78650=CARTESIAN_POINT('Ctrl Pts',(0.236937814318573,0.0109805865294207,
-1.12499409383492));
#78651=CARTESIAN_POINT('Ctrl Pts',(0.237052636155568,0.00813312326850457,
-1.12518027265812));
#78652=CARTESIAN_POINT('Ctrl Pts',(0.237153233259539,0.00361921584620531,
-1.12547778705443));
#78653=CARTESIAN_POINT('Ctrl Pts',(0.237172800738508,0.00195374530733741,
-1.12558807051801));
#78654=CARTESIAN_POINT('Ctrl Pts',(0.237176622468758,-0.00119089941568732,
-1.12579733092218));
#78655=CARTESIAN_POINT('Ctrl Pts',(0.2371645830232,-0.00266999556853016,
-1.12589618738561));
#78656=CARTESIAN_POINT('Ctrl Pts',(0.237105864454018,-0.0060262104382984,
-1.1261215234105));
#78657=CARTESIAN_POINT('Ctrl Pts',(0.237050727542241,-0.00790306210016809,
-1.12624826051714));
#78658=CARTESIAN_POINT('Ctrl Pts',(0.236848789925979,-0.0127965839830782,
-1.12658067828505));
#78659=CARTESIAN_POINT('Ctrl Pts',(0.236666645128691,-0.0158113718454506,
-1.12678743737864));
#78660=CARTESIAN_POINT('Ctrl Pts',(0.235030222425289,-0.0363670922790522,
-1.12821113877261));
#78661=CARTESIAN_POINT('Ctrl Pts',(0.231684966740276,-0.0536994512001545,
-1.12948720458719));
#78662=CARTESIAN_POINT('Ctrl Pts',(0.222744317114931,-0.0824184046399465,
-1.1316828527758));
#78663=CARTESIAN_POINT('Ctrl Pts',(0.218097936040237,-0.0940275297809924,
-1.13259319541156));
#78664=CARTESIAN_POINT('Ctrl Pts',(0.211658486553904,-0.107036364051021,
-1.13360481667437));
#78665=CARTESIAN_POINT('Ctrl Pts',(0.210734947422177,-0.108843377291534,
-1.13374510960598));
#78666=CARTESIAN_POINT('Ctrl Pts',(0.209312487455712,-0.111540591630558,
-1.13395392951042));
#78667=CARTESIAN_POINT('Ctrl Pts',(0.208830856307402,-0.112439737357566,
-1.13402344254483));
#78668=CARTESIAN_POINT('Ctrl Pts',(0.207946918314087,-0.114064667193416,
-1.13414884728472));
#78669=CARTESIAN_POINT('Ctrl Pts',(0.207546592278577,-0.114791468412994,
-1.13420485487078));
#78670=CARTESIAN_POINT('Ctrl Pts',(0.206631364403101,-0.116432645581979,
-1.13433114221386));
#78671=CARTESIAN_POINT('Ctrl Pts',(0.206114200753142,-0.117345720264258,
-1.13440127837755));
#78672=CARTESIAN_POINT('Ctrl Pts',(0.204504203039306,-0.120144756415573,
-1.134615992799));
#78673=CARTESIAN_POINT('Ctrl Pts',(0.203391382666009,-0.122019169957057,
-1.13475937347675));
#78674=CARTESIAN_POINT('Ctrl Pts',(0.194500326445898,-0.136535391462297,
-1.13586874097261));
#78675=CARTESIAN_POINT('Ctrl Pts',(0.185575657542781,-0.148438828680248,
-1.13677362065547));
#78676=CARTESIAN_POINT('Ctrl Pts',(0.16497822847736,-0.171124613563893,
-1.13865276890389));
#78677=CARTESIAN_POINT('Ctrl Pts',(0.153220901253196,-0.181727050625171,
-1.13962444560233));
#78678=CARTESIAN_POINT('Ctrl Pts',(0.138165686929101,-0.192796795172578,
-1.1408351812615));
#78679=CARTESIAN_POINT('Ctrl Pts',(0.135802244660728,-0.194468790384343,
-1.14102425148977));
#78680=CARTESIAN_POINT('Ctrl Pts',(0.13202384234333,-0.197039315489351,
-1.14132531500762));
#78681=CARTESIAN_POINT('Ctrl Pts',(0.130628899190503,-0.197966858968787,
-1.14143621176386));
#78682=CARTESIAN_POINT('Ctrl Pts',(0.127985191374101,-0.199684638743322,
-1.14164597813001));
#78683=CARTESIAN_POINT('Ctrl Pts',(0.12673863326206,-0.200478135541841,
-1.14174472010043));
#78684=CARTESIAN_POINT('Ctrl Pts',(0.123904425166016,-0.202245253126783,
-1.14196889275028));
#78685=CARTESIAN_POINT('Ctrl Pts',(0.122312574370884,-0.203211915978114,
-1.14209457063592));
#78686=CARTESIAN_POINT('Ctrl Pts',(0.118155070821138,-0.205670042304123,
-1.14242229765477));
#78687=CARTESIAN_POINT('Ctrl Pts',(0.115572582593216,-0.207132237553247,
-1.14262537576459));
#78688=CARTESIAN_POINT('Ctrl Pts',(0.0969645123772812,-0.217211722339492,
-1.14408571004271));
#78689=CARTESIAN_POINT('Ctrl Pts',(0.0800242044932442,-0.224006558375495,
-1.14540677223974));
#78690=CARTESIAN_POINT('Ctrl Pts',(0.0506573710478196,-0.232025762864838,
-1.14762867352109));
#78691=CARTESIAN_POINT('Ctrl Pts',(0.0386032106173287,-0.234333051683242,
-1.14852075039402));
#78692=CARTESIAN_POINT('Ctrl Pts',(0.0245681651621397,-0.235906489815959,
-1.14950294916515));
#78693=CARTESIAN_POINT('Ctrl Pts',(0.0227102269446111,-0.236092593722149,
-1.14963182293467));
#78694=CARTESIAN_POINT('Ctrl Pts',(0.0198669459657504,-0.236343519964401,
-1.14982709846271));
#78695=CARTESIAN_POINT('Ctrl Pts',(0.0188831233099919,-0.236424158481266,
-1.14989431173221));
#78696=CARTESIAN_POINT('Ctrl Pts',(0.0170690739544669,-0.236561450228668,
-1.15001755530464));
#78697=CARTESIAN_POINT('Ctrl Pts',(0.016239039773748,-0.236619877951739,
-1.15007367683561));
#78698=CARTESIAN_POINT('Ctrl Pts',(0.0143389670226909,-0.236743582327482,
-1.15020154602753));
#78699=CARTESIAN_POINT('Ctrl Pts',(0.0132687743564023,-0.236805974345982,
-1.15027313475458));
#78700=CARTESIAN_POINT('Ctrl Pts',(0.009838664754885,-0.2369826224232,-1.15050130823869));
#78701=CARTESIAN_POINT('Ctrl Pts',(0.00747736579035017,-0.23706887752416,
-1.15065644722717));
#78702=CARTESIAN_POINT('Ctrl Pts',(-0.0106753686953257,-0.237460461826431,
-1.15183693279482));
#78703=CARTESIAN_POINT('Ctrl Pts',(-0.0264625184678278,-0.236222996466737,
-1.1527947487485));
#78704=CARTESIAN_POINT('Ctrl Pts',(-0.0565479942935877,-0.230808302056091,
-1.15467080818325));
#78705=CARTESIAN_POINT('Ctrl Pts',(-0.0708068286774048,-0.226840169367799,
-1.15558399992836));
#78706=CARTESIAN_POINT('Ctrl Pts',(-0.087203329217904,-0.220579479207914,
-1.15672246529454));
#78707=CARTESIAN_POINT('Ctrl Pts',(-0.0897857384746955,-0.219540992489487,
-1.1569044043934));
#78708=CARTESIAN_POINT('Ctrl Pts',(-0.0938703353750423,-0.217814297385418,
-1.15719671405723));
#78709=CARTESIAN_POINT('Ctrl Pts',(-0.0953846900475314,-0.217155402146338,
-1.15730609623577));
#78710=CARTESIAN_POINT('Ctrl Pts',(-0.0982444529388262,-0.215875435413101,
-1.15751464320215));
#78711=CARTESIAN_POINT('Ctrl Pts',(-0.0995911679125088,-0.215257462706168,
-1.15761369823569));
#78712=CARTESIAN_POINT('Ctrl Pts',(-0.102653013448634,-0.213817577523939,
-1.15784089273573));
#78713=CARTESIAN_POINT('Ctrl Pts',(-0.104364206441023,-0.212987581038248,
-1.15796930613361));
#78714=CARTESIAN_POINT('Ctrl Pts',(-0.108841534430782,-0.210748988116981,
-1.15830919648846));
#78715=CARTESIAN_POINT('Ctrl Pts',(-0.111590240162673,-0.209306551096509,
-1.15852183289576));
#78716=CARTESIAN_POINT('Ctrl Pts',(-0.128245359726734,-0.200145122610809,
-1.15983532261843));
#78717=CARTESIAN_POINT('Ctrl Pts',(-0.141372263207861,-0.191098567686547,
-1.16098325038798));
#78718=CARTESIAN_POINT('Ctrl Pts',(-0.16416545409768,-0.171748834749719,
-1.16316502698073));
#78719=CARTESIAN_POINT('Ctrl Pts',(-0.174015518247122,-0.161761023090044,
-1.16419080476079));
#78720=CARTESIAN_POINT('Ctrl Pts',(-0.184229120115131,-0.149384714942885,
-1.16530935446074));
#78721=CARTESIAN_POINT('Ctrl Pts',(-0.18551022869534,-0.147790789655864,
-1.16545074836913));
#78722=CARTESIAN_POINT('Ctrl Pts',(-0.18740117947556,-0.14537477514018,
-1.16566086820921));
#78723=CARTESIAN_POINT('Ctrl Pts',(-0.188026539320907,-0.144565030089082,
-1.16573059779801));
#78724=CARTESIAN_POINT('Ctrl Pts',(-0.189149524688123,-0.143091321584795,
-1.16585621514323));
#78725=CARTESIAN_POINT('Ctrl Pts',(-0.189648921470875,-0.142428773909899,
-1.16591222106481));
#78726=CARTESIAN_POINT('Ctrl Pts',(-0.190770039981206,-0.140925038532919,
-1.16603828443429));
#78727=CARTESIAN_POINT('Ctrl Pts',(-0.191389684195424,-0.140082345521155,
-1.16610820071153));
#78728=CARTESIAN_POINT('Ctrl Pts',(-0.193272994339512,-0.137485289113059,
-1.16632153956532));
#78729=CARTESIAN_POINT('Ctrl Pts',(-0.194518303713542,-0.135717667936478,
-1.16646378662279));
#78730=CARTESIAN_POINT('Ctrl Pts',(-0.2043231189953,-0.121388225878524,
-1.16759558719514));
#78731=CARTESIAN_POINT('Ctrl Pts',(-0.211682254887129,-0.108045310553759,
-1.16852086338635));
#78732=CARTESIAN_POINT('Ctrl Pts',(-0.219536415776316,-0.0898712726390406,
-1.16973519403368));
#78733=CARTESIAN_POINT('Ctrl Pts',(-0.221235864916009,-0.0856024209953103,
-1.17001719864522));
#78734=CARTESIAN_POINT('Ctrl Pts',(-0.22538682782221,-0.0742244959781561,
-1.17076543685948));
#78735=CARTESIAN_POINT('Ctrl Pts',(-0.227625990001952,-0.0670439712040082,
-1.17123435290941));
#78736=CARTESIAN_POINT('Ctrl Pts',(-0.230794433838549,-0.0548768814839222,
-1.17203453332438));
#78737=CARTESIAN_POINT('Ctrl Pts',(-0.231911701121949,-0.049944968578224,
-1.17236034231648));
#78738=CARTESIAN_POINT('Ctrl Pts',(-0.233263025845686,-0.042949105542025,
-1.17282652693108));
#78739=CARTESIAN_POINT('Ctrl Pts',(-0.233628951144174,-0.040911827545721,
-1.17296275568478));
#78740=CARTESIAN_POINT('Ctrl Pts',(-0.234215009495198,-0.0373842038365646,
-1.17319957684469));
#78741=CARTESIAN_POINT('Ctrl Pts',(-0.234447697850059,-0.035896046635954,
-1.17329976777564));
#78742=CARTESIAN_POINT('Ctrl Pts',(-0.234895422259891,-0.032842323901222,
-1.17350599373551));
#78743=CARTESIAN_POINT('Ctrl Pts',(-0.235109017354494,-0.0312766268589381,
-1.17361206872707));
#78744=CARTESIAN_POINT('Ctrl Pts',(-0.235613546912353,-0.0272805471644105,
-1.17388372019997));
#78745=CARTESIAN_POINT('Ctrl Pts',(-0.235882526191231,-0.0248476316797227,
-1.17404997451111));
#78746=CARTESIAN_POINT('Ctrl Pts',(-0.236826541015641,-0.0149018788751919,
-1.1747333856812));
#78747=CARTESIAN_POINT('Ctrl Pts',(-0.237180585799741,-0.00736375334486454,
-1.17526029872133));
#78748=CARTESIAN_POINT('Ctrl Pts',(-0.237164963147181,0.0134802090323218,
-1.17674180571664));
#78749=CARTESIAN_POINT('Ctrl Pts',(-0.23603586025259,0.0267572040969771,
-1.17771438393518));
#78750=CARTESIAN_POINT('Ctrl Pts',(-0.231890173455107,0.05106891107705,
-1.17951314255089));
#78751=CARTESIAN_POINT('Ctrl Pts',(-0.229177530975958,0.0621192629928734,
-1.18033721590058));
#78752=CARTESIAN_POINT('Ctrl Pts',(-0.225153259850731,0.0745718067036157,
-1.18124576340917));
#78753=CARTESIAN_POINT('Ctrl Pts',(-0.22460598772417,0.0762043009547344,
-1.1813644463234));
#78754=CARTESIAN_POINT('Ctrl Pts',(-0.223723736382412,0.0787439198990912,
-1.1815482569367));
#78755=CARTESIAN_POINT('Ctrl Pts',(-0.223400918027898,0.0796551633578571,
-1.18161404389417));
#78756=CARTESIAN_POINT('Ctrl Pts',(-0.222817310851792,0.0812710965069608,
-1.18173037775845));
#78757=CARTESIAN_POINT('Ctrl Pts',(-0.222558741407624,0.0819765319401293,
-1.18178104865724));
#78758=CARTESIAN_POINT('Ctrl Pts',(-0.221923449729732,0.0836845873412313,
-1.18190347199583));
#78759=CARTESIAN_POINT('Ctrl Pts',(-0.221543282633284,0.084685900413273,
-1.18197502112334));
#78760=CARTESIAN_POINT('Ctrl Pts',(-0.220327251874794,0.0878245369980222,
-1.18219870654821));
#78761=CARTESIAN_POINT('Ctrl Pts',(-0.21946711455013,0.0899523974241675,
-1.18234949633113));
#78762=CARTESIAN_POINT('Ctrl Pts',(-0.214660259358054,0.101364282332333,
-1.18315527501331));
#78763=CARTESIAN_POINT('Ctrl Pts',(-0.210154719831366,0.11040282790138,
-1.18378319822383));
#78764=CARTESIAN_POINT('Ctrl Pts',(-0.195708108043289,0.13527366252212,
-1.18555517197028));
#78765=CARTESIAN_POINT('Ctrl Pts',(-0.184456672933163,0.150254158165038,
-1.18668276027806));
#78766=CARTESIAN_POINT('Ctrl Pts',(-0.168855845418044,0.166598567304544,
-1.18813307580829));
#78767=CARTESIAN_POINT('Ctrl Pts',(-0.166076516447608,0.169369321325349,
-1.18838756609604));
#78768=CARTESIAN_POINT('Ctrl Pts',(-0.161866074459566,0.173363456895554,
-1.18876839769736));
#78769=CARTESIAN_POINT('Ctrl Pts',(-0.160486991618448,0.174640887053243,
-1.18889242017034));
#78770=CARTESIAN_POINT('Ctrl Pts',(-0.157995729885839,0.176894088274434,
-1.18911529286234));
#78771=CARTESIAN_POINT('Ctrl Pts',(-0.156889318883804,0.177876110198741,
-1.18921387324091));
#78772=CARTESIAN_POINT('Ctrl Pts',(-0.154518828904213,0.179940773423516,
-1.18942428197248));
#78773=CARTESIAN_POINT('Ctrl Pts',(-0.153252401354669,0.181020583527869,
-1.18953621966753));
#78774=CARTESIAN_POINT('Ctrl Pts',(-0.149791691648096,0.183908986331325,
-1.18984090462305));
#78775=CARTESIAN_POINT('Ctrl Pts',(-0.147576137778808,0.185691541213951,
-1.19003468315785));
#78776=CARTESIAN_POINT('Ctrl Pts',(-0.132429907503383,0.197435363255094,
-1.1913514468248));
#78777=CARTESIAN_POINT('Ctrl Pts',(-0.118535028197694,0.206076842626899,
-1.19252554982149));
#78778=CARTESIAN_POINT('Ctrl Pts',(-0.0909763132200518,0.219501395551439,
-1.19476145484212));
#78779=CARTESIAN_POINT('Ctrl Pts',(-0.077542711279048,0.224599080845148,
-1.19581385467492));
#78780=CARTESIAN_POINT('Ctrl Pts',(-0.0615844206030869,0.229050871030349,
-1.19697127888527));
#78781=CARTESIAN_POINT('Ctrl Pts',(-0.0594304186414556,0.229619181719115,
-1.19712557344875));
#78782=CARTESIAN_POINT('Ctrl Pts',(-0.0562415411308435,0.230412651372072,
-1.19735084695065));
#78783=CARTESIAN_POINT('Ctrl Pts',(-0.0552127230172826,0.230661345235265,
-1.19742304571925));
#78784=CARTESIAN_POINT('Ctrl Pts',(-0.0533741286526486,0.231092777980647,
-1.19755117394801));
#78785=CARTESIAN_POINT('Ctrl Pts',(-0.0525650207246063,0.231278162187507,
-1.19760724729238));
#78786=CARTESIAN_POINT('Ctrl Pts',(-0.0507673437369217,0.231680127535726,
-1.19773113934569));
#78787=CARTESIAN_POINT('Ctrl Pts',(-0.0497783466183655,0.231894633372684,
-1.19779884161479));
#78788=CARTESIAN_POINT('Ctrl Pts',(-0.0468414856311332,0.232511961224511,
-1.1979986139317));
#78789=CARTESIAN_POINT('Ctrl Pts',(-0.0448898384669629,0.232896629276128,
-1.1981297151378));
#78790=CARTESIAN_POINT('Ctrl Pts',(-0.0426010743960498,0.233317901883917,
-1.19828177758529));
#78791=CARTESIAN_POINT('Ctrl Pts',(-0.0422685137818562,0.233378378649217,
-1.19830383099465));
#78792=CARTESIAN_POINT('Ctrl Pts',(-0.0419358257152316,0.23343814415511,
-1.19832585242651));
#78793=CARTESIAN_POINT('',(-0.237175055044089,5.9077571581536E-5,-1.19544314726977));
#78794=CARTESIAN_POINT('Ctrl Pts',(-0.0419358439263085,0.233438140883593,
-1.21800162451869));
#78795=CARTESIAN_POINT('Ctrl Pts',(-0.0481832754706132,0.232315825082111,
-1.21755312230286));
#78796=CARTESIAN_POINT('Ctrl Pts',(-0.0543849249259875,0.230942845640307,
-1.21709801040124));
#78797=CARTESIAN_POINT('Ctrl Pts',(-0.0660051115692908,0.227875887400181,
-1.21622856511696));
#78798=CARTESIAN_POINT('Ctrl Pts',(-0.0714306853965034,0.226233836549135,
-1.21581554198375));
#78799=CARTESIAN_POINT('Ctrl Pts',(-0.0891987386654505,0.220153392967026,
-1.21444481671099));
#78800=CARTESIAN_POINT('Ctrl Pts',(-0.101233010577412,0.214885713774959,
-1.21348563312763));
#78801=CARTESIAN_POINT('Ctrl Pts',(-0.114769745884238,0.207569382010105,
-1.21241010430238));
#78802=CARTESIAN_POINT('Ctrl Pts',(-0.116753015793813,0.206460352526113,
-1.2122526592125));
#78803=CARTESIAN_POINT('Ctrl Pts',(-0.11964347709157,0.204789053961714,
-1.21202371936478));
#78804=CARTESIAN_POINT('Ctrl Pts',(-0.120563234595947,0.204248928532995,
-1.21195094906331));
#78805=CARTESIAN_POINT('Ctrl Pts',(-0.122192397466522,0.203277366927712,
-1.21182223547746));
#78806=CARTESIAN_POINT('Ctrl Pts',(-0.12290321702151,0.20284838973218,-1.21176614228712));
#78807=CARTESIAN_POINT('Ctrl Pts',(-0.124469105945273,0.201892127998671,
-1.21164272055101));
#78808=CARTESIAN_POINT('Ctrl Pts',(-0.125323091549005,0.201363135899676,
-1.21157550308749));
#78809=CARTESIAN_POINT('Ctrl Pts',(-0.127827451402393,0.199789733597376,
-1.2113785784341));
#78810=CARTESIAN_POINT('Ctrl Pts',(-0.129468362186863,0.198730316712671,
-1.21124979946835));
#78811=CARTESIAN_POINT('Ctrl Pts',(-0.142141382055089,0.19032466504217,
-1.2102556299785));
#78812=CARTESIAN_POINT('Ctrl Pts',(-0.152554743999959,0.182084586471879,
-1.20944039810114));
#78813=CARTESIAN_POINT('Ctrl Pts',(-0.174527780677602,0.161481922963948,
-1.20759224170489));
#78814=CARTESIAN_POINT('Ctrl Pts',(-0.185562908911338,0.148669732259347,
-1.20656311849887));
#78815=CARTESIAN_POINT('Ctrl Pts',(-0.196889356537466,0.13227234268149,
-1.20527819735666));
#78816=CARTESIAN_POINT('Ctrl Pts',(-0.198583650983616,0.129714777650927,
-1.20507876298616));
#78817=CARTESIAN_POINT('Ctrl Pts',(-0.201241433686387,0.12552865123598,
-1.20475344088543));
#78818=CARTESIAN_POINT('Ctrl Pts',(-0.202235906231281,0.123920114589567,
-1.20462869233618));
#78819=CARTESIAN_POINT('Ctrl Pts',(-0.203974265404521,0.121031692420664,
-1.20440504446034));
#78820=CARTESIAN_POINT('Ctrl Pts',(-0.204725613153335,0.119756397185868,
-1.20430642288659));
#78821=CARTESIAN_POINT('Ctrl Pts',(-0.206292546161303,0.117038928817861,
-1.20409648953868));
#78822=CARTESIAN_POINT('Ctrl Pts',(-0.207105051777241,0.115595080984363,
-1.20398507378913));
#78823=CARTESIAN_POINT('Ctrl Pts',(-0.209254465579841,0.111680091186355,
-1.20368324331998));
#78824=CARTESIAN_POINT('Ctrl Pts',(-0.210562664326068,0.109193577408518,
-1.20349182968687));
#78825=CARTESIAN_POINT('Ctrl Pts',(-0.21336296895045,0.10363346077934,-1.20306426403028));
#78826=CARTESIAN_POINT('Ctrl Pts',(-0.214833430602607,0.100549717870182,
-1.20282742691546));
#78827=CARTESIAN_POINT('Ctrl Pts',(-0.219273659906438,0.0906955952659816,
-1.2020714177945));
#78828=CARTESIAN_POINT('Ctrl Pts',(-0.221993572046388,0.0838180506411659,
-1.20154479707658));
#78829=CARTESIAN_POINT('Ctrl Pts',(-0.229817428001329,0.0609664895496733,
-1.19980267347884));
#78830=CARTESIAN_POINT('Ctrl Pts',(-0.233550414748087,0.0445774651567908,
-1.19856149451342));
#78831=CARTESIAN_POINT('Ctrl Pts',(-0.236056795047792,0.0234435553854519,
-1.19704415606684));
#78832=CARTESIAN_POINT('Ctrl Pts',(-0.236460734547928,0.0189403817494118,
-1.1967258311806));
#78833=CARTESIAN_POINT('Ctrl Pts',(-0.236822474981413,0.0130049531258889,
-1.19631503900962));
#78834=CARTESIAN_POINT('Ctrl Pts',(-0.236896377527786,0.0115810201544257,
-1.19621715202846));
#78835=CARTESIAN_POINT('Ctrl Pts',(-0.236995636875841,0.00926522985563239,
-1.19605912546995));
#78836=CARTESIAN_POINT('Ctrl Pts',(-0.237028809321001,0.00837376861655289,
-1.19599857498779));
#78837=CARTESIAN_POINT('Ctrl Pts',(-0.23708153664459,0.00670320283296535,
-1.19588565963598));
#78838=CARTESIAN_POINT('Ctrl Pts',(-0.237102282419113,0.00592415785210215,
-1.19583323006463));
#78839=CARTESIAN_POINT('Ctrl Pts',(-0.237138178825484,0.00426979397335219,
-1.19572234715988));
#78840=CARTESIAN_POINT('Ctrl Pts',(-0.237152323864252,0.00339445763363649,
-1.19566394869549));
#78841=CARTESIAN_POINT('Ctrl Pts',(-0.23717033193529,0.0016990446880916,
-1.19555132749142));
#78842=CARTESIAN_POINT('Ctrl Pts',(-0.237174788959285,0.000878991296439202,
-1.19549707534045));
#78843=CARTESIAN_POINT('Ctrl Pts',(-0.237174992681668,5.89190195836492E-5,
-1.19544302870655));
#78844=CARTESIAN_POINT('Ctrl Pts',(-0.237174992640464,5.90846497784872E-5,
-1.19544303962237));
#78845=CARTESIAN_POINT('Ctrl Pts',(-0.23717571343138,-0.00283428242356205,
-1.19525235297691));
#78846=CARTESIAN_POINT('Ctrl Pts',(-0.237123488630181,-0.00572759877968307,
-1.19506424287379));
#78847=CARTESIAN_POINT('Ctrl Pts',(-0.236503771768316,-0.0227687045973912,
-1.19396767567369));
#78848=CARTESIAN_POINT('Ctrl Pts',(-0.234723191033778,-0.0368450523929681,
-1.19310682893217));
#78849=CARTESIAN_POINT('Ctrl Pts',(-0.228534035968796,-0.0651406092883096,
-1.19132962795524));
#78850=CARTESIAN_POINT('Ctrl Pts',(-0.224024566439007,-0.0792718214660879,
-1.19041554110495));
#78851=CARTESIAN_POINT('Ctrl Pts',(-0.217087957597159,-0.0955681589639875,
-1.18926820578326));
#78852=CARTESIAN_POINT('Ctrl Pts',(-0.215898705552173,-0.0982252619154099,
-1.18907811239317));
#78853=CARTESIAN_POINT('Ctrl Pts',(-0.213947213138157,-0.102378645776983,
-1.18877581340901));
#78854=CARTESIAN_POINT('Ctrl Pts',(-0.213217447541096,-0.103889927045731,
-1.18866472045405));
#78855=CARTESIAN_POINT('Ctrl Pts',(-0.211815496879125,-0.106716243866289,
-1.1884548233863));
#78856=CARTESIAN_POINT('Ctrl Pts',(-0.211146944919434,-0.108032999148215,
-1.18835614948209));
#78857=CARTESIAN_POINT('Ctrl Pts',(-0.209610349512394,-0.110990665758213,
-1.18813245925699));
#78858=CARTESIAN_POINT('Ctrl Pts',(-0.208735258496133,-0.112627785331814,
-1.18800719958805));
#78859=CARTESIAN_POINT('Ctrl Pts',(-0.20642100083665,-0.116837668412553,
-1.18768125377528));
#78860=CARTESIAN_POINT('Ctrl Pts',(-0.204952961038353,-0.119394106865174,
-1.18747955674621));
#78861=CARTESIAN_POINT('Ctrl Pts',(-0.192409671674333,-0.140323629130649,
-1.18579613848267));
#78862=CARTESIAN_POINT('Ctrl Pts',(-0.178937578504926,-0.157140627398603,
-1.18422224984896));
#78863=CARTESIAN_POINT('Ctrl Pts',(-0.1587849526264,-0.176294504272544,
-1.182200873858));
#78864=CARTESIAN_POINT('Ctrl Pts',(-0.154001323005728,-0.180488271378968,
-1.18174171122945));
#78865=CARTESIAN_POINT('Ctrl Pts',(-0.14706719896306,-0.18609069837606,
-1.18110989233811));
#78866=CARTESIAN_POINT('Ctrl Pts',(-0.145053844145608,-0.187664307944215,
-1.180930210797));
#78867=CARTESIAN_POINT('Ctrl Pts',(-0.141906397311298,-0.19004338318521,
-1.1806555400361));
#78868=CARTESIAN_POINT('Ctrl Pts',(-0.140790047312149,-0.190871883434588,
-1.1805592970011));
#78869=CARTESIAN_POINT('Ctrl Pts',(-0.138728450155233,-0.192373970829441,
-1.1803838048426));
#78870=CARTESIAN_POINT('Ctrl Pts',(-0.137785425931719,-0.193050522078221,
-1.18030437688981));
#78871=CARTESIAN_POINT('Ctrl Pts',(-0.136825087547286,-0.193728873097802,
-1.18022437462264));
#78872=CARTESIAN_POINT('Ctrl Pts',(-0.136812724756105,-0.193737603987655,
-1.18022334487149));
#78873=CARTESIAN_POINT('Ctrl Pts',(-0.136788035365436,-0.193755036666225,
-1.18022128867867));
#78874=CARTESIAN_POINT('Ctrl Pts',(-0.136775708772323,-0.19376373846129,
-1.18022026223662));
#78875=CARTESIAN_POINT('Ctrl Pts',(-0.136751078476457,-0.193781122370797,
-1.18021821155198));
#78876=CARTESIAN_POINT('Ctrl Pts',(-0.136738774776263,-0.19378980449045,
-1.18021718730901));
#78877=CARTESIAN_POINT('Ctrl Pts',(-0.136714176725909,-0.193807158622976,
-1.18021513989389));
#78878=CARTESIAN_POINT('Ctrl Pts',(-0.13670188237759,-0.193815830637692,
-1.18021411672162));
#78879=CARTESIAN_POINT('Ctrl Pts',(-0.136677289186981,-0.193833174332872,
-1.18021207029527));
#78880=CARTESIAN_POINT('Ctrl Pts',(-0.136664990344591,-0.1938418460126,
-1.18021104704125));
#78881=CARTESIAN_POINT('Ctrl Pts',(-0.136640373948553,-0.193859199057687,
-1.18020899926902));
#78882=CARTESIAN_POINT('Ctrl Pts',(-0.136628056392239,-0.193867880420062,
-1.180207974751));
#78883=CARTESIAN_POINT('Ctrl Pts',(-0.13660338789969,-0.193885263152169,
-1.18020592323225));
#78884=CARTESIAN_POINT('Ctrl Pts',(-0.136591036958593,-0.193893964516269,
-1.18020489623186));
#78885=CARTESIAN_POINT('Ctrl Pts',(-0.13656628649085,-0.193911397934974,
-1.18020283848658));
#78886=CARTESIAN_POINT('Ctrl Pts',(-0.136553886957918,-0.193920129980571,
-1.18020180774228));
#78887=CARTESIAN_POINT('Ctrl Pts',(-0.136529023470478,-0.193937635871761,
-1.18019974119647));
#78888=CARTESIAN_POINT('Ctrl Pts',(-0.136516559507797,-0.193946409705064,
-1.18019870539578));
#78889=CARTESIAN_POINT('Ctrl Pts',(-0.136491550590124,-0.193964010779834,
-1.18019662736496));
#78890=CARTESIAN_POINT('Ctrl Pts',(-0.136479005624352,-0.193972838005955,
-1.18019558513585));
#78891=CARTESIAN_POINT('Ctrl Pts',(-0.13645381727651,-0.193990558055298,
-1.18019349280672));
#78892=CARTESIAN_POINT('Ctrl Pts',(-0.136441173881835,-0.193999450859234,
-1.180192442708));
#78893=CARTESIAN_POINT('Ctrl Pts',(-0.136415770267691,-0.194017314924671,
-1.18019033311819));
#78894=CARTESIAN_POINT('Ctrl Pts',(-0.136403010031694,-0.194026286164016,
-1.18018927362854));
#78895=CARTESIAN_POINT('Ctrl Pts',(-0.136377353189231,-0.194044320737727,
-1.18018714364286));
#78896=CARTESIAN_POINT('Ctrl Pts',(-0.136364456564841,-0.194053384044809,
-1.18018607314867));
#78897=CARTESIAN_POINT('Ctrl Pts',(-0.136338506092843,-0.194071617285636,
-1.18018391943345));
#78898=CARTESIAN_POINT('Ctrl Pts',(-0.136325452223259,-0.19408078718826,
-1.18018283621449));
#78899=CARTESIAN_POINT('Ctrl Pts',(-0.136299164903168,-0.194099249182386,
-1.18018065520663));
#78900=CARTESIAN_POINT('Ctrl Pts',(-0.136285931427581,-0.194108541237587,
-1.18017955742017));
#78901=CARTESIAN_POINT('Ctrl Pts',(-0.13625926080581,-0.194127264285969,
-1.180177345293));
#78902=CARTESIAN_POINT('Ctrl Pts',(-0.136245823629571,-0.194136695238176,
-1.180176230955));
#78903=CARTESIAN_POINT('Ctrl Pts',(-0.136218719519434,-0.194155714199198,
-1.18017398357752));
#78904=CARTESIAN_POINT('Ctrl Pts',(-0.136205052551574,-0.194165302160654,
-1.1801728505412));
#78905=CARTESIAN_POINT('Ctrl Pts',(-0.136177460464758,-0.194184654840767,
-1.1801705634317));
#78906=CARTESIAN_POINT('Ctrl Pts',(-0.136163535307626,-0.194194419504753,
-1.18016940936219));
#78907=CARTESIAN_POINT('Ctrl Pts',(-0.136135395780618,-0.194214147121066,
-1.1801670776332));
#78908=CARTESIAN_POINT('Ctrl Pts',(-0.136121181366843,-0.1942241100111,
-1.18016589997789));
#78909=CARTESIAN_POINT('Ctrl Pts',(-0.136092429166997,-0.194244257736242,
-1.1801635182714));
#78910=CARTESIAN_POINT('Ctrl Pts',(-0.136077891330581,-0.194254442500297,
-1.18016231422499));
#78911=CARTESIAN_POINT('Ctrl Pts',(-0.136048454515408,-0.194275060107551,
-1.18015987663575));
#78912=CARTESIAN_POINT('Ctrl Pts',(-0.13603355548025,-0.19428549286868,
-1.18015864309847));
#78913=CARTESIAN_POINT('Ctrl Pts',(-0.136003354276113,-0.194306635500447,
-1.18015614308253));
#78914=CARTESIAN_POINT('Ctrl Pts',(-0.135988052040609,-0.194317345278435,
-1.18015487661007));
#78915=CARTESIAN_POINT('Ctrl Pts',(-0.135956997479325,-0.194339074380238,
-1.18015230687368));
#78916=CARTESIAN_POINT('Ctrl Pts',(-0.135941245078386,-0.194350093596838,
-1.18015100361697));
#78917=CARTESIAN_POINT('Ctrl Pts',(-0.135916103532947,-0.19436767621355,
-1.18014892394344));
#78918=CARTESIAN_POINT('Ctrl Pts',(-0.135906715257174,-0.194374240845436,
-1.18014814744364));
#78919=CARTESIAN_POINT('Ctrl Pts',(-0.135239915317502,-0.194840420256555,
-1.18009300279612));
#78920=CARTESIAN_POINT('Ctrl Pts',(-0.134580187697683,-0.195296690146628,
-1.18003886439368));
#78921=CARTESIAN_POINT('Ctrl Pts',(-0.133054832223663,-0.196340231067417,
-1.17991465064266));
#78922=CARTESIAN_POINT('Ctrl Pts',(-0.132187621147164,-0.19692513204853,
-1.17984473241733));
#78923=CARTESIAN_POINT('Ctrl Pts',(-0.129515197985657,-0.198701971352152,
-1.1796313176645));
#78924=CARTESIAN_POINT('Ctrl Pts',(-0.127697468455801,-0.199875004154864,
-1.17948899818403));
#78925=CARTESIAN_POINT('Ctrl Pts',(-0.113099343294529,-0.209015132386064,
-1.17836629878244));
#78926=CARTESIAN_POINT('Ctrl Pts',(-0.0996007901584415,-0.215774406846182,
-1.17744899296487));
#78927=CARTESIAN_POINT('Ctrl Pts',(-0.0709712821265411,-0.226846664402345,
-1.17556638437772));
#78928=CARTESIAN_POINT('Ctrl Pts',(-0.0558721049781062,-0.231029342004321,
-1.17460397910813));
#78929=CARTESIAN_POINT('Ctrl Pts',(-0.0376354152584684,-0.234187628086533,
-1.17340462834023));
#78930=CARTESIAN_POINT('Ctrl Pts',(-0.0347899742566997,-0.234627206767253,
-1.17321657150095));
#78931=CARTESIAN_POINT('Ctrl Pts',(-0.0302810581251585,-0.235239945699456,
-1.17291677210019));
#78932=CARTESIAN_POINT('Ctrl Pts',(-0.0286224864007411,-0.235447504904431,
-1.17280611060909));
#78933=CARTESIAN_POINT('Ctrl Pts',(-0.0254937732926261,-0.235805495581379,
-1.17259657511645));
#78934=CARTESIAN_POINT('Ctrl Pts',(-0.0240241436796043,-0.235959752021114,
-1.17249782632186));
#78935=CARTESIAN_POINT('Ctrl Pts',(-0.0206949118531588,-0.236277772929812,
-1.17227334534506));
#78936=CARTESIAN_POINT('Ctrl Pts',(-0.0188346438174366,-0.236433333529347,
-1.17214736276259));
#78937=CARTESIAN_POINT('Ctrl Pts',(-0.0131272684522955,-0.23684281605482,
-1.17175906349662));
#78938=CARTESIAN_POINT('Ctrl Pts',(-0.00927581123095014,-0.23702489532715,
-1.17149454497683));
#78939=CARTESIAN_POINT('Ctrl Pts',(0.0133253485765188,-0.237541692357222,
-1.16992688982243));
#78940=CARTESIAN_POINT('Ctrl Pts',(0.0320543621561828,-0.235745406568818,
-1.16855804385412));
#78941=CARTESIAN_POINT('Ctrl Pts',(0.0602544759826042,-0.229616307893173,
-1.16645403396751));
#78942=CARTESIAN_POINT('Ctrl Pts',(0.0699901438947053,-0.226838422821999,
-1.16572112293165));
#78943=CARTESIAN_POINT('Ctrl Pts',(0.0816837076881318,-0.22267696206279,
-1.16485331695987));
#78944=CARTESIAN_POINT('Ctrl Pts',(0.0838366973694974,-0.221875340411693,
-1.16469409794925));
#78945=CARTESIAN_POINT('Ctrl Pts',(0.0869761781877329,-0.220654192397584,
-1.16446309039073));
#78946=CARTESIAN_POINT('Ctrl Pts',(0.0879719415245645,-0.220259087918213,
-1.16438999452244));
#78947=CARTESIAN_POINT('Ctrl Pts',(0.089661337720843,-0.219575475398744,
-1.16426631893732));
#78948=CARTESIAN_POINT('Ctrl Pts',(0.0903563204855477,-0.219290401716164,
-1.16421554083563));
#78949=CARTESIAN_POINT('Ctrl Pts',(0.0919419634242805,-0.218631171543051,
-1.16409992172058));
#78950=CARTESIAN_POINT('Ctrl Pts',(0.0928317048229706,-0.218254870440072,
-1.16403520992679));
#78951=CARTESIAN_POINT('Ctrl Pts',(0.0952985530389372,-0.217193744214037,
-1.16385618567953));
#78952=CARTESIAN_POINT('Ctrl Pts',(0.0968705862958924,-0.216497174735559,
-1.16374254794702));
#78953=CARTESIAN_POINT('Ctrl Pts',(0.108613919945221,-0.211140164870983,
-1.16289601318515));
#78954=CARTESIAN_POINT('Ctrl Pts',(0.118452973115967,-0.205781709215421,
-1.16219976709747));
#78955=CARTESIAN_POINT('Ctrl Pts',(0.135296045942244,-0.19499882471013,
-1.16096824065607));
#78956=CARTESIAN_POINT('Ctrl Pts',(0.142443785311366,-0.18984027509809,
-1.16043125136447));
#78957=CARTESIAN_POINT('Ctrl Pts',(0.155361903658598,-0.179376026077553,
-1.15940545020663));
#78958=CARTESIAN_POINT('Ctrl Pts',(0.16118842765626,-0.174158999298415,
-1.15891869467996));
#78959=CARTESIAN_POINT('Ctrl Pts',(0.169263964329329,-0.166175278172396,
-1.15819665200071));
#78960=CARTESIAN_POINT('Ctrl Pts',(0.171725297880547,-0.163630476480484,
-1.15796960016637));
#78961=CARTESIAN_POINT('Ctrl Pts',(0.17608987934439,-0.158910914797117,
-1.15755307494382));
#78962=CARTESIAN_POINT('Ctrl Pts',(0.178012113622753,-0.156754619310853,
-1.15736441129175));
#78963=CARTESIAN_POINT('Ctrl Pts',(0.180985026645301,-0.153294492364698,
-1.15706386707515));
#78964=CARTESIAN_POINT('Ctrl Pts',(0.182062141361734,-0.152013676031831,
-1.15695307694633));
#78965=CARTESIAN_POINT('Ctrl Pts',(0.184064461264845,-0.149580872621275,
-1.15674343442754));
#78966=CARTESIAN_POINT('Ctrl Pts',(0.184992635775463,-0.148431424887543,
-1.15664470874059));
#78967=CARTESIAN_POINT('Ctrl Pts',(0.187067185084337,-0.145812625829884,
-1.15642046733574));
#78968=CARTESIAN_POINT('Ctrl Pts',(0.188207090294475,-0.144338298471596,
-1.15629470335024));
#78969=CARTESIAN_POINT('Ctrl Pts',(0.19164138993426,-0.139786594999662,
-1.15590778747334));
#78970=CARTESIAN_POINT('Ctrl Pts',(0.193878453539476,-0.136666955606424,
-1.15564445654857));
#78971=CARTESIAN_POINT('Ctrl Pts',(0.206604223226656,-0.117978975412042,
-1.1540768581113));
#78972=CARTESIAN_POINT('Ctrl Pts',(0.215288743854662,-0.101266271111253,
-1.15270666238492));
#78973=CARTESIAN_POINT('Ctrl Pts',(0.225483045351733,-0.0742412920769977,
-1.15060079122418));
#78974=CARTESIAN_POINT('Ctrl Pts',(0.228445234185086,-0.0645537589485454,
-1.14986742452374));
#78975=CARTESIAN_POINT('Ctrl Pts',(0.23130966592657,-0.0524699799103707,
-1.14899914651404));
#78976=CARTESIAN_POINT('Ctrl Pts',(0.231807164342592,-0.0502264858064748,
-1.14883988428649));
#78977=CARTESIAN_POINT('Ctrl Pts',(0.232488717182714,-0.0469268027877572,
-1.14860882638611));
#78978=CARTESIAN_POINT('Ctrl Pts',(0.232698326629021,-0.0458761085165478,
-1.14853572261445));
#78979=CARTESIAN_POINT('Ctrl Pts',(0.233042780784099,-0.0440863609553087,
-1.14841203822367));
#78980=CARTESIAN_POINT('Ctrl Pts',(0.233181243354767,-0.0433480415182524,
-1.1483612591427));
#78981=CARTESIAN_POINT('Ctrl Pts',(0.233489734654157,-0.0416588222514061,
-1.1482456441009));
#78982=CARTESIAN_POINT('Ctrl Pts',(0.233657464882031,-0.04070752814505,
-1.14818093730115));
#78983=CARTESIAN_POINT('Ctrl Pts',(0.234107519078384,-0.0380605447374178,
-1.14800194062593));
#78984=CARTESIAN_POINT('Ctrl Pts',(0.23437723378552,-0.03636273172241,-1.14788832513783));
#78985=CARTESIAN_POINT('Ctrl Pts',(0.236258131354591,-0.0236308883771642,
-1.14704424307061));
#78986=CARTESIAN_POINT('Ctrl Pts',(0.237108022606951,-0.0124969777036749,
-1.14635018056881));
#78987=CARTESIAN_POINT('Ctrl Pts',(0.237222106362764,0.00764528731840521,
-1.14510970813887));
#78988=CARTESIAN_POINT('Ctrl Pts',(0.236761988005263,0.0166294764994894,
-1.14456182047828));
#78989=CARTESIAN_POINT('Ctrl Pts',(0.234785677560178,0.0348569184840514,
-1.14343013261823));
#78990=CARTESIAN_POINT('Ctrl Pts',(0.233230126660741,0.0440795023206173,
-1.1428467093291));
#78991=CARTESIAN_POINT('Ctrl Pts',(0.230231859226091,0.0571093858675861,
-1.14198920209376));
#78992=CARTESIAN_POINT('Ctrl Pts',(0.229229278212034,0.0610092281020387,
-1.14172825093923));
#78993=CARTESIAN_POINT('Ctrl Pts',(0.227608727782022,0.066707199742506,
-1.14133963830574));
#78994=CARTESIAN_POINT('Ctrl Pts',(0.227067595627987,0.0685265651250507,
-1.14121443980705));
#78995=CARTESIAN_POINT('Ctrl Pts',(0.226065495052678,0.0717535068402572,
-1.1409902932548));
#78996=CARTESIAN_POINT('Ctrl Pts',(0.225613064297506,0.073163644289787,
-1.14089162772368));
#78997=CARTESIAN_POINT('Ctrl Pts',(0.2246278283599,0.0761383671523528,-1.14068192555849));
#78998=CARTESIAN_POINT('Ctrl Pts',(0.22409181696016,0.0777017989396298,
-1.14057078799549));
#78999=CARTESIAN_POINT('Ctrl Pts',(0.222606912065868,0.0818897519950092,
-1.14027052747034));
#79000=CARTESIAN_POINT('Ctrl Pts',(0.221627988211237,0.0845032689838849,
-1.14008042344662));
#79001=CARTESIAN_POINT('Ctrl Pts',(0.215219142871203,0.100735544230943,
-1.13888207996312));
#79002=CARTESIAN_POINT('Ctrl Pts',(0.208583204862185,0.113841282203137,
-1.13783325996404));
#79003=CARTESIAN_POINT('Ctrl Pts',(0.194432690161524,0.136345766527621,
-1.13589853544609));
#79004=CARTESIAN_POINT('Ctrl Pts',(0.187331109504395,0.14594967601894,-1.13502216821175));
#79005=CARTESIAN_POINT('Ctrl Pts',(0.175973922020966,0.159106548687766,
-1.13377662396129));
#79006=CARTESIAN_POINT('Ctrl Pts',(0.172269160985255,0.163110580995786,
-1.13339089834269));
#79007=CARTESIAN_POINT('Ctrl Pts',(0.167395270323038,0.168026668420938,
-1.13291231818626));
#79008=CARTESIAN_POINT('Ctrl Pts',(0.166351499667832,0.169060097773275,
-1.13281142126191));
#79009=CARTESIAN_POINT('Ctrl Pts',(0.164651716452049,0.17071205433796,-1.1326497582156));
#79010=CARTESIAN_POINT('Ctrl Pts',(0.16400167919979,0.171336635063889,-1.13258854688121));
#79011=CARTESIAN_POINT('Ctrl Pts',(0.162732234401276,0.172542522364348,
-1.13247021972754));
#79012=CARTESIAN_POINT('Ctrl Pts',(0.162113242334103,0.17312422946334,-1.1324130753917));
#79013=CARTESIAN_POINT('Ctrl Pts',(0.160565818415407,0.174562867857997,
-1.13227154946347));
#79014=CARTESIAN_POINT('Ctrl Pts',(0.159633621480794,0.175415746007112,
-1.13218746777091));
#79015=CARTESIAN_POINT('Ctrl Pts',(0.15627488324745,0.178439745861253,-1.13188850171064));
#79016=CARTESIAN_POINT('Ctrl Pts',(0.153810387821108,0.18056840574687,-1.13167647401497));
#79017=CARTESIAN_POINT('Ctrl Pts',(0.138141201076488,0.193548669630834,
-1.13036770839144));
#79018=CARTESIAN_POINT('Ctrl Pts',(0.123838347104174,0.202998216631934,
-1.12934041704827));
#79019=CARTESIAN_POINT('Ctrl Pts',(0.101371473007988,0.214575655586314,
-1.12778297015812));
#79020=CARTESIAN_POINT('Ctrl Pts',(0.0939119077846063,0.217943630893141,
-1.12727458701274));
#79021=CARTESIAN_POINT('Ctrl Pts',(0.0813055343578469,0.222867828632727,
-1.12641498976776));
#79022=CARTESIAN_POINT('Ctrl Pts',(0.0762531265663769,0.224646639916416,
-1.12607042489111));
#79023=CARTESIAN_POINT('Ctrl Pts',(0.069128485665901,0.226886980855791,
-1.12558207963748));
#79024=CARTESIAN_POINT('Ctrl Pts',(0.0671035072269477,0.22749410641624,
-1.12544301642279));
#79025=CARTESIAN_POINT('Ctrl Pts',(0.0636151842462336,0.228489343394919,
-1.12520287314986));
#79026=CARTESIAN_POINT('Ctrl Pts',(0.0621557195680453,0.228890668346634,
-1.12510222639941));
#79027=CARTESIAN_POINT('Ctrl Pts',(0.059178380292214,0.229678804571674,
-1.12489650311316));
#79028=CARTESIAN_POINT('Ctrl Pts',(0.0576603177507672,0.23006460292077,
-1.12479139959907));
#79029=CARTESIAN_POINT('Ctrl Pts',(0.0538236818327608,0.230999282853407,
-1.12452518422509));
#79030=CARTESIAN_POINT('Ctrl Pts',(0.0515004974405383,0.231528303774867,
-1.12436344715271));
#79031=CARTESIAN_POINT('Ctrl Pts',(0.0423794431009992,0.233461224261411,
-1.12372614550876));
#79032=CARTESIAN_POINT('Ctrl Pts',(0.0355298387196741,0.23460130896958,
-1.12324243105599));
#79033=CARTESIAN_POINT('Ctrl Pts',(0.0131211319716126,0.23732727781197,
-1.12164312504461));
#79034=CARTESIAN_POINT('Ctrl Pts',(-0.00254581916659853,0.237675876068617,
-1.12049590675736));
#79035=CARTESIAN_POINT('Ctrl Pts',(-0.0248166681487722,0.235968378843026,
-1.11887035590126));
#79036=CARTESIAN_POINT('Ctrl Pts',(-0.0314781245514314,0.235172451103579,
-1.11838538808268));
#79037=CARTESIAN_POINT('Ctrl Pts',(-0.0393785578008861,0.233886714018427,
-1.11781750139299));
#79038=CARTESIAN_POINT('Ctrl Pts',(-0.0406581203423751,0.233667676608155,
-1.11772575923853));
#79039=CARTESIAN_POINT('Ctrl Pts',(-0.041935825738619,0.233438144150908,
-1.1176344235547));
#79040=CARTESIAN_POINT('Origin',(0.,0.,-1.7456589891905));
#79041=CARTESIAN_POINT('',(-0.0419358256939468,0.233438144158933,-0.997911004226539));
#79042=CARTESIAN_POINT('',(-0.0419358384531382,0.233438141866817,-1.01783655831731));
#79043=CARTESIAN_POINT('',(-0.0419358257166344,0.233438144154858,-1.7456589891905));
#79044=CARTESIAN_POINT('',(-0.237174940775019,-0.000167610758756324,-1.07580646542871));
#79045=CARTESIAN_POINT('Ctrl Pts',(-0.0419358256939468,0.233438144158933,
-0.997911004226539));
#79046=CARTESIAN_POINT('Ctrl Pts',(-0.0395037055194274,0.233875060619492,
-0.998070885658115));
#79047=CARTESIAN_POINT('Ctrl Pts',(-0.0370649471817316,0.234273933759101,
-0.998231859080892));
#79048=CARTESIAN_POINT('Ctrl Pts',(-0.0327621878678806,0.234908807711934,
-0.998517273008057));
#79049=CARTESIAN_POINT('Ctrl Pts',(-0.0309007925650829,0.235160901460861,
-0.998641204004634));
#79050=CARTESIAN_POINT('Ctrl Pts',(-0.0275685550342167,0.235571949680004,
-0.998863976190943));
#79051=CARTESIAN_POINT('Ctrl Pts',(-0.0260988342980983,0.235739303854267,
-0.998962548508873));
#79052=CARTESIAN_POINT('Ctrl Pts',(-0.0229715385961057,0.236065799542703,
-0.999173008536609));
#79053=CARTESIAN_POINT('Ctrl Pts',(-0.0213136677327853,0.236221253536087,
-0.999285006236125));
#79054=CARTESIAN_POINT('Ctrl Pts',(-0.0168165544126772,0.23659520873371,
-0.999590030645525));
#79055=CARTESIAN_POINT('Ctrl Pts',(-0.0139748686674424,0.236780047973819,
-0.999784092559481));
#79056=CARTESIAN_POINT('Ctrl Pts',(-0.00765908000192806,0.237076775547993,
-1.00021850949973));
#79057=CARTESIAN_POINT('Ctrl Pts',(-0.00418451024441479,0.237163544281956,
-1.00045958404844));
#79058=CARTESIAN_POINT('Ctrl Pts',(0.00688332156365574,0.237196650520249,
-1.00123425551244));
#79059=CARTESIAN_POINT('Ctrl Pts',(0.0144721234967209,0.236854745070778,
-1.00177571935123));
#79060=CARTESIAN_POINT('Ctrl Pts',(0.0295711457241576,0.235446126494015,
-1.00287056801049));
#79061=CARTESIAN_POINT('Ctrl Pts',(0.0370731570972976,0.234381963261688,
-1.00342330109824));
#79062=CARTESIAN_POINT('Ctrl Pts',(0.0561602198867919,0.230735055215907,
-1.00484176435888));
#79063=CARTESIAN_POINT('Ctrl Pts',(0.0676270761274038,0.227638456918103,
-1.00570614079791));
#79064=CARTESIAN_POINT('Ctrl Pts',(0.0809992281168247,0.222927048008454,
-1.00669762269112));
#79065=CARTESIAN_POINT('Ctrl Pts',(0.083172165866514,0.222125494957821,
-1.0068581628455));
#79066=CARTESIAN_POINT('Ctrl Pts',(0.0863360119806713,0.220905475324993,
-1.00709072135076));
#79067=CARTESIAN_POINT('Ctrl Pts',(0.0873362954927727,0.220511921662653,
-1.00716407077778));
#79068=CARTESIAN_POINT('Ctrl Pts',(0.0891050594726022,0.219802091612276,
-1.00729341487535));
#79069=CARTESIAN_POINT('Ctrl Pts',(0.0898745948312143,0.219488560920778,
-1.00734956525357));
#79070=CARTESIAN_POINT('Ctrl Pts',(0.0915652039246766,0.218789375992474,
-1.00747264774058));
#79071=CARTESIAN_POINT('Ctrl Pts',(0.0924855047009454,0.218401943965069,
-1.00753947342932));
#79072=CARTESIAN_POINT('Ctrl Pts',(0.0951705600999876,0.217251562481697,
-1.00773400616461));
#79073=CARTESIAN_POINT('Ctrl Pts',(0.0969285659546191,0.216472932698964,
-1.00786081896333));
#79074=CARTESIAN_POINT('Ctrl Pts',(0.100966386160027,0.214625506608964,
-1.00815123568739));
#79075=CARTESIAN_POINT('Ctrl Pts',(0.103239069689121,0.213541599673102,
-1.00831406286444));
#79076=CARTESIAN_POINT('Ctrl Pts',(0.111057652169243,0.209658687004037,
-1.00887348328622));
#79077=CARTESIAN_POINT('Ctrl Pts',(0.116510842144015,0.206678013438127,
-1.0092623755141));
#79078=CARTESIAN_POINT('Ctrl Pts',(0.139758560259365,0.192758040598492,
-1.01094119849615));
#79079=CARTESIAN_POINT('Ctrl Pts',(0.156179431548195,0.179711110205591,
-1.01219158069486));
#79080=CARTESIAN_POINT('Ctrl Pts',(0.173287549748883,0.161979968531225,
-1.01377532910191));
#79081=CARTESIAN_POINT('Ctrl Pts',(0.175830562782717,0.159215877948241,
-1.01401914618759));
#79082=CARTESIAN_POINT('Ctrl Pts',(0.179525563313952,0.155003126083689,
-1.01438705624024));
#79083=CARTESIAN_POINT('Ctrl Pts',(0.180728038580167,0.153599390388899,
-1.01450905880859));
#79084=CARTESIAN_POINT('Ctrl Pts',(0.182861322127711,0.151049321250023,
-1.01472973217788));
#79085=CARTESIAN_POINT('Ctrl Pts',(0.183798073446195,0.14990806719247,-1.01482815451542));
#79086=CARTESIAN_POINT('Ctrl Pts',(0.18578059734147,0.147446219615703,-1.01503979342924));
#79087=CARTESIAN_POINT('Ctrl Pts',(0.186823073535118,0.146123088418209,
-1.01515313429471));
#79088=CARTESIAN_POINT('Ctrl Pts',(0.189645521350974,0.142461203614739,
-1.01546578083391));
#79089=CARTESIAN_POINT('Ctrl Pts',(0.191396201537394,0.140100360436919,
-1.01566621162363));
#79090=CARTESIAN_POINT('Ctrl Pts',(0.202109076250495,0.125078084565119,
-1.01693509022905));
#79091=CARTESIAN_POINT('Ctrl Pts',(0.209853328757292,0.111597610748854,
-1.01804904138494));
#79092=CARTESIAN_POINT('Ctrl Pts',(0.22241519543432,0.0837278678197506,
-1.02027734978069));
#79093=CARTESIAN_POINT('Ctrl Pts',(0.227283070624532,0.0694359463824354,
-1.02138508368915));
#79094=CARTESIAN_POINT('Ctrl Pts',(0.231263654141999,0.0526669738965393,
-1.02258830719844));
#79095=CARTESIAN_POINT('Ctrl Pts',(0.231735782018901,0.0505491446729149,
-1.02273851225793));
#79096=CARTESIAN_POINT('Ctrl Pts',(0.232392654371467,0.0473997033287799,
-1.02295899762309));
#79097=CARTESIAN_POINT('Ctrl Pts',(0.232599718162231,0.04637293280376,-1.02303042724171));
#79098=CARTESIAN_POINT('Ctrl Pts',(0.232958608523065,0.044530391475474,
-1.02315775770819));
#79099=CARTESIAN_POINT('Ctrl Pts',(0.233112963382452,0.0437151622787919,
-1.02321379448628));
#79100=CARTESIAN_POINT('Ctrl Pts',(0.233447851712856,0.0418942132404122,
-1.02333829396824));
#79101=CARTESIAN_POINT('Ctrl Pts',(0.23362616763129,0.0408881213423924,
-1.02340663304528));
#79102=CARTESIAN_POINT('Ctrl Pts',(0.234140671618654,0.037871889577955,
-1.02361025670466));
#79103=CARTESIAN_POINT('Ctrl Pts',(0.234457468222649,0.0358584774264697,
-1.0237445157702));
#79104=CARTESIAN_POINT('Ctrl Pts',(0.236651664567177,0.020637841411547,
-1.02474863622168));
#79105=CARTESIAN_POINT('Ctrl Pts',(0.237437993336628,0.00729561798802651,
-1.02556829761763));
#79106=CARTESIAN_POINT('Ctrl Pts',(0.236674537128162,-0.0226565124179727,
-1.02740638068047));
#79107=CARTESIAN_POINT('Ctrl Pts',(0.2345063536851,-0.0391771551577578,
-1.02842145672832));
#79108=CARTESIAN_POINT('Ctrl Pts',(0.229911195095774,-0.0583292898643307,
-1.02969118834136));
#79109=CARTESIAN_POINT('Ctrl Pts',(0.229134509341683,-0.0613093705956127,
-1.02989136937367));
#79110=CARTESIAN_POINT('Ctrl Pts',(0.227786573459721,-0.0660972599727433,
-1.03021768593589));
#79111=CARTESIAN_POINT('Ctrl Pts',(0.227251270761086,-0.0679148762477218,
-1.03034267102888));
#79112=CARTESIAN_POINT('Ctrl Pts',(0.22625888593375,-0.0711413406657514,
-1.03056660613414));
#79113=CARTESIAN_POINT('Ctrl Pts',(0.225810271827769,-0.0725527034847115,
-1.03066527610617));
#79114=CARTESIAN_POINT('Ctrl Pts',(0.224832244951795,-0.0755326605728396,
-1.03087516842429));
#79115=CARTESIAN_POINT('Ctrl Pts',(0.224299569249094,-0.0771000919416258,
-1.03098649345032));
#79116=CARTESIAN_POINT('Ctrl Pts',(0.222821219024635,-0.0813052045236052,
-1.03128771683671));
#79117=CARTESIAN_POINT('Ctrl Pts',(0.221845162712163,-0.0839318446342196,
-1.03147860675645));
#79118=CARTESIAN_POINT('Ctrl Pts',(0.214978749279347,-0.101452672615652,
-1.03277094216049));
#79119=CARTESIAN_POINT('Ctrl Pts',(0.207640258122412,-0.115731820248825,
-1.03392154336467));
#79120=CARTESIAN_POINT('Ctrl Pts',(0.190866620668025,-0.141565051613736,
-1.0361673230617));
#79121=CARTESIAN_POINT('Ctrl Pts',(0.181668931873745,-0.153190075005969,
-1.03725418555946));
#79122=CARTESIAN_POINT('Ctrl Pts',(0.16993967111422,-0.165460723834768,
-1.03843942680745));
#79123=CARTESIAN_POINT('Ctrl Pts',(0.168409994050772,-0.167017417344487,
-1.03859052592468));
#79124=CARTESIAN_POINT('Ctrl Pts',(0.166112903541157,-0.16929142340211,
-1.03881205931299));
#79125=CARTESIAN_POINT('Ctrl Pts',(0.165361911283401,-0.17002506039485,
-1.03888365815618));
#79126=CARTESIAN_POINT('Ctrl Pts',(0.164008659216534,-0.171329591298828,
-1.03901116303144));
#79127=CARTESIAN_POINT('Ctrl Pts',(0.163408249876109,-0.171902335894749,
-1.03906720674767));
#79128=CARTESIAN_POINT('Ctrl Pts',(0.162063422706916,-0.173171784893965,
-1.03919156767787));
#79129=CARTESIAN_POINT('Ctrl Pts',(0.161317507197171,-0.173866851442591,
-1.03925976288274));
#79130=CARTESIAN_POINT('Ctrl Pts',(0.159075352176605,-0.175929307564545,
-1.03946251298447));
#79131=CARTESIAN_POINT('Ctrl Pts',(0.157565998515745,-0.177282389745873,
-1.03959605535742));
#79132=CARTESIAN_POINT('Ctrl Pts',(0.14680435203695,-0.18668379279955,-1.04052926957786));
#79133=CARTESIAN_POINT('Ctrl Pts',(0.13695621997452,-0.194024298481766,
-1.04128660916368));
#79134=CARTESIAN_POINT('Ctrl Pts',(0.111475754418332,-0.210105411199603,
-1.04313702348199));
#79135=CARTESIAN_POINT('Ctrl Pts',(0.0953411112426121,-0.217901638173178,
-1.04422336469095));
#79136=CARTESIAN_POINT('Ctrl Pts',(0.0756558190753961,-0.224804728092625,
-1.04556929784692));
#79137=CARTESIAN_POINT('Ctrl Pts',(0.0728082600008156,-0.22574305021203,
-1.04576430875033));
#79138=CARTESIAN_POINT('Ctrl Pts',(0.0681557743682794,-0.227178943837498,
-1.04608386395093));
#79139=CARTESIAN_POINT('Ctrl Pts',(0.0663613458199406,-0.227709581594742,
-1.04620733608837));
#79140=CARTESIAN_POINT('Ctrl Pts',(0.0631381880482992,-0.228621380954511,
-1.04642960536175));
#79141=CARTESIAN_POINT('Ctrl Pts',(0.0617118039432741,-0.229010523130603,
-1.04652813848353));
#79142=CARTESIAN_POINT('Ctrl Pts',(0.0586671946068927,-0.229810635622641,
-1.04673886187873));
#79143=CARTESIAN_POINT('Ctrl Pts',(0.0570480886870439,-0.230217903949045,
-1.04685116543061));
#79144=CARTESIAN_POINT('Ctrl Pts',(0.0526359396573457,-0.231278329753846,
-1.04715792139466));
#79145=CARTESIAN_POINT('Ctrl Pts',(0.0498352077782843,-0.231897949044186,
-1.04735342915494));
#79146=CARTESIAN_POINT('Ctrl Pts',(0.0435856875377352,-0.233162120464749,
-1.04779160436029));
#79147=CARTESIAN_POINT('Ctrl Pts',(0.0401324999153883,-0.233781237102707,
-1.0480350107266));
#79148=CARTESIAN_POINT('Ctrl Pts',(0.0290548992958242,-0.235514662775766,
-1.04882007640004));
#79149=CARTESIAN_POINT('Ctrl Pts',(0.0213899516262793,-0.236334073523972,
-1.04936984116713));
#79150=CARTESIAN_POINT('Ctrl Pts',(0.00478799391328773,-0.237294613084045,
-1.05057110856909));
#79151=CARTESIAN_POINT('Ctrl Pts',(-0.00414509168481391,-0.237306693014067,
-1.05122406692639));
#79152=CARTESIAN_POINT('Ctrl Pts',(-0.0242902853884312,-0.236195952007191,
-1.05269541458123));
#79153=CARTESIAN_POINT('Ctrl Pts',(-0.035466344310009,-0.234778066270788,
-1.05351101266602));
#79154=CARTESIAN_POINT('Ctrl Pts',(-0.0481873793934987,-0.232234614500244,
-1.05441163721122));
#79155=CARTESIAN_POINT('Ctrl Pts',(-0.0498705338404079,-0.231878998590682,
-1.05453021653198));
#79156=CARTESIAN_POINT('Ctrl Pts',(-0.0524930028081179,-0.231295047854816,
-1.05471390190666));
#79157=CARTESIAN_POINT('Ctrl Pts',(-0.0534350043918111,-0.231079239428459,
-1.05477966583622));
#79158=CARTESIAN_POINT('Ctrl Pts',(-0.0551070662549488,-0.230685405854194,
-1.05489598017823));
#79159=CARTESIAN_POINT('Ctrl Pts',(-0.0558376110229498,-0.230509666703362,
-1.05494665433323));
#79160=CARTESIAN_POINT('Ctrl Pts',(-0.0576079170433217,-0.230074893519484,
-1.05506911274893));
#79161=CARTESIAN_POINT('Ctrl Pts',(-0.058646774827929,-0.229812281322856,
-1.05514069337026));
#79162=CARTESIAN_POINT('Ctrl Pts',(-0.061907423111873,-0.228964473593114,
-1.05536458143485));
#79163=CARTESIAN_POINT('Ctrl Pts',(-0.0641225870506104,-0.228354010235895,
-1.05551553889758));
#79164=CARTESIAN_POINT('Ctrl Pts',(-0.0760387201802356,-0.224883034764211,
-1.05632314052172));
#79165=CARTESIAN_POINT('Ctrl Pts',(-0.0855591086550003,-0.221436111529642,
-1.05695258421108));
#79166=CARTESIAN_POINT('Ctrl Pts',(-0.112001080645514,-0.209901502775712,
-1.05872974198964));
#79167=CARTESIAN_POINT('Ctrl Pts',(-0.128221636485734,-0.2004046965426,
-1.0598610489778));
#79168=CARTESIAN_POINT('Ctrl Pts',(-0.146237878195228,-0.186765647193521,
-1.06131218136869));
#79169=CARTESIAN_POINT('Ctrl Pts',(-0.149262305835884,-0.184357493278386,
-1.06156297218875));
#79170=CARTESIAN_POINT('Ctrl Pts',(-0.153659624721604,-0.180677041837979,
-1.06193932951711));
#79171=CARTESIAN_POINT('Ctrl Pts',(-0.155078580404469,-0.179460600924075,
-1.06206265767154));
#79172=CARTESIAN_POINT('Ctrl Pts',(-0.157593859110736,-0.177252197603157,
-1.06228476957315));
#79173=CARTESIAN_POINT('Ctrl Pts',(-0.158695574409021,-0.176266504130917,
-1.06238329083007));
#79174=CARTESIAN_POINT('Ctrl Pts',(-0.160960147694014,-0.174201973018063,
-1.06258842426603));
#79175=CARTESIAN_POINT('Ctrl Pts',(-0.162121538277117,-0.173121642679709,
-1.06269509673446));
#79176=CARTESIAN_POINT('Ctrl Pts',(-0.165218586701251,-0.170182260488473,
-1.0629836062656));
#79177=CARTESIAN_POINT('Ctrl Pts',(-0.167133620764754,-0.168301916091612,
-1.06316635310828));
#79178=CARTESIAN_POINT('Ctrl Pts',(-0.171322343294662,-0.16404706792143,
-1.06357606163662));
#79179=CARTESIAN_POINT('Ctrl Pts',(-0.173579366219792,-0.161657006033895,
-1.06380368119495));
#79180=CARTESIAN_POINT('Ctrl Pts',(-0.180460826024781,-0.154059614458277,
-1.06451964334591));
#79181=CARTESIAN_POINT('Ctrl Pts',(-0.184905782807541,-0.148695363808847,
-1.06501457395697));
#79182=CARTESIAN_POINT('Ctrl Pts',(-0.194794536377068,-0.135631276239693,
-1.06619366010916));
#79183=CARTESIAN_POINT('Ctrl Pts',(-0.200028103684586,-0.127786919545031,
-1.06688210049181));
#79184=CARTESIAN_POINT('Ctrl Pts',(-0.210368095907426,-0.110090393717345,
-1.06837768425044));
#79185=CARTESIAN_POINT('Ctrl Pts',(-0.215279144308696,-0.100147728734526,
-1.06918280575839));
#79186=CARTESIAN_POINT('Ctrl Pts',(-0.220350216298021,-0.087767091446773,
-1.07011827124123));
#79187=CARTESIAN_POINT('Ctrl Pts',(-0.221191759099009,-0.0856241020359536,
-1.07027783831571));
#79188=CARTESIAN_POINT('Ctrl Pts',(-0.222379393101687,-0.0824653628230672,
-1.0705092639707));
#79189=CARTESIAN_POINT('Ctrl Pts',(-0.22274998036216,-0.0814590504621102,
-1.07058243601345));
#79190=CARTESIAN_POINT('Ctrl Pts',(-0.223395543726707,-0.0796687007431247,
-1.07071159105221));
#79191=CARTESIAN_POINT('Ctrl Pts',(-0.22367324072467,-0.0788856912771928,
-1.0707677279384));
#79192=CARTESIAN_POINT('Ctrl Pts',(-0.224276289152258,-0.0771565144426505,
-1.07089092803574));
#79193=CARTESIAN_POINT('Ctrl Pts',(-0.224599773585302,-0.0762097329305833,
-1.07095788333495));
#79194=CARTESIAN_POINT('Ctrl Pts',(-0.225530436687023,-0.0734284458676882,
-1.07115318645172));
#79195=CARTESIAN_POINT('Ctrl Pts',(-0.226121215753691,-0.0715884830683424,
-1.07128062923413));
#79196=CARTESIAN_POINT('Ctrl Pts',(-0.227434682839628,-0.0673191537280007,
-1.07157273294577));
#79197=CARTESIAN_POINT('Ctrl Pts',(-0.228141061333201,-0.0648849801559172,
-1.07173660435289));
#79198=CARTESIAN_POINT('Ctrl Pts',(-0.234346240336132,-0.0421463515096981,
-1.07324667502831));
#79199=CARTESIAN_POINT('Ctrl Pts',(-0.23716007325367,-0.0212056605925111,
-1.0744921961247));
#79200=CARTESIAN_POINT('Ctrl Pts',(-0.237174940775019,-0.000167610758756324,
-1.07580646542871));
#79201=CARTESIAN_POINT('Ctrl Pts',(-0.237174940975967,-0.000167326167951933,
-1.0758064832074));
#79202=CARTESIAN_POINT('Ctrl Pts',(-0.237178862066123,0.0053905870843023,
-1.07615369207584));
#79203=CARTESIAN_POINT('Ctrl Pts',(-0.236987418744219,0.0109466937660265,
-1.07650459862563));
#79204=CARTESIAN_POINT('Ctrl Pts',(-0.236357235544948,0.0199882338165463,
-1.07708571951255));
#79205=CARTESIAN_POINT('Ctrl Pts',(-0.236035958238224,0.0234797083819207,
-1.07731257753821));
#79206=CARTESIAN_POINT('Ctrl Pts',(-0.235451748788358,0.028585350679067,
-1.07764857627253));
#79207=CARTESIAN_POINT('Ctrl Pts',(-0.235249318460083,0.0302060627445365,
-1.07775586497137));
#79208=CARTESIAN_POINT('Ctrl Pts',(-0.234844445694626,0.0331961253736699,
-1.07795503732914));
#79209=CARTESIAN_POINT('Ctrl Pts',(-0.23464672248286,0.0345660513302701,
-1.07804677063649));
#79210=CARTESIAN_POINT('Ctrl Pts',(-0.234212791364183,0.0373970501584988,
-1.07823737613234));
#79211=CARTESIAN_POINT('Ctrl Pts',(-0.233974875812903,0.0388577960900436,
-1.07833629820839));
#79212=CARTESIAN_POINT('Ctrl Pts',(-0.233402731425097,0.0421746639260142,
-1.07856226748829));
#79213=CARTESIAN_POINT('Ctrl Pts',(-0.233060006585016,0.044029198130332,
-1.07868957783672));
#79214=CARTESIAN_POINT('Ctrl Pts',(-0.232105461240899,0.0488705456121785,
-1.07902454410932));
#79215=CARTESIAN_POINT('Ctrl Pts',(-0.231458118140091,0.0518499124122168,
-1.07923330578739));
#79216=CARTESIAN_POINT('Ctrl Pts',(-0.228201385953775,0.0655594948387103,
-1.08020646466981));
#79217=CARTESIAN_POINT('Ctrl Pts',(-0.224902383434084,0.0761102998773847,
-1.08099207286858));
#79218=CARTESIAN_POINT('Ctrl Pts',(-0.214898809544695,0.101686817098394,
-1.08297985397713));
#79219=CARTESIAN_POINT('Ctrl Pts',(-0.207344183031431,0.116318988124808,
-1.08419510814419));
#79220=CARTESIAN_POINT('Ctrl Pts',(-0.1968971818537,0.132251231487878,-1.08554657566402));
#79221=CARTESIAN_POINT('Ctrl Pts',(-0.19541948445007,0.134425127051742,
-1.08573154644371));
#79222=CARTESIAN_POINT('Ctrl Pts',(-0.192761715652386,0.138198587886219,
-1.08605304185617));
#79223=CARTESIAN_POINT('Ctrl Pts',(-0.191597122826209,0.139808697461259,
-1.08619036016341));
#79224=CARTESIAN_POINT('Ctrl Pts',(-0.189809300981019,0.142216149260442,
-1.08639566263785));
#79225=CARTESIAN_POINT('Ctrl Pts',(-0.189201012937958,0.143024405775023,
-1.08646458600006));
#79226=CARTESIAN_POINT('Ctrl Pts',(-0.188084165482272,0.144488810588983,
-1.08658941907345));
#79227=CARTESIAN_POINT('Ctrl Pts',(-0.187577320183138,0.145146197636944,
-1.08664543841547));
#79228=CARTESIAN_POINT('Ctrl Pts',(-0.186416063762288,0.146636124650379,
-1.08677236760309));
#79229=CARTESIAN_POINT('Ctrl Pts',(-0.185759518108305,0.147466957045006,
-1.08684312701278));
#79230=CARTESIAN_POINT('Ctrl Pts',(-0.183703075522032,0.150033775571511,
-1.08706176988591));
#79231=CARTESIAN_POINT('Ctrl Pts',(-0.182284197757902,0.151754492177387,
-1.0872083916332));
#79232=CARTESIAN_POINT('Ctrl Pts',(-0.171580297743114,0.164368652182197,
-1.08828581918711));
#79233=CARTESIAN_POINT('Ctrl Pts',(-0.161349171137063,0.174423068417167,
-1.08916025726684));
#79234=CARTESIAN_POINT('Ctrl Pts',(-0.137584934772982,0.193884761787855,
-1.09104387152952));
#79235=CARTESIAN_POINT('Ctrl Pts',(-0.123855728318893,0.202929999385158,
-1.09205099101611));
#79236=CARTESIAN_POINT('Ctrl Pts',(-0.106808676220347,0.211782423124832,
-1.09329659049535));
#79237=CARTESIAN_POINT('Ctrl Pts',(-0.104290327266397,0.213033834424817,
-1.09348036552311));
#79238=CARTESIAN_POINT('Ctrl Pts',(-0.100253109059542,0.214951255750261,
-1.09377492901638));
#79239=CARTESIAN_POINT('Ctrl Pts',(-0.0987484288401349,0.2156466456769,
-1.09388470170737));
#79240=CARTESIAN_POINT('Ctrl Pts',(-0.0958862203241227,0.216933181829503,
-1.09409355313709));
#79241=CARTESIAN_POINT('Ctrl Pts',(-0.0945301989032289,0.217527501597632,
-1.09419251744437));
#79242=CARTESIAN_POINT('Ctrl Pts',(-0.0914296588243891,0.218851946143835,
-1.09441888364329));
#79243=CARTESIAN_POINT('Ctrl Pts',(-0.0896818122788387,0.219573971660029,
-1.09454655218031));
#79244=CARTESIAN_POINT('Ctrl Pts',(-0.0850774328848414,0.2214118681141,
-1.09488311449045));
#79245=CARTESIAN_POINT('Ctrl Pts',(-0.0822076444581387,0.222493340570655,
-1.09509313129082));
#79246=CARTESIAN_POINT('Ctrl Pts',(-0.067140052852537,0.227840220495628,
-1.09619750318521));
#79247=CARTESIAN_POINT('Ctrl Pts',(-0.0546373980029665,0.231156380301354,
-1.09712135088387));
#79248=CARTESIAN_POINT('Ctrl Pts',(-0.0419358102824288,0.233438146927524,
-1.09805944304797));
#79249=CARTESIAN_POINT('Ctrl Pts',(-0.041935825738619,0.233438144150908,
-1.1176344235547));
#79250=CARTESIAN_POINT('Ctrl Pts',(-0.0432584147431629,0.23320054861047,
-1.11753987940428));
#79251=CARTESIAN_POINT('Ctrl Pts',(-0.0445790138342224,0.232951707726502,
-1.11744577078433));
#79252=CARTESIAN_POINT('Ctrl Pts',(-0.0478545145984987,0.232305628549752,
-1.11721319422148));
#79253=CARTESIAN_POINT('Ctrl Pts',(-0.0498066840877963,0.231894921239782,
-1.11707532872025));
#79254=CARTESIAN_POINT('Ctrl Pts',(-0.0527420365903041,0.23123858723122,
-1.11686939068683));
#79255=CARTESIAN_POINT('Ctrl Pts',(-0.0537291523560751,0.231011222520726,
-1.11680037029715));
#79256=CARTESIAN_POINT('Ctrl Pts',(-0.0555221924243775,0.230586112531759,
-1.11667546141249));
#79257=CARTESIAN_POINT('Ctrl Pts',(-0.0563285566144401,0.230390457483617,
-1.11661946209737));
#79258=CARTESIAN_POINT('Ctrl Pts',(-0.0581593880948962,0.229936040176821,
-1.11649270523686));
#79259=CARTESIAN_POINT('Ctrl Pts',(-0.0591831699277879,0.229674660115662,
-1.11642209661691));
#79260=CARTESIAN_POINT('Ctrl Pts',(-0.0623513108756212,0.228843216399275,
-1.11620434306506));
#79261=CARTESIAN_POINT('Ctrl Pts',(-0.0644895124102746,0.228249879115558,
-1.11605844550895));
#79262=CARTESIAN_POINT('Ctrl Pts',(-0.0804411449225277,0.223581336608984,
-1.11497583139735));
#79263=CARTESIAN_POINT('Ctrl Pts',(-0.0938678722178763,0.218284964487372,
-1.11409628320732));
#79264=CARTESIAN_POINT('Ctrl Pts',(-0.121225158260334,0.204498946064232,
-1.11221768093849));
#79265=CARTESIAN_POINT('Ctrl Pts',(-0.134928190839646,0.195728522223323,
-1.111220778427));
#79266=CARTESIAN_POINT('Ctrl Pts',(-0.149870746536511,0.183844912791191,
-1.10998343070978));
#79267=CARTESIAN_POINT('Ctrl Pts',(-0.152081003720497,0.18202076745062,
-1.10979622974101));
#79268=CARTESIAN_POINT('Ctrl Pts',(-0.155525100972375,0.179071795722006,
-1.10949748089988));
#79269=CARTESIAN_POINT('Ctrl Pts',(-0.156781091943716,0.177973183444333,
-1.10938700094757));
#79270=CARTESIAN_POINT('Ctrl Pts',(-0.159127602488053,0.175876580659945,
-1.10917761533894));
#79271=CARTESIAN_POINT('Ctrl Pts',(-0.160220592650936,0.174881465624513,
-1.10907883277091));
#79272=CARTESIAN_POINT('Ctrl Pts',(-0.162676037205598,0.172603560706968,
-1.10885400800687));
#79273=CARTESIAN_POINT('Ctrl Pts',(-0.164032740614149,0.171314745156312,
-1.10872771235579));
#79274=CARTESIAN_POINT('Ctrl Pts',(-0.167523835053847,0.167918849777242,
-1.10839718727363));
#79275=CARTESIAN_POINT('Ctrl Pts',(-0.169633702827952,0.165787155296867,
-1.10819189907962));
#79276=CARTESIAN_POINT('Ctrl Pts',(-0.18633269399496,0.14826285050924,-1.10652098070454));
#79277=CARTESIAN_POINT('Ctrl Pts',(-0.198835186131925,0.131018926427349,
-1.10496576128198));
#79278=CARTESIAN_POINT('Ctrl Pts',(-0.211936469554454,0.106661251859097,
-1.10295434041515));
#79279=CARTESIAN_POINT('Ctrl Pts',(-0.21476233504746,0.100850581086543,
-1.10248776970752));
#79280=CARTESIAN_POINT('Ctrl Pts',(-0.218866844715034,0.0914532183775448,
-1.10176075598685));
#79281=CARTESIAN_POINT('Ctrl Pts',(-0.220302443603446,0.0879387522343233,
-1.10149476703641));
#79282=CARTESIAN_POINT('Ctrl Pts',(-0.222115461967171,0.0831768616275617,
-1.1011435827967));
#79283=CARTESIAN_POINT('Ctrl Pts',(-0.222567797019122,0.0819587986620246,
-1.10105454939646));
#79284=CARTESIAN_POINT('Ctrl Pts',(-0.223304577744365,0.079923678961788,
-1.10090718962121));
#79285=CARTESIAN_POINT('Ctrl Pts',(-0.223594599298818,0.079108685664839,
-1.10084854765242));
#79286=CARTESIAN_POINT('Ctrl Pts',(-0.224175104256493,0.0774487028060394,
-1.10072988227105));
#79287=CARTESIAN_POINT('Ctrl Pts',(-0.22446528291949,0.0766036276237135,
-1.10066987634708));
#79288=CARTESIAN_POINT('Ctrl Pts',(-0.22520818891043,0.074399622486152,
-1.10051438000326));
#79289=CARTESIAN_POINT('Ctrl Pts',(-0.22565340218859,0.0730381715987563,
-1.10041931512584));
#79290=CARTESIAN_POINT('Ctrl Pts',(-0.227469110746063,0.0673106546749251,
-1.10002318580741));
#79291=CARTESIAN_POINT('Ctrl Pts',(-0.228725529703862,0.0629091332568091,
-1.09972798206613));
#79292=CARTESIAN_POINT('Ctrl Pts',(-0.234701318000397,0.0394189412878362,
-1.09818747149911));
#79293=CARTESIAN_POINT('Ctrl Pts',(-0.237160909058553,0.0198342418859032,
-1.09701798258436));
#79294=CARTESIAN_POINT('Ctrl Pts',(-0.237180895959023,-0.00817906410562867,
-1.09526945720993));
#79295=CARTESIAN_POINT('Ctrl Pts',(-0.23674608175383,-0.0165210456300815,
-1.09474017428215));
#79296=CARTESIAN_POINT('Ctrl Pts',(-0.235605684004054,-0.0273576742908374,
-1.09403156010411));
#79297=CARTESIAN_POINT('Ctrl Pts',(-0.235298000269286,-0.0298886421000947,
-1.09386457201332));
#79298=CARTESIAN_POINT('Ctrl Pts',(-0.234730728404759,-0.0340004443507289,
-1.09359062134863));
#79299=CARTESIAN_POINT('Ctrl Pts',(-0.234495814488319,-0.0355845169790469,
-1.09348443583019));
#79300=CARTESIAN_POINT('Ctrl Pts',(-0.234010490452502,-0.0386433475482477,
-1.09327808426633));
#79301=CARTESIAN_POINT('Ctrl Pts',(-0.233762133698072,-0.0401183576945601,
-1.09317798762596));
#79302=CARTESIAN_POINT('Ctrl Pts',(-0.233147763302373,-0.0435675598671642,
-1.09294248566356));
#79303=CARTESIAN_POINT('Ctrl Pts',(-0.232770604039708,-0.0455396230792217,
-1.09280673365433));
#79304=CARTESIAN_POINT('Ctrl Pts',(-0.231434182177033,-0.052076446103443,
-1.09235295129829));
#79305=CARTESIAN_POINT('Ctrl Pts',(-0.230365358728379,-0.0566174277673322,
-1.09203149976684));
#79306=CARTESIAN_POINT('Ctrl Pts',(-0.227436181018103,-0.0675994291027317,
-1.09123837718875));
#79307=CARTESIAN_POINT('Ctrl Pts',(-0.225435366848108,-0.0739985218730699,
-1.09076274281024));
#79308=CARTESIAN_POINT('Ctrl Pts',(-0.219886246610391,-0.0894196673008559,
-1.08958509792107));
#79309=CARTESIAN_POINT('Ctrl Pts',(-0.216050722666752,-0.0983255080361264,
-1.08887747868718));
#79310=CARTESIAN_POINT('Ctrl Pts',(-0.211077489394449,-0.108166853959196,
-1.08807278828868));
#79311=CARTESIAN_POINT('Ctrl Pts',(-0.210463235784185,-0.109357218463305,
-1.08797507328014));
#79312=CARTESIAN_POINT('Ctrl Pts',(-0.204794420627367,-0.120118147979523,
-1.08708851419382));
#79313=CARTESIAN_POINT('Ctrl Pts',(-0.199099755496709,-0.129338562640794,
-1.08630504860256));
#79314=CARTESIAN_POINT('Ctrl Pts',(-0.191794456136614,-0.13953428040076,
-1.08543432176941));
#79315=CARTESIAN_POINT('Ctrl Pts',(-0.190779238413752,-0.140919166289695,
-1.08531596517228));
#79316=CARTESIAN_POINT('Ctrl Pts',(-0.189169783698143,-0.143065389767239,
-1.08513256053827));
#79317=CARTESIAN_POINT('Ctrl Pts',(-0.188585808980038,-0.143834298927607,
-1.08506685749316));
#79318=CARTESIAN_POINT('Ctrl Pts',(-0.187539111361058,-0.145195133329188,
-1.08495061294781));
#79319=CARTESIAN_POINT('Ctrl Pts',(-0.18707826474446,-0.145788435466187,
-1.08489994822086));
#79320=CARTESIAN_POINT('Ctrl Pts',(-0.185952965723256,-0.147223042905706,
-1.08477746600266));
#79321=CARTESIAN_POINT('Ctrl Pts',(-0.185285618023984,-0.148062046749886,
-1.08470585259045));
#79322=CARTESIAN_POINT('Ctrl Pts',(-0.183167875745051,-0.150687775624103,
-1.08448168594729));
#79323=CARTESIAN_POINT('Ctrl Pts',(-0.181697103286738,-0.15245799436519,
-1.08433048781053));
#79324=CARTESIAN_POINT('Ctrl Pts',(-0.173599167340606,-0.16192097419043,
-1.08352009172825));
#79325=CARTESIAN_POINT('Ctrl Pts',(-0.166508250020531,-0.169204379850674,
-1.0828883038835));
#79326=CARTESIAN_POINT('Ctrl Pts',(-0.14496027030146,-0.188666264735665,
-1.08109977920796));
#79327=CARTESIAN_POINT('Ctrl Pts',(-0.129489536818853,-0.199601713344846,
-1.07995946483688));
#79328=CARTESIAN_POINT('Ctrl Pts',(-0.109595528023059,-0.210368255174794,
-1.07850528921785));
#79329=CARTESIAN_POINT('Ctrl Pts',(-0.106263112035296,-0.212071051985996,
-1.07826233900726));
#79330=CARTESIAN_POINT('Ctrl Pts',(-0.101229227633994,-0.214494824395458,
-1.07789550127565));
#79331=CARTESIAN_POINT('Ctrl Pts',(-0.0995572560229314,-0.215275959346244,
-1.07777368633027));
#79332=CARTESIAN_POINT('Ctrl Pts',(-0.0965320681297575,-0.216646529050584,
-1.07755324147311));
#79333=CARTESIAN_POINT('Ctrl Pts',(-0.0951821297104626,-0.21724299929477,
-1.07745485826849));
#79334=CARTESIAN_POINT('Ctrl Pts',(-0.0922786719891962,-0.218493634851812,
-1.07724318150654));
#79335=CARTESIAN_POINT('Ctrl Pts',(-0.0907235770867759,-0.21914391180543,
-1.07712976255671));
#79336=CARTESIAN_POINT('Ctrl Pts',(-0.0864320615048512,-0.220884939992683,
-1.07681657502509));
#79337=CARTESIAN_POINT('Ctrl Pts',(-0.0836821241165773,-0.221941340717135,
-1.07661567436842));
#79338=CARTESIAN_POINT('Ctrl Pts',(-0.0661468319828223,-0.228305381865129,
-1.07533270991089));
#79339=CARTESIAN_POINT('Ctrl Pts',(-0.0508870687365766,-0.232183315238453,
-1.07420388970789));
#79340=CARTESIAN_POINT('Ctrl Pts',(-0.0206860742155622,-0.236736673614914,
-1.07197708491382));
#79341=CARTESIAN_POINT('Ctrl Pts',(-0.00583693106709541,-0.237567181760435,
-1.07088651934837));
#79342=CARTESIAN_POINT('Ctrl Pts',(0.0111713767472046,-0.236921783383169,
-1.06969812353675));
#79343=CARTESIAN_POINT('Ctrl Pts',(0.0133482226765466,-0.236809114880699,
-1.06954721637732));
#79344=CARTESIAN_POINT('Ctrl Pts',(0.0165701763129834,-0.236597782211589,
-1.06932592038241));
#79345=CARTESIAN_POINT('Ctrl Pts',(0.0176166108213919,-0.236522168979225,
-1.06925437013267));
#79346=CARTESIAN_POINT('Ctrl Pts',(0.0194894788098894,-0.236374340695349,
-1.06912693138538));
#79347=CARTESIAN_POINT('Ctrl Pts',(0.0203160699731221,-0.236304731406512,
-1.06907090556273));
#79348=CARTESIAN_POINT('Ctrl Pts',(0.022157803791001,-0.236139898833785,
-1.06894656186513));
#79349=CARTESIAN_POINT('Ctrl Pts',(0.0231727133625775,-0.236042465547013,
-1.06887836616163));
#79350=CARTESIAN_POINT('Ctrl Pts',(0.0262042667836905,-0.235731689030862,
-1.06867555262856));
#79351=CARTESIAN_POINT('Ctrl Pts',(0.0282188947616265,-0.235499017964752,
-1.06854194855638));
#79352=CARTESIAN_POINT('Ctrl Pts',(0.0425162286639773,-0.233661691164076,
-1.06760057908901));
#79353=CARTESIAN_POINT('Ctrl Pts',(0.0546612103196223,-0.231122582108777,
-1.066836022966));
#79354=CARTESIAN_POINT('Ctrl Pts',(0.0835576052644631,-0.222674558692563,
-1.06498741405034));
#79355=CARTESIAN_POINT('Ctrl Pts',(0.0999492663670512,-0.215814504679519,
-1.06390955869622));
#79356=CARTESIAN_POINT('Ctrl Pts',(0.118053699579086,-0.205728868638331,
-1.06257259555048));
#79357=CARTESIAN_POINT('Ctrl Pts',(0.120655360564963,-0.204213922242535,
-1.06237679568973));
#79358=CARTESIAN_POINT('Ctrl Pts',(0.124829066146606,-0.201675974774374,
-1.06205622661396));
#79359=CARTESIAN_POINT('Ctrl Pts',(0.126419097810772,-0.200683098265499,
-1.0619325415429));
#79360=CARTESIAN_POINT('Ctrl Pts',(0.129241827575505,-0.198873619299367,
-1.0617100648972));
#79361=CARTESIAN_POINT('Ctrl Pts',(0.130478986493682,-0.19806413194422,
-1.06161153981394));
#79362=CARTESIAN_POINT('Ctrl Pts',(0.133094500257903,-0.196317631088904,
-1.06140102372933));
#79363=CARTESIAN_POINT('Ctrl Pts',(0.134470702127523,-0.195377553211979,
-1.06128892131451));
#79364=CARTESIAN_POINT('Ctrl Pts',(0.138178099611331,-0.192787319425447,
-1.06098320895841));
#79365=CARTESIAN_POINT('Ctrl Pts',(0.140489515939453,-0.191109477573222,
-1.06078855538736));
#79366=CARTESIAN_POINT('Ctrl Pts',(0.145556013586486,-0.187290150293546,
-1.06035258462282));
#79367=CARTESIAN_POINT('Ctrl Pts',(0.148295226981576,-0.185128811831091,
-1.06011053968791));
#79368=CARTESIAN_POINT('Ctrl Pts',(0.156877657019354,-0.178044243243746,
-1.05933149275798));
#79369=CARTESIAN_POINT('Ctrl Pts',(0.162530690091508,-0.17289912606251,
-1.05878652292557));
#79370=CARTESIAN_POINT('Ctrl Pts',(0.173864174519878,-0.161536236966017,
-1.05762757763605));
#79371=CARTESIAN_POINT('Ctrl Pts',(0.179482076943847,-0.155270351159474,
-1.05701294170188));
#79372=CARTESIAN_POINT('Ctrl Pts',(0.191634048293048,-0.140173895407708,
-1.05559890707435));
#79373=CARTESIAN_POINT('Ctrl Pts',(0.197912449813362,-0.131160351655729,
-1.05480164848869));
#79374=CARTESIAN_POINT('Ctrl Pts',(0.204725113886799,-0.119770182574942,
-1.05387368016769));
#79375=CARTESIAN_POINT('Ctrl Pts',(0.205876817717127,-0.117779479506916,
-1.05371428644884));
#79376=CARTESIAN_POINT('Ctrl Pts',(0.207522567309833,-0.114836898388701,
-1.05348307539116));
#79377=CARTESIAN_POINT('Ctrl Pts',(0.20803936526954,-0.113897988499236,
-1.05340994758363));
#79378=CARTESIAN_POINT('Ctrl Pts',(0.208945332949383,-0.112225301201956,
-1.05328085484548));
#79379=CARTESIAN_POINT('Ctrl Pts',(0.209337033802809,-0.111492944795534,
-1.05322473634107));
#79380=CARTESIAN_POINT('Ctrl Pts',(0.210192080126655,-0.109873886307508,
-1.0531015600062));
#79381=CARTESIAN_POINT('Ctrl Pts',(0.210653670030632,-0.108986296542092,
-1.05303461019088));
#79382=CARTESIAN_POINT('Ctrl Pts',(0.21199054352247,-0.106375400452049,
-1.05283928139431));
#79383=CARTESIAN_POINT('Ctrl Pts',(0.212850418549568,-0.104644236702914,
-1.05271180808617));
#79384=CARTESIAN_POINT('Ctrl Pts',(0.214789057711334,-0.100618433236373,
-1.05241961094872));
#79385=CARTESIAN_POINT('Ctrl Pts',(0.215852397946036,-0.0983165897528305,
-1.05225567752442));
#79386=CARTESIAN_POINT('Ctrl Pts',(0.2194210200343,-0.0902543627498628,
-1.05169082208325));
#79387=CARTESIAN_POINT('Ctrl Pts',(0.221734378838158,-0.0844115511749129,
-1.05129776320076));
#79388=CARTESIAN_POINT('Ctrl Pts',(0.230975722706703,-0.058057775409552,
-1.04956810329019));
#79389=CARTESIAN_POINT('Ctrl Pts',(0.235308154437333,-0.0367496063000072,
-1.04827267502526));
#79390=CARTESIAN_POINT('Ctrl Pts',(0.236876294148964,-0.01224935120234,
-1.04668717273614));
#79391=CARTESIAN_POINT('Ctrl Pts',(0.237008590165596,-0.0093462475537947,
-1.04649800961096));
#79392=CARTESIAN_POINT('Ctrl Pts',(0.237137592671283,-0.00459818055543863,
-1.04618613342297));
#79393=CARTESIAN_POINT('Ctrl Pts',(0.237166174676999,-0.0027543404976851,
-1.0460644071904));
#79394=CARTESIAN_POINT('Ctrl Pts',(0.237178917304436,0.000565321360051544,
-1.04584405775318));
#79395=CARTESIAN_POINT('Ctrl Pts',(0.237170808543679,0.00204103122160897,
-1.04574568031712));
#79396=CARTESIAN_POINT('Ctrl Pts',(0.237123923356802,0.00520288001015451,
-1.04553394380727));
#79397=CARTESIAN_POINT('Ctrl Pts',(0.237080931901491,0.00688886512915874,
-1.04542045864654));
#79398=CARTESIAN_POINT('Ctrl Pts',(0.236913308281436,0.0115225442702795,
-1.04510689388477));
#79399=CARTESIAN_POINT('Ctrl Pts',(0.236751653754406,0.0144685089101486,
-1.04490567766309));
#79400=CARTESIAN_POINT('Ctrl Pts',(0.235372694165352,0.0332026542227912,
-1.04361368612197));
#79401=CARTESIAN_POINT('Ctrl Pts',(0.232631933987971,0.0488358064434803,
-1.04247534349324));
#79402=CARTESIAN_POINT('Ctrl Pts',(0.2243863945295,0.078221135425702,-1.04024984078445));
#79403=CARTESIAN_POINT('Ctrl Pts',(0.21911155581906,0.0919673583819196,
-1.03917057086671));
#79404=CARTESIAN_POINT('Ctrl Pts',(0.211628035709293,0.107099695578416,
-1.03799174648102));
#79405=CARTESIAN_POINT('Ctrl Pts',(0.210630725807367,0.109048010005371,
-1.03784020551841));
#79406=CARTESIAN_POINT('Ctrl Pts',(0.209114822937106,0.111911016950864,
-1.03761816690457));
#79407=CARTESIAN_POINT('Ctrl Pts',(0.208616920979453,0.112836453655353,
-1.03754649698122));
#79408=CARTESIAN_POINT('Ctrl Pts',(0.207714980146303,0.11448648752969,-1.0374189345759));
#79409=CARTESIAN_POINT('Ctrl Pts',(0.207313273852756,0.115212305549409,
-1.03736290352999));
#79410=CARTESIAN_POINT('Ctrl Pts',(0.206410129580288,0.116824121426516,
-1.03723865641094));
#79411=CARTESIAN_POINT('Ctrl Pts',(0.205906788185745,0.117709012463264,
-1.03717056137602));
#79412=CARTESIAN_POINT('Ctrl Pts',(0.204387682084271,0.120340088063792,
-1.03696835805898));
#79413=CARTESIAN_POINT('Ctrl Pts',(0.203355260157899,0.122076616166908,
-1.03683525450085));
#79414=CARTESIAN_POINT('Ctrl Pts',(0.19622874852658,0.133722017962486,-1.0359435488359));
#79415=CARTESIAN_POINT('Ctrl Pts',(0.189434191489689,0.143185389677278,
-1.03522296781266));
#79416=CARTESIAN_POINT('Ctrl Pts',(0.170008526071012,0.166424199934096,
-1.03336109604057));
#79417=CARTESIAN_POINT('Ctrl Pts',(0.156400355804899,0.179272882566176,
-1.03222990967809));
#79418=CARTESIAN_POINT('Ctrl Pts',(0.139084193357974,0.192135612061835,
-1.03083703494809));
#79419=CARTESIAN_POINT('Ctrl Pts',(0.136708374297954,0.193833241385375,
-1.03064698887796));
#79420=CARTESIAN_POINT('Ctrl Pts',(0.132778626281439,0.196533031779483,
-1.03033395521202));
#79421=CARTESIAN_POINT('Ctrl Pts',(0.131243208204679,0.197561676840038,
-1.03021196715654));
#79422=CARTESIAN_POINT('Ctrl Pts',(0.128460147090678,0.1993794121323,-1.02999133583768));
#79423=CARTESIAN_POINT('Ctrl Pts',(0.127216849449188,0.200175004485255,
-1.02989294111283));
#79424=CARTESIAN_POINT('Ctrl Pts',(0.124539605077382,0.201853170216394,
-1.02968137965615));
#79425=CARTESIAN_POINT('Ctrl Pts',(0.123103530718277,0.202732178084126,
-1.0295680888783));
#79426=CARTESIAN_POINT('Ctrl Pts',(0.11913709296571,0.205102314762505,-1.02925563121948));
#79427=CARTESIAN_POINT('Ctrl Pts',(0.11658827321648,0.206561805874336,-1.02905534103617));
#79428=CARTESIAN_POINT('Ctrl Pts',(0.100446991949007,0.215410612474166,
-1.0277894580985));
#79429=CARTESIAN_POINT('Ctrl Pts',(0.0861881651912132,0.221501177972588,
-1.02667862028116));
#79430=CARTESIAN_POINT('Ctrl Pts',(0.0570305285888865,0.230711662890633,
-1.02444985760861));
#79431=CARTESIAN_POINT('Ctrl Pts',(0.042217314780757,0.233876293929315,
-1.02333837641646));
#79432=CARTESIAN_POINT('Ctrl Pts',(0.0250501503004153,0.23585836026058,
-1.0221319627321));
#79433=CARTESIAN_POINT('Ctrl Pts',(0.0228941366896339,0.236077392957802,
-1.02198194878531));
#79434=CARTESIAN_POINT('Ctrl Pts',(0.0196926342274622,0.236358364298436,
-1.02176169994375));
#79435=CARTESIAN_POINT('Ctrl Pts',(0.018649317604025,0.236442972561779,
-1.02169031886137));
#79436=CARTESIAN_POINT('Ctrl Pts',(0.0167782821581367,0.236582243355564,
-1.02156305436527));
#79437=CARTESIAN_POINT('Ctrl Pts',(0.0159508028836025,0.236639473821558,
-1.02150703537961));
#79438=CARTESIAN_POINT('Ctrl Pts',(0.0141033221573189,0.23675751500798,
-1.0213825527393));
#79439=CARTESIAN_POINT('Ctrl Pts',(0.0130832122459482,0.236816076866771,
-1.02131421287601));
#79440=CARTESIAN_POINT('Ctrl Pts',(0.0100263736711766,0.236971749300597,
-1.02111052376976));
#79441=CARTESIAN_POINT('Ctrl Pts',(0.00798867851495863,0.237049192857883,
-1.02097620131491));
#79442=CARTESIAN_POINT('Ctrl Pts',(-0.00751269379989495,0.237438207772837,
-1.01996371900727));
#79443=CARTESIAN_POINT('Ctrl Pts',(-0.0209817699170307,0.236628836981253,
-1.01913673223224));
#79444=CARTESIAN_POINT('Ctrl Pts',(-0.0368600042990974,0.234307400803627,
-1.0181523677623));
#79445=CARTESIAN_POINT('Ctrl Pts',(-0.0394020145324293,0.233893328965883,
-1.01799451955588));
#79446=CARTESIAN_POINT('Ctrl Pts',(-0.0419358384531398,0.233438141866817,
-1.01783655831731));
#79447=CARTESIAN_POINT('Origin',(0.,0.,-1.7456589891905));
#79448=CARTESIAN_POINT('',(-0.0419358085112891,0.233438147245699,-0.898263402204347));
#79449=CARTESIAN_POINT('',(-0.0419358257166344,0.233438144154858,-0.917832673049623));
#79450=CARTESIAN_POINT('',(-0.0419358257166344,0.233438144154858,-1.7456589891905));
#79451=CARTESIAN_POINT('Ctrl Pts',(-0.0419358085112876,0.233438147245699,
-0.898263402204347));
#79452=CARTESIAN_POINT('Ctrl Pts',(-0.0319888766060671,0.235225055840433,
-0.898895225798914));
#79453=CARTESIAN_POINT('Ctrl Pts',(-0.0219318578014211,0.236375459711886,
-0.899511712826814));
#79454=CARTESIAN_POINT('Ctrl Pts',(0.00272931081665239,0.237606640110077,
-0.901027390268067));
#79455=CARTESIAN_POINT('Ctrl Pts',(0.0173186563714538,0.236990193389189,
-0.901929115462318));
#79456=CARTESIAN_POINT('Ctrl Pts',(0.0345123267016579,0.234667005850247,
-0.903054578955355));
#79457=CARTESIAN_POINT('Ctrl Pts',(0.0372596020371669,0.234246505485218,
-0.903236254471884));
#79458=CARTESIAN_POINT('Ctrl Pts',(0.0416257230043633,0.233499473865356,
-0.903528240560429));
#79459=CARTESIAN_POINT('Ctrl Pts',(0.0432496965276298,0.23320413510385,
-0.903637566652367));
#79460=CARTESIAN_POINT('Ctrl Pts',(0.046325568956889,0.232611518075377,
-0.903846070506072));
#79461=CARTESIAN_POINT('Ctrl Pts',(0.0477780279958681,0.232317533884336,
-0.903945139189474));
#79462=CARTESIAN_POINT('Ctrl Pts',(0.0510895793313697,0.231614892706939,
-0.904172455702432));
#79463=CARTESIAN_POINT('Ctrl Pts',(0.0529466776716615,0.231197432072285,
-0.904300978534616));
#79464=CARTESIAN_POINT('Ctrl Pts',(0.057823902761613,0.230039227300763,
-0.904641358884654));
#79465=CARTESIAN_POINT('Ctrl Pts',(0.0608347485656282,0.229261382723428,
-0.904854381261831));
#79466=CARTESIAN_POINT('Ctrl Pts',(0.0823465451792399,0.223250282427531,
-0.906397872384761));
#79467=CARTESIAN_POINT('Ctrl Pts',(0.100162873238279,0.215844320331424,
-0.907799880074513));
#79468=CARTESIAN_POINT('Ctrl Pts',(0.125812924226704,0.201316504406839,
-0.909949487679603));
#79469=CARTESIAN_POINT('Ctrl Pts',(0.134402978183474,0.1956862460259,-0.910693401308479));
#79470=CARTESIAN_POINT('Ctrl Pts',(0.144449562121192,0.18812668697498,-0.911572616295714));
#79471=CARTESIAN_POINT('Ctrl Pts',(0.146276713074969,0.186709535248029,
-0.911732891397154));
#79472=CARTESIAN_POINT('Ctrl Pts',(0.148922018199757,0.184595143502008,
-0.911965141409346));
#79473=CARTESIAN_POINT('Ctrl Pts',(0.149756560701523,0.183918751486441,
-0.912038442588177));
#79474=CARTESIAN_POINT('Ctrl Pts',(0.151167242551874,0.18275943326571,-0.912162359577785));
#79475=CARTESIAN_POINT('Ctrl Pts',(0.151745718614855,0.182279408077655,
-0.912213175675524));
#79476=CARTESIAN_POINT('Ctrl Pts',(0.15306127146946,0.181177145847669,-0.912328737402071));
#79477=CARTESIAN_POINT('Ctrl Pts',(0.153796845382576,0.180553154040393,
-0.912393355066334));
#79478=CARTESIAN_POINT('Ctrl Pts',(0.155827416314408,0.178809194829818,
-0.912571808566162));
#79479=CARTESIAN_POINT('Ctrl Pts',(0.157114154114831,0.177679640993131,
-0.912684976811264));
#79480=CARTESIAN_POINT('Ctrl Pts',(0.165813577980176,0.169874502992107,
-0.913451594860854));
#79481=CARTESIAN_POINT('Ctrl Pts',(0.172811851616639,0.162750123594717,
-0.91407606452951));
#79482=CARTESIAN_POINT('Ctrl Pts',(0.180882076414711,0.153424896482839,
-0.914837880136115));
#79483=CARTESIAN_POINT('Ctrl Pts',(0.182396277977555,0.15162164235704,-0.914982818756633));
#79484=CARTESIAN_POINT('Ctrl Pts',(0.188940325026111,0.143588446716834,
-0.915619517746367));
#79485=CARTESIAN_POINT('Ctrl Pts',(0.19367961999078,0.137128741727366,-0.916108381332049));
#79486=CARTESIAN_POINT('Ctrl Pts',(0.202270450707712,0.124083085174235,
-0.917072996734549));
#79487=CARTESIAN_POINT('Ctrl Pts',(0.206148895609117,0.117526878646687,
-0.917547635043089));
#79488=CARTESIAN_POINT('Ctrl Pts',(0.211331547029984,0.107717587695387,
-0.918253493502797));
#79489=CARTESIAN_POINT('Ctrl Pts',(0.21288988123294,0.104604006103212,-0.918476909430575));
#79490=CARTESIAN_POINT('Ctrl Pts',(0.215598850286897,0.0988799639369577,
-0.918887393180001));
#79491=CARTESIAN_POINT('Ctrl Pts',(0.216772011600246,0.0962808670801677,
-0.919073688260315));
#79492=CARTESIAN_POINT('Ctrl Pts',(0.218555885205595,0.092130782567806,
-0.919371345368958));
#79493=CARTESIAN_POINT('Ctrl Pts',(0.219197620987187,0.0905933704529978,
-0.91948165351673));
#79494=CARTESIAN_POINT('Ctrl Pts',(0.220378426406352,0.0876784892344844,
-0.91969093397954));
#79495=CARTESIAN_POINT('Ctrl Pts',(0.220920912300254,0.086302483382735,
-0.919789785527184));
#79496=CARTESIAN_POINT('Ctrl Pts',(0.222122553961468,0.0831689534384998,
-0.920015073220043));
#79497=CARTESIAN_POINT('Ctrl Pts',(0.222773779863433,0.0814085158215507,
-0.920141766482311));
#79498=CARTESIAN_POINT('Ctrl Pts',(0.224417420068755,0.0767978531035248,
-0.920473989617902));
#79499=CARTESIAN_POINT('Ctrl Pts',(0.225376420084786,0.0739361649639672,
-0.920680595850073));
#79500=CARTESIAN_POINT('Ctrl Pts',(0.232607012340755,0.0509104165485765,
-0.922346846383017));
#79501=CARTESIAN_POINT('Ctrl Pts',(0.236213491604805,0.0300121412479962,
-0.923895134425683));
#79502=CARTESIAN_POINT('Ctrl Pts',(0.237251504713968,0.00242790597118925,
-0.925902865784434));
#79503=CARTESIAN_POINT('Ctrl Pts',(0.23722902780818,-0.0040706487750538,
-0.92637220302656));
#79504=CARTESIAN_POINT('Ctrl Pts',(0.236770127078069,-0.014366785062582,
-0.927102966723891));
#79505=CARTESIAN_POINT('Ctrl Pts',(0.236508769790435,-0.0181687472925312,
-0.927370000774217));
#79506=CARTESIAN_POINT('Ctrl Pts',(0.23603539020919,-0.0232587319903634,
-0.927722341845574));
#79507=CARTESIAN_POINT('Ctrl Pts',(0.235904219791878,-0.0245534788415448,
-0.927811517314698));
#79508=CARTESIAN_POINT('Ctrl Pts',(0.235668061219351,-0.0267075802354654,
-0.927959058867024));
#79509=CARTESIAN_POINT('Ctrl Pts',(0.235569014407845,-0.0275675434954728,
-0.92801774192755));
#79510=CARTESIAN_POINT('Ctrl Pts',(0.235358188720312,-0.0293138472968358,
-0.928136437930932));
#79511=CARTESIAN_POINT('Ctrl Pts',(0.235246106804209,-0.0302001314727833,
-0.928196433825474));
#79512=CARTESIAN_POINT('Ctrl Pts',(0.234941487447494,-0.0325042348595186,
-0.928351819804342));
#79513=CARTESIAN_POINT('Ctrl Pts',(0.234741119756891,-0.0339210075579321,
-0.928446785683628));
#79514=CARTESIAN_POINT('Ctrl Pts',(0.233848577443344,-0.039844897126972,
-0.928841761282919));
#79515=CARTESIAN_POINT('Ctrl Pts',(0.233039273817071,-0.0443336915432166,
-0.929135953584295));
#79516=CARTESIAN_POINT('Ctrl Pts',(0.229251243090949,-0.0623514239198177,
-0.930306285253463));
#79517=CARTESIAN_POINT('Ctrl Pts',(0.225219367307328,-0.0756315542121117,
-0.931145925736226));
#79518=CARTESIAN_POINT('Ctrl Pts',(0.215742212030513,-0.0992001264668327,
-0.932706840439582));
#79519=CARTESIAN_POINT('Ctrl Pts',(0.210656937786624,-0.10958550398997,
-0.93342235517345));
#79520=CARTESIAN_POINT('Ctrl Pts',(0.2027722181171,-0.123094138228909,-0.934424965733036));
#79521=CARTESIAN_POINT('Ctrl Pts',(0.200617503706549,-0.126575484638188,
-0.934690186483372));
#79522=CARTESIAN_POINT('Ctrl Pts',(0.197326646982513,-0.131597209075127,
-0.935083968886161));
#79523=CARTESIAN_POINT('Ctrl Pts',(0.196260169098409,-0.133182494031873,
-0.935209970361829));
#79524=CARTESIAN_POINT('Ctrl Pts',(0.194332237145921,-0.135974853394169,
-0.935435036153001));
#79525=CARTESIAN_POINT('Ctrl Pts',(0.193478387075772,-0.137187071963324,
-0.935533809641351));
#79526=CARTESIAN_POINT('Ctrl Pts',(0.191652412792085,-0.139728468202048,
-0.93574320054388));
#79527=CARTESIAN_POINT('Ctrl Pts',(0.190677703206727,-0.14105568197786,
-0.935853913889724));
#79528=CARTESIAN_POINT('Ctrl Pts',(0.18803206828221,-0.144580577432116,
-0.93615168830083));
#79529=CARTESIAN_POINT('Ctrl Pts',(0.186336502464633,-0.146759356789292,
-0.936339702000014));
#79530=CARTESIAN_POINT('Ctrl Pts',(0.176794996504949,-0.158588099291582,
-0.937382921135005));
#79531=CARTESIAN_POINT('Ctrl Pts',(0.168238597987363,-0.167637532785864,
-0.938266581391823));
#79532=CARTESIAN_POINT('Ctrl Pts',(0.146059497676426,-0.187679074047201,
-0.94043187299895));
#79533=CARTESIAN_POINT('Ctrl Pts',(0.131852452782993,-0.19791859963494,
-0.941725639439422));
#79534=CARTESIAN_POINT('Ctrl Pts',(0.114160820006072,-0.207912146388026,
-0.943154650002809));
#79535=CARTESIAN_POINT('Ctrl Pts',(0.111646318887781,-0.209273158137317,
-0.943353709977922));
#79536=CARTESIAN_POINT('Ctrl Pts',(0.108070786129276,-0.211125672514613,
-0.943630501436753));
#79537=CARTESIAN_POINT('Ctrl Pts',(0.107029901337166,-0.211655249808483,
-0.943710343775937));
#79538=CARTESIAN_POINT('Ctrl Pts',(0.105232379963273,-0.212553134131468,
-0.943846910657466));
#79539=CARTESIAN_POINT('Ctrl Pts',(0.104477627775119,-0.212925137098191,
-0.943903856758308));
#79540=CARTESIAN_POINT('Ctrl Pts',(0.102874038487572,-0.213704935721174,
-0.944023993684628));
#79541=CARTESIAN_POINT('Ctrl Pts',(0.102024734816949,-0.214111701942578,
-0.944087122900321));
#79542=CARTESIAN_POINT('Ctrl Pts',(0.0996784290524052,-0.215218312598164,
-0.944260217331233));
#79543=CARTESIAN_POINT('Ctrl Pts',(0.0981764676106642,-0.215907602646411,
-0.944369564149316));
#79544=CARTESIAN_POINT('Ctrl Pts',(0.0898335827235146,-0.219631309546036,
-0.944969596557978));
#79545=CARTESIAN_POINT('Ctrl Pts',(0.082858509684902,-0.222356640966223,
-0.945444164032441));
#79546=CARTESIAN_POINT('Ctrl Pts',(0.0552310604596983,-0.231670230502304,
-0.947263025850331));
#79547=CARTESIAN_POINT('Ctrl Pts',(0.0338456399187812,-0.235745786048531,
-0.94855226219004));
#79548=CARTESIAN_POINT('Ctrl Pts',(0.00783959537356827,-0.237085672763866,
-0.950217867414755));
#79549=CARTESIAN_POINT('Ctrl Pts',(0.00347047608295848,-0.237189855239467,
-0.950500517005462));
#79550=CARTESIAN_POINT('Ctrl Pts',(-0.00285774619201431,-0.237165873104083,
-0.950915249877816));
#79551=CARTESIAN_POINT('Ctrl Pts',(-0.00481645643009057,-0.237134180253688,
-0.951044355814498));
#79552=CARTESIAN_POINT('Ctrl Pts',(-0.00826284334683571,-0.237035699872771,
-0.951272924836401));
#79553=CARTESIAN_POINT('Ctrl Pts',(-0.00975072168636051,-0.236979156991875,
-0.951372063975333));
#79554=CARTESIAN_POINT('Ctrl Pts',(-0.0128587934093212,-0.236831723239201,
-0.951580168173632));
#79555=CARTESIAN_POINT('Ctrl Pts',(-0.0144787786149538,-0.236738206557033,
-0.951689210127748));
#79556=CARTESIAN_POINT('Ctrl Pts',(-0.0187396364615713,-0.23644834337798,
-0.951977583149281));
#79557=CARTESIAN_POINT('Ctrl Pts',(-0.021378337559641,-0.236224382224938,
-0.952157763953975));
#79558=CARTESIAN_POINT('Ctrl Pts',(-0.0339353077155991,-0.234946492717549,
-0.953023140324025));
#79559=CARTESIAN_POINT('Ctrl Pts',(-0.043783057441229,-0.233311928742815,
-0.953726088025518));
#79560=CARTESIAN_POINT('Ctrl Pts',(-0.0690710093377817,-0.22745704596678,
-0.95559130993288));
#79561=CARTESIAN_POINT('Ctrl Pts',(-0.0842388904726483,-0.222286481649304,
-0.956772467794112));
#79562=CARTESIAN_POINT('Ctrl Pts',(-0.104442294603412,-0.213032158306117,
-0.958371278548418));
#79563=CARTESIAN_POINT('Ctrl Pts',(-0.110009504577016,-0.210211362646114,
-0.95881425889012));
#79564=CARTESIAN_POINT('Ctrl Pts',(-0.116795117537509,-0.206429695407859,
-0.959351832413855));
#79565=CARTESIAN_POINT('Ctrl Pts',(-0.118123570667535,-0.205672411826346,
-0.959456956689106));
#79566=CARTESIAN_POINT('Ctrl Pts',(-0.120234982846617,-0.204441596567279,
-0.959623736123055));
#79567=CARTESIAN_POINT('Ctrl Pts',(-0.121022660571354,-0.203976305503068,
-0.959685886229579));
#79568=CARTESIAN_POINT('Ctrl Pts',(-0.122530572155076,-0.203073753529747,
-0.959804704399139));
#79569=CARTESIAN_POINT('Ctrl Pts',(-0.123251192871967,-0.202637197878695,
-0.959861412627666));
#79570=CARTESIAN_POINT('Ctrl Pts',(-0.124848733371003,-0.201657725100745,
-0.959986995165987));
#79571=CARTESIAN_POINT('Ctrl Pts',(-0.125724479764138,-0.201112902624777,
-0.960055747997172));
#79572=CARTESIAN_POINT('Ctrl Pts',(-0.128310582099416,-0.199480532979008,
-0.960258597617436));
#79573=CARTESIAN_POINT('Ctrl Pts',(-0.130010630686126,-0.198376725143669,
-0.960391712239343));
#79574=CARTESIAN_POINT('Ctrl Pts',(-0.143475385024,-0.18938687182922,-0.961445900195743));
#79575=CARTESIAN_POINT('Ctrl Pts',(-0.154527897562318,-0.18048215593357,
-0.962311666027193));
#79576=CARTESIAN_POINT('Ctrl Pts',(-0.175190280963965,-0.160536895272755,
-0.964072759845347));
#79577=CARTESIAN_POINT('Ctrl Pts',(-0.184706539918831,-0.149489684743957,
-0.964965352191268));
#79578=CARTESIAN_POINT('Ctrl Pts',(-0.195470993990589,-0.134384016733147,
-0.966155228931278));
#79579=CARTESIAN_POINT('Ctrl Pts',(-0.197708951521922,-0.131069221931135,
-0.96641446546335));
#79580=CARTESIAN_POINT('Ctrl Pts',(-0.200881452717741,-0.126103957145347,
-0.966801030348078));
#79581=CARTESIAN_POINT('Ctrl Pts',(-0.201881791469812,-0.12449621673432,
-0.966925934562255));
#79582=CARTESIAN_POINT('Ctrl Pts',(-0.203629931297421,-0.121610133161877,
-0.967149780077638));
#79583=CARTESIAN_POINT('Ctrl Pts',(-0.204385219520994,-0.120336425405647,
-0.967248442196158));
#79584=CARTESIAN_POINT('Ctrl Pts',(-0.205959878806111,-0.117623347575269,
-0.967458376303169));
#79585=CARTESIAN_POINT('Ctrl Pts',(-0.206776195673512,-0.116182306030534,
-0.96756975152088));
#79586=CARTESIAN_POINT('Ctrl Pts',(-0.208934448051046,-0.11227754621146,
-0.96787125820561));
#79587=CARTESIAN_POINT('Ctrl Pts',(-0.210247836318726,-0.109798438590742,
-0.968062384457869));
#79588=CARTESIAN_POINT('Ctrl Pts',(-0.217855327254678,-0.0948015864052863,
-0.969217259501373));
#79589=CARTESIAN_POINT('Ctrl Pts',(-0.223073029847663,-0.0817715463605787,
-0.970217751685048));
#79590=CARTESIAN_POINT('Ctrl Pts',(-0.230143598316615,-0.0582810542876215,
-0.97200118546628));
#79591=CARTESIAN_POINT('Ctrl Pts',(-0.232502932319108,-0.0480119339481906,
-0.97277377070854));
#79592=CARTESIAN_POINT('Ctrl Pts',(-0.234947239019236,-0.0327969245437359,
-0.973887166313279));
#79593=CARTESIAN_POINT('Ctrl Pts',(-0.235572931925849,-0.0279507231698396,
-0.974237128396923));
#79594=CARTESIAN_POINT('Ctrl Pts',(-0.236354030232911,-0.0199650137968235,
-0.974802897139983));
#79595=CARTESIAN_POINT('Ctrl Pts',(-0.236597529332452,-0.0168357009774926,
-0.975021863389482));
#79596=CARTESIAN_POINT('Ctrl Pts',(-0.236848795085307,-0.0124937713187137,
-0.975321082821356));
#79597=CARTESIAN_POINT('Ctrl Pts',(-0.236909480417535,-0.0112846932238761,
-0.97540391192189));
#79598=CARTESIAN_POINT('Ctrl Pts',(-0.236996945547756,-0.00922757519841145,
-0.975543939118901));
#79599=CARTESIAN_POINT('Ctrl Pts',(-0.237028436896408,-0.00837976965484352,
-0.975601389024825));
#79600=CARTESIAN_POINT('Ctrl Pts',(-0.237084692688825,-0.00660917387670398,
-0.975720807168831));
#79601=CARTESIAN_POINT('Ctrl Pts',(-0.237108620234517,-0.00568638460834532,
-0.97578272988657));
#79602=CARTESIAN_POINT('Ctrl Pts',(-0.237158629248897,-0.00319691335545359,
-0.97594899037061));
#79603=CARTESIAN_POINT('Ctrl Pts',(-0.2371745748802,-0.00163004199203212,
-0.976052788121025));
#79604=CARTESIAN_POINT('Ctrl Pts',(-0.237176804291559,0.00675282459052012,
-0.976604136278266));
#79605=CARTESIAN_POINT('Ctrl Pts',(-0.236884803550436,0.0135663447479153,
-0.977038236216962));
#79606=CARTESIAN_POINT('Ctrl Pts',(-0.234531519968222,0.0408807918839849,
-0.978755387496812));
#79607=CARTESIAN_POINT('Ctrl Pts',(-0.230097666489288,0.0610851876736562,
-0.979980872939617));
#79608=CARTESIAN_POINT('Ctrl Pts',(-0.221198374569576,0.0857611609345249,
-0.981642806249572));
#79609=CARTESIAN_POINT('Ctrl Pts',(-0.219099792493792,0.0909888497071163,
-0.982004383795237));
#79610=CARTESIAN_POINT('Ctrl Pts',(-0.215919966670541,0.0981603241674078,
-0.982516638991088));
#79611=CARTESIAN_POINT('Ctrl Pts',(-0.214994387093487,0.10017132434792,
-0.982662104474577));
#79612=CARTESIAN_POINT('Ctrl Pts',(-0.213446575958021,0.103413939031685,
-0.982899780081914));
#79613=CARTESIAN_POINT('Ctrl Pts',(-0.212841494215128,0.104653627640114,
-0.982991397594286));
#79614=CARTESIAN_POINT('Ctrl Pts',(-0.211548598945636,0.107244909669007,
-0.983184525314668));
#79615=CARTESIAN_POINT('Ctrl Pts',(-0.210858569625071,0.108595321249922,
-0.983286109423759));
#79616=CARTESIAN_POINT('Ctrl Pts',(-0.20916926372872,0.111824541026068,
-0.983531340483627));
#79617=CARTESIAN_POINT('Ctrl Pts',(-0.208157573921936,0.113696670007702,
-0.983675418917355));
#79618=CARTESIAN_POINT('Ctrl Pts',(-0.204465647789918,0.120314087666368,
-0.984191681042377));
#79619=CARTESIAN_POINT('Ctrl Pts',(-0.201647396242047,0.124979998622409,
-0.984568713108398));
#79620=CARTESIAN_POINT('Ctrl Pts',(-0.194085521389976,0.136576997967156,
-0.985540091974101));
#79621=CARTESIAN_POINT('Ctrl Pts',(-0.18913014063275,0.143360496846779,
-0.986141210838845));
#79622=CARTESIAN_POINT('Ctrl Pts',(-0.172249803260152,0.164065895495319,
-0.988076706470161));
#79623=CARTESIAN_POINT('Ctrl Pts',(-0.159067255915847,0.17687641688348,
-0.989435959969911));
#79624=CARTESIAN_POINT('Ctrl Pts',(-0.142790248278858,0.189387969247969,
-0.990869878302855));
#79625=CARTESIAN_POINT('Ctrl Pts',(-0.141020501855693,0.190709404138559,
-0.991022827030757));
#79626=CARTESIAN_POINT('Ctrl Pts',(-0.138378553212631,0.192625204109848,
-0.991246526366501));
#79627=CARTESIAN_POINT('Ctrl Pts',(-0.137520486135181,0.193238736404825,
-0.991318473394183));
#79628=CARTESIAN_POINT('Ctrl Pts',(-0.135980017646399,0.194324739071332,
-0.991446339114255));
#79629=CARTESIAN_POINT('Ctrl Pts',(-0.135299199578616,0.194799373896884,
-0.991502399092463));
#79630=CARTESIAN_POINT('Ctrl Pts',(-0.133780130516193,0.195846592271087,
-0.991626483754823));
#79631=CARTESIAN_POINT('Ctrl Pts',(-0.132940682336721,0.196417377285793,
-0.991694389692887));
#79632=CARTESIAN_POINT('Ctrl Pts',(-0.130432651398717,0.198099274696238,
-0.991895389534579));
#79633=CARTESIAN_POINT('Ctrl Pts',(-0.128753570566453,0.199194673382225,
-0.992027496703202));
#79634=CARTESIAN_POINT('Ctrl Pts',(-0.116463658670243,0.206992024070043,
-0.99297830901679));
#79635=CARTESIAN_POINT('Ctrl Pts',(-0.105348180682879,0.212864571647068,
-0.993752479754958));
#79636=CARTESIAN_POINT('Ctrl Pts',(-0.0776842685374338,0.224779332082987,
-0.995601714421009));
#79637=CARTESIAN_POINT('Ctrl Pts',(-0.0608295107684455,0.229913653799764,
-0.996671092514741));
#79638=CARTESIAN_POINT('Ctrl Pts',(-0.0430210306692712,0.233241239222924,
-0.997839698133149));
#79639=CARTESIAN_POINT('Ctrl Pts',(-0.042478593486725,0.233340639033401,
-0.997875324044025));
#79640=CARTESIAN_POINT('Ctrl Pts',(-0.0419358256939468,0.233438144158933,
-0.997911004226539));
#79641=CARTESIAN_POINT('',(-0.237174942067321,-0.00016577202159111,-0.995658989184409));
#79642=CARTESIAN_POINT('Ctrl Pts',(-0.0419358384531397,0.233438141866817,
-1.01783655831731));
#79643=CARTESIAN_POINT('Ctrl Pts',(-0.055592946826114,0.230984719791547,
-1.01698515986923));
#79644=CARTESIAN_POINT('Ctrl Pts',(-0.069012121426973,0.227336927612748,
-1.01612846358432));
#79645=CARTESIAN_POINT('Ctrl Pts',(-0.0849425892911568,0.221464019903327,
-1.01503406101721));
#79646=CARTESIAN_POINT('Ctrl Pts',(-0.0878245833239149,0.220337007194613,
-1.01483293535467));
#79647=CARTESIAN_POINT('Ctrl Pts',(-0.0924381062532635,0.218427980104624,
-1.01450540334796));
#79648=CARTESIAN_POINT('Ctrl Pts',(-0.0941837853024383,0.21768095970503,
-1.01438016221878));
#79649=CARTESIAN_POINT('Ctrl Pts',(-0.0972747531210218,0.216314115171633,
-1.01415596832755));
#79650=CARTESIAN_POINT('Ctrl Pts',(-0.0986235736721244,0.215702490860777,
-1.01405729854005));
#79651=CARTESIAN_POINT('Ctrl Pts',(-0.101464987729986,0.214381825853848,
-1.01384761782651));
#79652=CARTESIAN_POINT('Ctrl Pts',(-0.102956070470368,0.213669741202609,
-1.01373650625723));
#79653=CARTESIAN_POINT('Ctrl Pts',(-0.106943571968904,0.211714032113678,
-1.01343639235263));
#79654=CARTESIAN_POINT('Ctrl Pts',(-0.109425630478381,0.210441890369043,
-1.01324641061616));
#79655=CARTESIAN_POINT('Ctrl Pts',(-0.125199291740754,0.202002830148127,
-1.01201803951623));
#79656=CARTESIAN_POINT('Ctrl Pts',(-0.137800888181475,0.193625336759183,
-1.01093637717332));
#79657=CARTESIAN_POINT('Ctrl Pts',(-0.161823302152502,0.174116199737272,
-1.008682628341));
#79658=CARTESIAN_POINT('Ctrl Pts',(-0.173095748347187,0.162914595846265,
-1.00751457028428));
#79659=CARTESIAN_POINT('Ctrl Pts',(-0.184504154036458,0.149045727716184,
-1.00626183067727));
#79660=CARTESIAN_POINT('Ctrl Pts',(-0.185819788098912,0.147402235121337,
-1.00611618535596));
#79661=CARTESIAN_POINT('Ctrl Pts',(-0.187749257879857,0.144925040901263,
-1.0059010679874));
#79662=CARTESIAN_POINT('Ctrl Pts',(-0.188379760875563,0.144104535348781,
-1.00583052295506));
#79663=CARTESIAN_POINT('Ctrl Pts',(-0.189505883057362,0.142619033322668,
-1.00570410970204));
#79664=CARTESIAN_POINT('Ctrl Pts',(-0.190003402434016,0.141955540567041,
-1.00564811461029));
#79665=CARTESIAN_POINT('Ctrl Pts',(-0.191112958528264,0.140459550157149,
-1.00552290146471));
#79666=CARTESIAN_POINT('Ctrl Pts',(-0.191723045335776,0.139625649988255,
-1.00545381553612));
#79667=CARTESIAN_POINT('Ctrl Pts',(-0.193554890896918,0.13708713667679,
-1.0052455617486));
#79668=CARTESIAN_POINT('Ctrl Pts',(-0.194759545791538,0.135370228984546,
-1.0051074899361));
#79669=CARTESIAN_POINT('Ctrl Pts',(-0.197530986951853,0.131306700051836,
-1.00478658416685));
#79670=CARTESIAN_POINT('Ctrl Pts',(-0.199079014492286,0.128947616244146,
-1.00460477594465));
#79671=CARTESIAN_POINT('Ctrl Pts',(-0.209825244877523,0.111916124700385,
-1.00331965870747));
#79672=CARTESIAN_POINT('Ctrl Pts',(-0.21743493112877,0.096301697396637,
-1.00228138320339));
#79673=CARTESIAN_POINT('Ctrl Pts',(-0.226965413984013,0.0697013506874559,
-1.00053463564309));
#79674=CARTESIAN_POINT('Ctrl Pts',(-0.229937143142169,0.059164555169512,
-0.999848561577447));
#79675=CARTESIAN_POINT('Ctrl Pts',(-0.232728571919164,0.0457911769869978,
-0.998961868290114));
#79676=CARTESIAN_POINT('Ctrl Pts',(-0.233239761376087,0.043111863716989,
-0.998783492065912));
#79677=CARTESIAN_POINT('Ctrl Pts',(-0.23398401988198,0.038809101737257,
-0.998495576213637));
#79678=CARTESIAN_POINT('Ctrl Pts',(-0.234246664096322,0.0371909675907741,
-0.998386972906712));
#79679=CARTESIAN_POINT('Ctrl Pts',(-0.234707754011815,0.0341512909935617,
-0.998182287846869));
#79680=CARTESIAN_POINT('Ctrl Pts',(-0.23491011161308,0.0327304105710576,
-0.99808633438141));
#79681=CARTESIAN_POINT('Ctrl Pts',(-0.235289166899945,0.0298839726597515,
-0.99789352695911));
#79682=CARTESIAN_POINT('Ctrl Pts',(-0.235465834169476,0.0284584726186601,
-0.997796676386154));
#79683=CARTESIAN_POINT('Ctrl Pts',(-0.235840539784608,0.0251922177554452,
-0.99757406024522));
#79684=CARTESIAN_POINT('Ctrl Pts',(-0.236029992892698,0.0233505922664693,
-0.997448032424324));
#79685=CARTESIAN_POINT('Ctrl Pts',(-0.236854354096121,0.0142971437432219,
-0.99682586748679));
#79686=CARTESIAN_POINT('Ctrl Pts',(-0.237180312975127,0.00706187281541956,
-0.996320355240562));
#79687=CARTESIAN_POINT('Ctrl Pts',(-0.237174934520829,-0.000176238589683619,
-0.995806388174485));
#79688=CARTESIAN_POINT('Ctrl Pts',(-0.237174942067321,-0.00016577202159111,
-0.995658989184409));
#79689=CARTESIAN_POINT('Ctrl Pts',(-0.237163585248673,-0.0164143088910714,
-0.99457247635419));
#79690=CARTESIAN_POINT('Ctrl Pts',(-0.23547834423869,-0.0325957541205758,
-0.993485963523971));
#79691=CARTESIAN_POINT('Ctrl Pts',(-0.232184488208474,-0.0483977691672791,
-0.992399450693752));
#79692=CARTESIAN_POINT('Ctrl Pts',(-0.229804709060592,-0.0598145723176513,
-0.99161445567468));
#79693=CARTESIAN_POINT('Ctrl Pts',(-0.226586336671938,-0.071033649634856,
-0.990829460655608));
#79694=CARTESIAN_POINT('Ctrl Pts',(-0.222569518205059,-0.0819438233850974,
-0.990044465636536));
#79695=CARTESIAN_POINT('Ctrl Pts',(-0.217718298757162,-0.0951203329818135,
-0.98909640608781));
#79696=CARTESIAN_POINT('Ctrl Pts',(-0.211676632312198,-0.107908762849582,
-0.988148346539084));
#79697=CARTESIAN_POINT('Ctrl Pts',(-0.204528599500758,-0.120083440204129,
-0.987200286990358));
#79698=CARTESIAN_POINT('Ctrl Pts',(-0.197394987953441,-0.132233554963291,
-0.986254140166086));
#79699=CARTESIAN_POINT('Ctrl Pts',(-0.189159797849578,-0.143771627616582,
-0.985307993341815));
#79700=CARTESIAN_POINT('Ctrl Pts',(-0.179953918574813,-0.154494555938291,
-0.984361846517543));
#79701=CARTESIAN_POINT('Ctrl Pts',(-0.170749497480443,-0.165215785784125,
-0.983415849559754));
#79702=CARTESIAN_POINT('Ctrl Pts',(-0.160575197282862,-0.175121463826213,
-0.982469852601965));
#79703=CARTESIAN_POINT('Ctrl Pts',(-0.149602964644826,-0.184040575945847,
-0.981523855644176));
#79704=CARTESIAN_POINT('Ctrl Pts',(-0.138632511781998,-0.192958241321216,
-0.980578012133911));
#79705=CARTESIAN_POINT('Ctrl Pts',(-0.12686504275345,-0.200889146492325,
-0.979632168623647));
#79706=CARTESIAN_POINT('Ctrl Pts',(-0.114504790606895,-0.207703234334642,
-0.978686325113382));
#79707=CARTESIAN_POINT('Ctrl Pts',(-0.102115785638396,-0.214533173330489,
-0.977738281351074));
#79708=CARTESIAN_POINT('Ctrl Pts',(-0.0891319983572828,-0.220240744143584,
-0.976790237588767));
#79709=CARTESIAN_POINT('Ctrl Pts',(-0.0757809214441986,-0.224742591802418,
-0.975842193826459));
#79710=CARTESIAN_POINT('Ctrl Pts',(-0.0680257844447021,-0.227357545305599,
-0.97529151096349));
#79711=CARTESIAN_POINT('Ctrl Pts',(-0.0601470726480214,-0.229566609646384,
-0.974740828100521));
#79712=CARTESIAN_POINT('Ctrl Pts',(-0.0521911341244206,-0.231361332430047,
-0.974190145237552));
#79713=CARTESIAN_POINT('Ctrl Pts',(-0.0384941335573052,-0.234451139988606,
-0.973242085688825));
#79714=CARTESIAN_POINT('Ctrl Pts',(-0.0244758356660067,-0.236330766586181,
-0.972294026140098));
#79715=CARTESIAN_POINT('Ctrl Pts',(-0.0103713680518171,-0.23694812797263,
-0.971345966591371));
#79716=CARTESIAN_POINT('Ctrl Pts',(0.00370464358600231,-0.23756424382316,
-0.970399819767098));
#79717=CARTESIAN_POINT('Ctrl Pts',(0.0178656583111794,-0.236923042955139,
-0.969453672942825));
#79718=CARTESIAN_POINT('Ctrl Pts',(0.0318700518927368,-0.23502399966249,
-0.968507526118551));
#79719=CARTESIAN_POINT('Ctrl Pts',(0.0458722272253272,-0.233125257171929,
-0.967561529160761));
#79720=CARTESIAN_POINT('Ctrl Pts',(0.0597169990888082,-0.22996913074344,
-0.966615532202972));
#79721=CARTESIAN_POINT('Ctrl Pts',(0.073167361654758,-0.225606998591537,
-0.965669535245182));
#79722=CARTESIAN_POINT('Ctrl Pts',(0.0866155424749664,-0.221245574008906,
-0.964723691734916));
#79723=CARTESIAN_POINT('Ctrl Pts',(0.0996686528945936,-0.215678807214401,
-0.96377784822465));
#79724=CARTESIAN_POINT('Ctrl Pts',(0.112106517191718,-0.20900743869093,
-0.962832004714384));
#79725=CARTESIAN_POINT('Ctrl Pts',(0.124573314854705,-0.202320551012267,
-0.961883960952075));
#79726=CARTESIAN_POINT('Ctrl Pts',(0.136421293702348,-0.194524366434287,
-0.960935917189766));
#79727=CARTESIAN_POINT('Ctrl Pts',(0.14745683687118,-0.18576453344206,-0.959987873427458));
#79728=CARTESIAN_POINT('Ctrl Pts',(0.153866967656463,-0.180676276862538,
-0.959437190564494));
#79729=CARTESIAN_POINT('Ctrl Pts',(0.160003566873437,-0.175263679067963,
-0.95888650770153));
#79730=CARTESIAN_POINT('Ctrl Pts',(0.165834347993985,-0.169561049921289,
-0.958335824838567));
#79731=CARTESIAN_POINT('Ctrl Pts',(0.175872662402621,-0.159743362865875,
-0.957387765289839));
#79732=CARTESIAN_POINT('Ctrl Pts',(0.185069800982204,-0.148998209825383,
-0.956439705741112));
#79733=CARTESIAN_POINT('Ctrl Pts',(0.193254245309879,-0.137494644603742,
-0.955491646192384));
#79734=CARTESIAN_POINT('Ctrl Pts',(0.201422177397549,-0.126014287998623,
-0.954545499368111));
#79735=CARTESIAN_POINT('Ctrl Pts',(0.208580934834249,-0.113779188139508,
-0.953599352543837));
#79736=CARTESIAN_POINT('Ctrl Pts',(0.214598745691559,-0.100991875775281,
-0.952653205719564));
#79737=CARTESIAN_POINT('Ctrl Pts',(0.220615603347815,-0.0882065888784383,
-0.951707208761774));
#79738=CARTESIAN_POINT('Ctrl Pts',(0.225491474053488,-0.074869995353623,
-0.950761211803983));
#79739=CARTESIAN_POINT('Ctrl Pts',(0.229140663662373,-0.0612089607930668,
-0.949815214846193));
#79740=CARTESIAN_POINT('Ctrl Pts',(0.232789261346405,-0.0475501421507673,
-0.948869371335927));
#79741=CARTESIAN_POINT('Ctrl Pts',(0.235211375546206,-0.0335677980348952,
-0.94792352782566));
#79742=CARTESIAN_POINT('Ctrl Pts',(0.236371893925085,-0.0195014970519764,
-0.946977684315394));
#79743=CARTESIAN_POINT('Ctrl Pts',(0.237535111939693,-0.00540247458063008,
-0.946029640553085));
#79744=CARTESIAN_POINT('Ctrl Pts',(0.237430851188402,0.00878005786051047,
-0.945081596790776));
#79745=CARTESIAN_POINT('Ctrl Pts',(0.236076130180546,0.0228044158876671,
-0.944133553028467));
#79746=CARTESIAN_POINT('Ctrl Pts',(0.235289223844806,0.0309506364912213,
-0.943582870165505));
#79747=CARTESIAN_POINT('Ctrl Pts',(0.234081396039,0.0390435480085086,-0.943032187302543));
#79748=CARTESIAN_POINT('Ctrl Pts',(0.232463897269428,0.0470374009837774,
-0.942481504439582));
#79749=CARTESIAN_POINT('Ctrl Pts',(0.229679199838862,0.0607996753417688,
-0.941533444890855));
#79750=CARTESIAN_POINT('Ctrl Pts',(0.225658792039843,0.0743599848162986,
-0.940585385342128));
#79751=CARTESIAN_POINT('Ctrl Pts',(0.220451349750043,0.0874824726352891,
-0.939637325793401));
#79752=CARTESIAN_POINT('Ctrl Pts',(0.215254413553688,0.100578485636974,
-0.938691178969128));
#79753=CARTESIAN_POINT('Ctrl Pts',(0.208875435538092,0.113237637112344,
-0.937745032144855));
#79754=CARTESIAN_POINT('Ctrl Pts',(0.201412795245007,0.125239237208604,
-0.936798885320582));
#79755=CARTESIAN_POINT('Ctrl Pts',(0.193951337009112,0.137238936291666,
-0.935852888362792));
#79756=CARTESIAN_POINT('Ctrl Pts',(0.185406954935095,0.148580557734724,
-0.934906891405002));
#79757=CARTESIAN_POINT('Ctrl Pts',(0.175923499719716,0.159068862042095,
-0.933960894447212));
#79758=CARTESIAN_POINT('Ctrl Pts',(0.166441582789117,0.169555465070921,
-0.933015050936947));
#79759=CARTESIAN_POINT('Ctrl Pts',(0.156021468637956,0.179188419199748,
-0.932069207426681));
#79760=CARTESIAN_POINT('Ctrl Pts',(0.144845163585783,0.187808038195408,
-0.931123363916415));
#79761=CARTESIAN_POINT('Ctrl Pts',(0.133642859848036,0.196447708430093,
-0.930175320154107));
#79762=CARTESIAN_POINT('Ctrl Pts',(0.121681542756846,0.204068862554768,
-0.929227276391798));
#79763=CARTESIAN_POINT('Ctrl Pts',(0.109173329406417,0.210554422350418,
-0.928279232629489));
#79764=CARTESIAN_POINT('Ctrl Pts',(0.101907780059194,0.214321639411681,
-0.927728549766525));
#79765=CARTESIAN_POINT('Ctrl Pts',(0.0944581931614917,0.217706564800712,
-0.927177866903561));
#79766=CARTESIAN_POINT('Ctrl Pts',(0.0868690852762904,0.220693775735204,
-0.926627184040597));
#79767=CARTESIAN_POINT('Ctrl Pts',(0.0738038378845529,0.225836494808489,
-0.925679140087625));
#79768=CARTESIAN_POINT('Ctrl Pts',(0.060236485051065,0.229832236751135,
-0.924731096134653));
#79769=CARTESIAN_POINT('Ctrl Pts',(0.046391447811875,0.232593667572697,
-0.923783052181681));
#79770=CARTESIAN_POINT('Ctrl Pts',(0.0319084307160987,0.235482345234341,
-0.922791322326338));
#79771=CARTESIAN_POINT('Ctrl Pts',(0.0171223396133438,0.237019582137728,
-0.921799592470995));
#79772=CARTESIAN_POINT('Ctrl Pts',(0.00230831192544603,0.237163766880725,
-0.920807862615652));
#79773=CARTESIAN_POINT('Ctrl Pts',(-0.0125057157624517,0.237307951623722,
-0.919816132760309));
#79774=CARTESIAN_POINT('Ctrl Pts',(-0.0273466268406475,0.236059010181803,
-0.918824402904966));
#79775=CARTESIAN_POINT('Ctrl Pts',(-0.0419358257166344,0.233438144154858,
-0.917832673049623));
#79776=CARTESIAN_POINT('Origin',(0.,0.,-1.7456589891905));
#79777=CARTESIAN_POINT('',(-0.0419357988072456,0.233438148988974,-0.798166224572097));
#79778=CARTESIAN_POINT('',(-0.0419725940269791,0.233652521193877,-0.817841625530981));
#79779=CARTESIAN_POINT('',(-0.0419358257166344,0.233438144154858,-1.7456589891905));
#79780=CARTESIAN_POINT('',(-0.237174902566701,0.000214982501742253,-0.87588669733343));
#79781=CARTESIAN_POINT('Ctrl Pts',(-0.0419357988072473,0.233438148988973,
-0.798166224572096));
#79782=CARTESIAN_POINT('Ctrl Pts',(-0.0313505303885184,0.235339730579862,
-0.798950663251301));
#79783=CARTESIAN_POINT('Ctrl Pts',(-0.0206424454919457,0.236520164301066,
-0.799731423587888));
#79784=CARTESIAN_POINT('Ctrl Pts',(-0.00773759091582227,0.237058496772595,
-0.800632917265799));
#79785=CARTESIAN_POINT('Ctrl Pts',(-0.00558869131939521,0.237118891153116,
-0.800781705334997));
#79786=CARTESIAN_POINT('Ctrl Pts',(-0.00239573691432892,0.237165195726478,
-0.801000528277506));
#79787=CARTESIAN_POINT('Ctrl Pts',(-0.00135218428014268,0.237173441431424,
-0.801071688460254));
#79788=CARTESIAN_POINT('Ctrl Pts',(0.000521048498413145,0.237175878683289,
-0.801198742591875));
#79789=CARTESIAN_POINT('Ctrl Pts',(0.00135067642484936,0.23717260518958,
-0.801254769673511));
#79790=CARTESIAN_POINT('Ctrl Pts',(0.00320559434414651,0.237155552499976,
-0.801379495737443));
#79791=CARTESIAN_POINT('Ctrl Pts',(0.00423082805610003,0.237139478173074,
-0.801448068472577));
#79792=CARTESIAN_POINT('Ctrl Pts',(0.00731158285574852,0.237071189915555,
-0.801653115216069));
#79793=CARTESIAN_POINT('Ctrl Pts',(0.00936662263562405,0.236998893271651,
-0.801788542367449));
#79794=CARTESIAN_POINT('Ctrl Pts',(0.0141660993478863,0.236767518537997,
-0.802102213752993));
#79795=CARTESIAN_POINT('Ctrl Pts',(0.0169092692564717,0.236587434541174,
-0.802279494950369));
#79796=CARTESIAN_POINT('Ctrl Pts',(0.0267707555675258,0.235767639680444,
-0.802911582093368));
#79797=CARTESIAN_POINT('Ctrl Pts',(0.0338628208650324,0.234853948012336,
-0.803356400021272));
#79798=CARTESIAN_POINT('Ctrl Pts',(0.0578518690443821,0.230653861070634,
-0.804858891986051));
#79799=CARTESIAN_POINT('Ctrl Pts',(0.0744262271455292,0.225851175732788,
-0.805897325575825));
#79800=CARTESIAN_POINT('Ctrl Pts',(0.0951789250522059,0.217302547967147,
-0.807323036174596));
#79801=CARTESIAN_POINT('Ctrl Pts',(0.0999550525873154,0.215147405769776,
-0.807660058752244));
#79802=CARTESIAN_POINT('Ctrl Pts',(0.106587427359322,0.211886136863276,
-0.808143063357768));
#79803=CARTESIAN_POINT('Ctrl Pts',(0.108506124442552,0.210910016648227,
-0.808284610420606));
#79804=CARTESIAN_POINT('Ctrl Pts',(0.111743984749855,0.209206907655467,
-0.808526725806087));
#79805=CARTESIAN_POINT('Ctrl Pts',(0.113070017559556,0.208493211616066,
-0.808626824018616));
#79806=CARTESIAN_POINT('Ctrl Pts',(0.115750026286485,0.207017693544718,
-0.808831101478219));
#79807=CARTESIAN_POINT('Ctrl Pts',(0.117103490873556,0.206255099943955,
-0.808935304531674));
#79808=CARTESIAN_POINT('Ctrl Pts',(0.120458173629493,0.204321279883737,
-0.809196236131926));
#79809=CARTESIAN_POINT('Ctrl Pts',(0.122449854276526,0.203133920190778,
-0.809353539219415));
#79810=CARTESIAN_POINT('Ctrl Pts',(0.130349808864888,0.198265884837244,
-0.809987319821));
#79811=CARTESIAN_POINT('Ctrl Pts',(0.136111661532759,0.194355427874229,
-0.810472073058823));
#79812=CARTESIAN_POINT('Ctrl Pts',(0.151725078004736,0.182723798572182,
-0.811850733306218));
#79813=CARTESIAN_POINT('Ctrl Pts',(0.161149405734649,0.17446861236761,-0.81276156678856));
#79814=CARTESIAN_POINT('Ctrl Pts',(0.178334889008115,0.156829572738885,
-0.814559265563252));
#79815=CARTESIAN_POINT('Ctrl Pts',(0.186114967456051,0.147513121454618,
-0.81544313942304));
#79816=CARTESIAN_POINT('Ctrl Pts',(0.194480916801083,0.13577340810298,-0.816451003309508));
#79817=CARTESIAN_POINT('Ctrl Pts',(0.195785380974853,0.133885514207047,
-0.816610034666844));
#79818=CARTESIAN_POINT('Ctrl Pts',(0.197658237439339,0.131089086919469,
-0.816840836304333));
#79819=CARTESIAN_POINT('Ctrl Pts',(0.198248155764343,0.130195224122643,
-0.816913910393796));
#79820=CARTESIAN_POINT('Ctrl Pts',(0.1992848767388,0.12860096655052,-0.817042961276389));
#79821=CARTESIAN_POINT('Ctrl Pts',(0.199734078162534,0.127902184438335,
-0.817099090955306));
#79822=CARTESIAN_POINT('Ctrl Pts',(0.200716795547122,0.126355656022187,
-0.817222357081028));
#79823=CARTESIAN_POINT('Ctrl Pts',(0.201248621552795,0.125506877253641,
-0.817289384784154));
#79824=CARTESIAN_POINT('Ctrl Pts',(0.202793535346434,0.123006169340596,
-0.817485118898756));
#79825=CARTESIAN_POINT('Ctrl Pts',(0.203791802079835,0.121345118035626,
-0.817612914212986));
#79826=CARTESIAN_POINT('Ctrl Pts',(0.206053099904848,0.117475831025437,
-0.817905962876084));
#79827=CARTESIAN_POINT('Ctrl Pts',(0.20730120577119,0.115259108322226,-0.818070419497504));
#79828=CARTESIAN_POINT('Ctrl Pts',(0.211521920149926,0.107472387532533,
-0.818637790437155));
#79829=CARTESIAN_POINT('Ctrl Pts',(0.214307785370698,0.101803834609038,
-0.819032767262254));
#79830=CARTESIAN_POINT('Ctrl Pts',(0.225594897074708,0.0763143162073501,
-0.820759022301788));
#79831=CARTESIAN_POINT('Ctrl Pts',(0.231595545126583,0.0555014073332016,
-0.822049855728221));
#79832=CARTESIAN_POINT('Ctrl Pts',(0.235122646530788,0.0312709182436343,
-0.823630897655418));
#79833=CARTESIAN_POINT('Ctrl Pts',(0.235490257000925,0.0283701761924342,
-0.823821193578872));
#79834=CARTESIAN_POINT('Ctrl Pts',(0.23600271011883,0.0236246121801196,
-0.824134573250991));
#79835=CARTESIAN_POINT('Ctrl Pts',(0.236179759789948,0.0217835310958926,
-0.824256654046997));
#79836=CARTESIAN_POINT('Ctrl Pts',(0.236459398030211,0.0184692706802739,
-0.824477411771021));
#79837=CARTESIAN_POINT('Ctrl Pts',(0.236569795975551,0.0169968332302047,
-0.824575839407845));
#79838=CARTESIAN_POINT('Ctrl Pts',(0.236776632342303,0.0138434682858655,
-0.824787426670993));
#79839=CARTESIAN_POINT('Ctrl Pts',(0.236868934157923,0.0121623605964905,
-0.824900709980918));
#79840=CARTESIAN_POINT('Ctrl Pts',(0.237073024718818,0.00754825537854731,
-0.825213028893489));
#79841=CARTESIAN_POINT('Ctrl Pts',(0.237148275612999,0.00461402659129783,
-0.825413185681062));
#79842=CARTESIAN_POINT('Ctrl Pts',(0.23727814123191,-0.0137273667745005,
-0.826674517661553));
#79843=CARTESIAN_POINT('Ctrl Pts',(0.235885745392215,-0.0291052450653689,
-0.827780535774551));
#79844=CARTESIAN_POINT('Ctrl Pts',(0.230180700180887,-0.059155944858936,
-0.830009825768871));
#79845=CARTESIAN_POINT('Ctrl Pts',(0.225921901876457,-0.0737695390719033,
-0.831126936641177));
#79846=CARTESIAN_POINT('Ctrl Pts',(0.219493212181919,-0.0898854205187167,
-0.832338150587589));
#79847=CARTESIAN_POINT('Ctrl Pts',(0.218664327372071,-0.0918834684372917,
-0.832487885336042));
#79848=CARTESIAN_POINT('Ctrl Pts',(0.217394148488585,-0.0948306870701711,
-0.832707819121343));
#79849=CARTESIAN_POINT('Ctrl Pts',(0.216973746867276,-0.0957886646831998,
-0.832779159479583));
#79850=CARTESIAN_POINT('Ctrl Pts',(0.216208581340307,-0.0975013761813056,
-0.832906398213576));
#79851=CARTESIAN_POINT('Ctrl Pts',(0.215866182390205,-0.0982571135452776,
-0.832962431593476));
#79852=CARTESIAN_POINT('Ctrl Pts',(0.21509278039432,-0.0999405963812236,
-0.833087005315389));
#79853=CARTESIAN_POINT('Ctrl Pts',(0.214659734911456,-0.100867364828591,
-0.833155421168655));
#79854=CARTESIAN_POINT('Ctrl Pts',(0.213343465269904,-0.103637465355318,
-0.833359511830507));
#79855=CARTESIAN_POINT('Ctrl Pts',(0.212442369088613,-0.105472266036051,
-0.833494154143036));
#79856=CARTESIAN_POINT('Ctrl Pts',(0.20522117803054,-0.119707835901997,
-0.834536346054862));
#79857=CARTESIAN_POINT('Ctrl Pts',(0.197843421773374,-0.131543849740473,
-0.835389216138793));
#79858=CARTESIAN_POINT('Ctrl Pts',(0.179850938551566,-0.155439020156128,
-0.837223677738599));
#79859=CARTESIAN_POINT('Ctrl Pts',(0.168966982884659,-0.16720566685208,
-0.83820260917595));
#79860=CARTESIAN_POINT('Ctrl Pts',(0.154657817767472,-0.179840373342346,
-0.839432955434803));
#79861=CARTESIAN_POINT('Ctrl Pts',(0.152292897754663,-0.18184738753357,
-0.839634540738782));
#79862=CARTESIAN_POINT('Ctrl Pts',(0.148416025697946,-0.185008860028065,
-0.839962691842541));
#79863=CARTESIAN_POINT('Ctrl Pts',(0.146928309207657,-0.186192552420041,
-0.840088085510707));
#79864=CARTESIAN_POINT('Ctrl Pts',(0.144256117361922,-0.188266695189936,
-0.840312474077857));
#79865=CARTESIAN_POINT('Ctrl Pts',(0.143077211867114,-0.189164180510896,
-0.840411184602881));
#79866=CARTESIAN_POINT('Ctrl Pts',(0.14056633942817,-0.191038774898792,
-0.840620870140371));
#79867=CARTESIAN_POINT('Ctrl Pts',(0.139232423437442,-0.192013127988283,
-0.840731945086161));
#79868=CARTESIAN_POINT('Ctrl Pts',(0.135622406275613,-0.194592652480213,
-0.841031757625378));
#79869=CARTESIAN_POINT('Ctrl Pts',(0.133328088124021,-0.196171754474485,
-0.841221470777826));
#79870=CARTESIAN_POINT('Ctrl Pts',(0.118615927055236,-0.205920323341553,
-0.842433284075799));
#79871=CARTESIAN_POINT('Ctrl Pts',(0.105483112612292,-0.212946206355859,
-0.843497207005598));
#79872=CARTESIAN_POINT('Ctrl Pts',(0.0768930563187806,-0.224944776934417,
-0.845754454897625));
#79873=CARTESIAN_POINT('Ctrl Pts',(0.0614043772829213,-0.2296568510206,
-0.846945182757649));
#79874=CARTESIAN_POINT('Ctrl Pts',(0.0435224776969564,-0.233156747777846,
-0.848215756403463));
#79875=CARTESIAN_POINT('Ctrl Pts',(0.0414835367088001,-0.233528139651552,
-0.848359092360264));
#79876=CARTESIAN_POINT('Ctrl Pts',(0.038425713185093,-0.234043805790342,
-0.848571502632581));
#79877=CARTESIAN_POINT('Ctrl Pts',(0.0374103952715134,-0.234208242569475,
-0.848641611970352));
#79878=CARTESIAN_POINT('Ctrl Pts',(0.0355742498664127,-0.234493372173651,
-0.848767605397444));
#79879=CARTESIAN_POINT('Ctrl Pts',(0.0347538321768465,-0.234616367818152,
-0.848823611645411));
#79880=CARTESIAN_POINT('Ctrl Pts',(0.0329032437455452,-0.234883884493721,
-0.848949296615929));
#79881=CARTESIAN_POINT('Ctrl Pts',(0.0318727513889932,-0.235025935726976,
-0.849018838306567));
#79882=CARTESIAN_POINT('Ctrl Pts',(0.0287272171535784,-0.235438471760219,
-0.849229846032715));
#79883=CARTESIAN_POINT('Ctrl Pts',(0.0266093672971932,-0.235687227777629,
-0.849370173467309));
#79884=CARTESIAN_POINT('Ctrl Pts',(0.0126418887242216,-0.237137121539453,
-0.85028590792747));
#79885=CARTESIAN_POINT('Ctrl Pts',(0.000718042601137179,-0.237472919934315,
-0.851022069231414));
#79886=CARTESIAN_POINT('Ctrl Pts',(-0.0292519667418776,-0.236058382514719,
-0.852865126087821));
#79887=CARTESIAN_POINT('Ctrl Pts',(-0.0471631501467768,-0.233141155909607,
-0.853964325181293));
#79888=CARTESIAN_POINT('Ctrl Pts',(-0.0674324281551723,-0.227406484930319,
-0.855323736490781));
#79889=CARTESIAN_POINT('Ctrl Pts',(-0.0702811419881151,-0.226542273257707,
-0.855517397569422));
#79890=CARTESIAN_POINT('Ctrl Pts',(-0.0748869501440595,-0.225049780471825,
-0.855835185707767));
#79891=CARTESIAN_POINT('Ctrl Pts',(-0.0766542751552424,-0.224453961342068,
-0.855958260632406));
#79892=CARTESIAN_POINT('Ctrl Pts',(-0.0798091627026552,-0.223348746221201,
-0.856180096272979));
#79893=CARTESIAN_POINT('Ctrl Pts',(-0.0811993514392261,-0.222847100153498,
-0.856278597178528));
#79894=CARTESIAN_POINT('Ctrl Pts',(-0.0841534494289636,-0.22174980940939,
-0.856489556940586));
#79895=CARTESIAN_POINT('Ctrl Pts',(-0.0857159174386802,-0.221150542104236,
-0.856602131977871));
#79896=CARTESIAN_POINT('Ctrl Pts',(-0.0899561287354448,-0.219472570186539,
-0.856910426842706));
#79897=CARTESIAN_POINT('Ctrl Pts',(-0.0926206529295792,-0.218361460738713,
-0.857107220059606));
#79898=CARTESIAN_POINT('Ctrl Pts',(-0.098503298920414,-0.215781350585711,
-0.857548741898548));
#79899=CARTESIAN_POINT('Ctrl Pts',(-0.101710121856105,-0.214288450483594,
-0.857794226949027));
#79900=CARTESIAN_POINT('Ctrl Pts',(-0.111882859661351,-0.209272857421391,
-0.858588615694429));
#79901=CARTESIAN_POINT('Ctrl Pts',(-0.118708218240034,-0.205478082047925,
-0.859145841925031));
#79902=CARTESIAN_POINT('Ctrl Pts',(-0.138078098720645,-0.1934212305751,
-0.860794735045849));
#79903=CARTESIAN_POINT('Ctrl Pts',(-0.150040295602851,-0.184296591813715,
-0.861903131385808));
#79904=CARTESIAN_POINT('Ctrl Pts',(-0.165036758918983,-0.17042359398197,
-0.863367505551587));
#79905=CARTESIAN_POINT('Ctrl Pts',(-0.168886921020689,-0.166608976985486,
-0.863750910674673));
#79906=CARTESIAN_POINT('Ctrl Pts',(-0.173642117154723,-0.16156326864552,
-0.864230594587012));
#79907=CARTESIAN_POINT('Ctrl Pts',(-0.1746703484961,-0.160451065064583,
-0.864334705246915));
#79908=CARTESIAN_POINT('Ctrl Pts',(-0.176300314283349,-0.158653745351712,
-0.86450026108293));
#79909=CARTESIAN_POINT('Ctrl Pts',(-0.176908855424301,-0.157974898872121,
-0.864562189082302));
#79910=CARTESIAN_POINT('Ctrl Pts',(-0.17807980834442,-0.156653412680118,
-0.864681552493512));
#79911=CARTESIAN_POINT('Ctrl Pts',(-0.178642683408639,-0.156011222462758,
-0.864739019284844));
#79912=CARTESIAN_POINT('Ctrl Pts',(-0.180015346096379,-0.154427967317936,
-0.864879418477489));
#79913=CARTESIAN_POINT('Ctrl Pts',(-0.180821251566946,-0.153483540060386,
-0.864962072178599));
#79914=CARTESIAN_POINT('Ctrl Pts',(-0.183675999509331,-0.150084411941833,
-0.865255846228854));
#79915=CARTESIAN_POINT('Ctrl Pts',(-0.18568267523755,-0.147594546041182,
-0.865464203683312));
#79916=CARTESIAN_POINT('Ctrl Pts',(-0.193190259396895,-0.137883626336553,
-0.866254381989254));
#79917=CARTESIAN_POINT('Ctrl Pts',(-0.198325726549276,-0.130389060151497,
-0.866817997511125));
#79918=CARTESIAN_POINT('Ctrl Pts',(-0.209883835834251,-0.111252222847797,
-0.868194353797005));
#79919=CARTESIAN_POINT('Ctrl Pts',(-0.215781610133051,-0.099330592018818,
-0.869000276477057));
#79920=CARTESIAN_POINT('Ctrl Pts',(-0.2234437995909,-0.0798927662217952,
-0.870309197419156));
#79921=CARTESIAN_POINT('Ctrl Pts',(-0.225893669858742,-0.0726774928777872,
-0.870793708034588));
#79922=CARTESIAN_POINT('Ctrl Pts',(-0.228668639172929,-0.06299731507165,
-0.871449296863225));
#79923=CARTESIAN_POINT('Ctrl Pts',(-0.229308479676761,-0.0606269631479993,
-0.871610239816516));
#79924=CARTESIAN_POINT('Ctrl Pts',(-0.230299849166122,-0.0567138612169758,
-0.871876818091302));
#79925=CARTESIAN_POINT('Ctrl Pts',(-0.230672951872816,-0.0551767310511085,
-0.871981756396661));
#79926=CARTESIAN_POINT('Ctrl Pts',(-0.231371085821785,-0.0521696035377968,
-0.872187537240103));
#79927=CARTESIAN_POINT('Ctrl Pts',(-0.231697551301291,-0.0507000140896716,
-0.872288328384588));
#79928=CARTESIAN_POINT('Ctrl Pts',(-0.232318588727858,-0.0477730514545132,
-0.87248956036089));
#79929=CARTESIAN_POINT('Ctrl Pts',(-0.232613490476748,-0.0463158178941775,
-0.872589985581281));
#79930=CARTESIAN_POINT('Ctrl Pts',(-0.233272741333017,-0.0428929485776275,
-0.872826467599483));
#79931=CARTESIAN_POINT('Ctrl Pts',(-0.233625972873291,-0.0409253132170732,
-0.872962867722792));
#79932=CARTESIAN_POINT('Ctrl Pts',(-0.234678820381688,-0.0346019227963592,
-0.873402768668219));
#79933=CARTESIAN_POINT('Ctrl Pts',(-0.235281766051343,-0.0302312419375767,
-0.873709196959671));
#79934=CARTESIAN_POINT('Ctrl Pts',(-0.236711368924702,-0.0171909327698615,
-0.874630663518059));
#79935=CARTESIAN_POINT('Ctrl Pts',(-0.237182793595308,-0.008490628075348,
-0.875255150768821));
#79936=CARTESIAN_POINT('Ctrl Pts',(-0.237174902566701,0.000214982501742253,
-0.87588669733343));
#79937=CARTESIAN_POINT('Ctrl Pts',(-0.23717490269649,0.000214839266908004,
-0.875886686942491));
#79938=CARTESIAN_POINT('Ctrl Pts',(-0.237160436115023,0.0161854302161968,
-0.877045269750223));
#79939=CARTESIAN_POINT('Ctrl Pts',(-0.235532942994856,0.0321144320544727,
-0.878225659313285));
#79940=CARTESIAN_POINT('Ctrl Pts',(-0.231758761892673,0.0504730591886212,
-0.879551285230372));
#79941=CARTESIAN_POINT('Ctrl Pts',(-0.231153454613579,0.0531764548900551,
-0.879745483075348));
#79942=CARTESIAN_POINT('Ctrl Pts',(-0.230220788146122,0.0570244099532458,
-0.880019889551011));
#79943=CARTESIAN_POINT('Ctrl Pts',(-0.229931986411869,0.0581779716961225,
-0.880101892122108));
#79944=CARTESIAN_POINT('Ctrl Pts',(-0.229366075977925,0.060368330891023,
-0.880257038402641));
#79945=CARTESIAN_POINT('Ctrl Pts',(-0.229090583242611,0.061405512501592,
-0.880330263927035));
#79946=CARTESIAN_POINT('Ctrl Pts',(-0.228610189196349,0.0631658679588368,
-0.8804540964853));
#79947=CARTESIAN_POINT('Ctrl Pts',(-0.228408878006416,0.0638899834536621,
-0.880504903069019));
#79948=CARTESIAN_POINT('Ctrl Pts',(-0.227941147699356,0.0655419376381564,
-0.88062050309687));
#79949=CARTESIAN_POINT('Ctrl Pts',(-0.227672502856321,0.0664691201189385,
-0.880685168021568));
#79950=CARTESIAN_POINT('Ctrl Pts',(-0.226910778673012,0.0690392750089375,
-0.88086388221992));
#79951=CARTESIAN_POINT('Ctrl Pts',(-0.226405513889538,0.070678615366744,
-0.880977260760265));
#79952=CARTESIAN_POINT('Ctrl Pts',(-0.222747210813616,0.0821060711419424,
-0.88176424633515));
#79953=CARTESIAN_POINT('Ctrl Pts',(-0.218977887177857,0.0916867770309371,
-0.882407013997007));
#79954=CARTESIAN_POINT('Ctrl Pts',(-0.209255150934324,0.112346310699076,
-0.883816233200857));
#79955=CARTESIAN_POINT('Ctrl Pts',(-0.203019981926796,0.123257038955161,
-0.884577205928329));
#79956=CARTESIAN_POINT('Ctrl Pts',(-0.192492860221365,0.138694465400979,
-0.885739931034289));
#79957=CARTESIAN_POINT('Ctrl Pts',(-0.188839378594836,0.1436291651109,-0.886125945113413));
#79958=CARTESIAN_POINT('Ctrl Pts',(-0.182279144853885,0.151806399116678,
-0.886796443276678));
#79959=CARTESIAN_POINT('Ctrl Pts',(-0.179466960670738,0.155120842253829,
-0.887077525421505));
#79960=CARTESIAN_POINT('Ctrl Pts',(-0.175461992822456,0.159586343550733,
-0.887470553022884));
#79961=CARTESIAN_POINT('Ctrl Pts',(-0.174345733097042,0.160805090391318,
-0.887579355544892));
#79962=CARTESIAN_POINT('Ctrl Pts',(-0.173169647989306,0.162062513911321,
-0.88769326396694));
#79963=CARTESIAN_POINT('Ctrl Pts',(-0.173122423481623,0.16211296027101,
-0.887697836639924));
#79964=CARTESIAN_POINT('Ctrl Pts',(-0.173027224790476,0.162214564774533,
-0.887707052154992));
#79965=CARTESIAN_POINT('Ctrl Pts',(-0.172979249949819,0.162265722290524,
-0.887711695024554));
#79966=CARTESIAN_POINT('Ctrl Pts',(-0.172915833791056,0.162333285425153,
-0.88771783063105));
#79967=CARTESIAN_POINT('Ctrl Pts',(-0.172900412777663,0.16234971017496,
-0.887719322509477));
#79968=CARTESIAN_POINT('Ctrl Pts',(-0.172867231935001,0.162385040631729,
-0.887722532257328));
#79969=CARTESIAN_POINT('Ctrl Pts',(-0.172849471345733,0.162403945621211,
-0.887724250158876));
#79970=CARTESIAN_POINT('Ctrl Pts',(-0.17281112655442,0.162444747736535,
-0.88772795871381));
#79971=CARTESIAN_POINT('Ctrl Pts',(-0.172790541292811,0.162466643862455,
-0.887729949412034));
#79972=CARTESIAN_POINT('Ctrl Pts',(-0.172745919821677,0.162514088744458,
-0.887734264043252));
#79973=CARTESIAN_POINT('Ctrl Pts',(-0.172721882107559,0.162539636079017,
-0.887736588039945));
#79974=CARTESIAN_POINT('Ctrl Pts',(-0.17266952791604,0.162595253498637,
-0.8877416490409));
#79975=CARTESIAN_POINT('Ctrl Pts',(-0.172641209253794,0.162625321516726,
-0.887744386137709));
#79976=CARTESIAN_POINT('Ctrl Pts',(-0.172579175490758,0.162691152886866,
-0.887750380984973));
#79977=CARTESIAN_POINT('Ctrl Pts',(-0.172545457131033,0.16272691315257,
-0.887753638873601));
#79978=CARTESIAN_POINT('Ctrl Pts',(-0.172471073335732,0.162805752345842,
-0.88776082455701));
#79979=CARTESIAN_POINT('Ctrl Pts',(-0.172430402880675,0.162848826513648,
-0.887764752564831));
#79980=CARTESIAN_POINT('Ctrl Pts',(-0.172339891753788,0.162944615124906,
-0.887773492316094));
#79981=CARTESIAN_POINT('Ctrl Pts',(-0.172290043041345,0.162997321931075,
-0.887778304401207));
#79982=CARTESIAN_POINT('Ctrl Pts',(-0.172177856387801,0.1631158318827,-0.887789131276454));
#79983=CARTESIAN_POINT('Ctrl Pts',(-0.17211550491725,0.163181622151898,
-0.887795146642349));
#79984=CARTESIAN_POINT('Ctrl Pts',(-0.171973096879435,0.163331711832582,
-0.887808880855109));
#79985=CARTESIAN_POINT('Ctrl Pts',(-0.171893016062611,0.163415988107903,
-0.887816600735816));
#79986=CARTESIAN_POINT('Ctrl Pts',(-0.171691709049339,0.163627529960834,
-0.887835998633214));
#79987=CARTESIAN_POINT('Ctrl Pts',(-0.171570403445524,0.163754719561374,
-0.887847680043757));
#79988=CARTESIAN_POINT('Ctrl Pts',(-0.170430437871161,0.16494732264286,
-0.88795738511415));
#79989=CARTESIAN_POINT('Ctrl Pts',(-0.169402027773762,0.166003331948233,
-0.888055826389046));
#79990=CARTESIAN_POINT('Ctrl Pts',(-0.167086899056528,0.168336673984274,
-0.888276312912292));
#79991=CARTESIAN_POINT('Ctrl Pts',(-0.165795254012181,0.169608965195928,
-0.888398571983746));
#79992=CARTESIAN_POINT('Ctrl Pts',(-0.16247198856065,0.172808198930739,
-0.88871131093992));
#79993=CARTESIAN_POINT('Ctrl Pts',(-0.160420645423922,0.174714155248683,
-0.888902668918628));
#79994=CARTESIAN_POINT('Ctrl Pts',(-0.143707484802519,0.189700267806334,
-0.890449001653943));
#79995=CARTESIAN_POINT('Ctrl Pts',(-0.127508080645291,0.200946322777468,
-0.891880272615361));
#79996=CARTESIAN_POINT('Ctrl Pts',(-0.103218165637264,0.213678689250855,
-0.893880426729042));
#79997=CARTESIAN_POINT('Ctrl Pts',(-0.0961497172639372,0.216951188626471,
-0.894445892296079));
#79998=CARTESIAN_POINT('Ctrl Pts',(-0.0849671138441651,0.221474308544954,
-0.895304106626987));
#79999=CARTESIAN_POINT('Ctrl Pts',(-0.0809585001955723,0.22297086462913,
-0.895604766087735));
#80000=CARTESIAN_POINT('Ctrl Pts',(-0.0756286173282596,0.224797979357973,
-0.895993513610001));
#80001=CARTESIAN_POINT('Ctrl Pts',(-0.0743421361698405,0.225226699771743,
-0.896086513230532));
#80002=CARTESIAN_POINT('Ctrl Pts',(-0.0722175744162482,0.225914523293802,
-0.896238649657227));
#80003=CARTESIAN_POINT('Ctrl Pts',(-0.0713816274285868,0.226180046028471,
-0.89629814365353));
#80004=CARTESIAN_POINT('Ctrl Pts',(-0.0698038938496573,0.226671564795226,
-0.896409715166161));
#80005=CARTESIAN_POINT('Ctrl Pts',(-0.0690624387684199,0.226898570904394,
-0.896461852163554));
#80006=CARTESIAN_POINT('Ctrl Pts',(-0.0672955731796037,0.227430056446354,
-0.896585419587905));
#80007=CARTESIAN_POINT('Ctrl Pts',(-0.0662691794182706,0.22773124667358,
-0.89665666363972));
#80008=CARTESIAN_POINT('Ctrl Pts',(-0.0626045639227825,0.228779736020652,
-0.89690923629057));
#80009=CARTESIAN_POINT('Ctrl Pts',(-0.0599553495863132,0.229488249487896,
-0.897088521173322));
#80010=CARTESIAN_POINT('Ctrl Pts',(-0.0522100329691301,0.231416388623629,
-0.897604712859081));
#80011=CARTESIAN_POINT('Ctrl Pts',(-0.0470876893284127,0.232512641753263,
-0.897936157593881));
#80012=CARTESIAN_POINT('Ctrl Pts',(-0.0419358085112875,0.233438147245699,
-0.898263402204347));
#80013=CARTESIAN_POINT('',(-0.237254449915977,-6.65203262155088E-5,-0.895658993950963));
#80014=CARTESIAN_POINT('Ctrl Pts',(-0.0419358257166344,0.233438144154858,
-0.917832673049623));
#80015=CARTESIAN_POINT('Ctrl Pts',(-0.0558504293696778,0.230938465296363,
-0.916886800148356));
#80016=CARTESIAN_POINT('Ctrl Pts',(-0.0695352643872399,0.227191402517845,
-0.915940927247089));
#80017=CARTESIAN_POINT('Ctrl Pts',(-0.0827588563410773,0.222267749172292,
-0.914995054345823));
#80018=CARTESIAN_POINT('Ctrl Pts',(-0.0960128478354698,0.217332776905218,
-0.91404700698986));
#80019=CARTESIAN_POINT('Ctrl Pts',(-0.108802715093054,0.211216154142449,
-0.913098959633897));
#80020=CARTESIAN_POINT('Ctrl Pts',(-0.120917503389532,0.204036609457819,
-0.912150912277934));
#80021=CARTESIAN_POINT('Ctrl Pts',(-0.126787381578739,0.20055796404352,
-0.911691562732493));
#80022=CARTESIAN_POINT('Ctrl Pts',(-0.132499180445869,0.196830462375787,
-0.911232213187052));
#80023=CARTESIAN_POINT('Ctrl Pts',(-0.138031530126742,0.192871141739428,
-0.910772863641611));
#80024=CARTESIAN_POINT('Ctrl Pts',(-0.149367873262532,0.184758093955488,
-0.909831610039296));
#80025=CARTESIAN_POINT('Ctrl Pts',(-0.160027179815794,0.175612883814287,
-0.908890356436981));
#80026=CARTESIAN_POINT('Ctrl Pts',(-0.169815694091736,0.165573580818746,
-0.907949102834666));
#80027=CARTESIAN_POINT('Ctrl Pts',(-0.17958447881759,0.155554512858444,
-0.907009746405872));
#80028=CARTESIAN_POINT('Ctrl Pts',(-0.188485316369692,0.144645477147395,
-0.906070389977077));
#80029=CARTESIAN_POINT('Ctrl Pts',(-0.196358430816218,0.133023859786102,
-0.905131033548283));
#80030=CARTESIAN_POINT('Ctrl Pts',(-0.204230121710632,0.121404343750536,
-0.90419184696623));
#80031=CARTESIAN_POINT('Ctrl Pts',(-0.211073945122252,0.109073175716272,
-0.903252660384176));
#80032=CARTESIAN_POINT('Ctrl Pts',(-0.216771925601164,0.0962388325789722,
-0.902313473802122));
#80033=CARTESIAN_POINT('Ctrl Pts',(-0.222469382240046,0.0834056693584373,
-0.901374373563559));
#80034=CARTESIAN_POINT('Ctrl Pts',(-0.227020883339142,0.0700702071992786,
-0.900435273324997));
#80035=CARTESIAN_POINT('Ctrl Pts',(-0.230356521300201,0.0564610814585572,
-0.899496173086434));
#80036=CARTESIAN_POINT('Ctrl Pts',(-0.233699367139866,0.0428225481719909,
-0.898555043574732));
#80037=CARTESIAN_POINT('Ctrl Pts',(-0.235820962713621,0.0289100078227147,
-0.897613914063031));
#80038=CARTESIAN_POINT('Ctrl Pts',(-0.236702619460895,0.0149616364529731,
-0.896672784551329));
#80039=CARTESIAN_POINT('Ctrl Pts',(-0.237019194434059,0.00995321871475168,
-0.896334854794841));
#80040=CARTESIAN_POINT('Ctrl Pts',(-0.237176394014881,0.00494019484129286,
-0.895996925038354));
#80041=CARTESIAN_POINT('Ctrl Pts',(-0.237174990683324,-6.64783058782736E-5,
-0.895658995281866));
#80042=CARTESIAN_POINT('Ctrl Pts',(-0.237538664790808,-6.66706272502535E-5,
-0.895658989190502));
#80043=CARTESIAN_POINT('Ctrl Pts',(-0.237552354346597,-0.00372902877874097,
-0.895412173874543));
#80044=CARTESIAN_POINT('Ctrl Pts',(-0.235817901732334,-0.0857960183084813,
-0.889880585092257));
#80045=CARTESIAN_POINT('Ctrl Pts',(-0.141192310182904,-0.242020628383875,
-0.879064222843641));
#80046=CARTESIAN_POINT('Ctrl Pts',(0.126406588917608,-0.25006124709024,
-0.863209902444656));
#80047=CARTESIAN_POINT('Ctrl Pts',(0.278604525080261,-0.029812273024942,
-0.847355582045672));
#80048=CARTESIAN_POINT('Ctrl Pts',(0.181168188818849,0.206234623149449,
-0.832232823074446));
#80049=CARTESIAN_POINT('Ctrl Pts',(0.0247392917291787,0.245026920599375,
-0.82239483756955));
#80050=CARTESIAN_POINT('Ctrl Pts',(-0.0419725940269774,0.233652521193878,
-0.817841625530982));
#80051=CARTESIAN_POINT('Origin',(0.,0.,-1.7456589891905));
#80052=CARTESIAN_POINT('',(-0.0419358257124846,0.233438144155603,-0.697888113229229));
#80053=CARTESIAN_POINT('',(-0.0419358371735614,0.233438142096686,-0.71773215975824));
#80054=CARTESIAN_POINT('',(-0.0419358257166344,0.233438144154858,-1.7456589891905));
#80055=CARTESIAN_POINT('Ctrl Pts',(-0.0419358257124646,0.233438144155607,
-0.69788811322923));
#80056=CARTESIAN_POINT('Ctrl Pts',(-0.0412725130934422,0.233557304468866,
-0.69793329997025));
#80057=CARTESIAN_POINT('Ctrl Pts',(-0.0406086977456027,0.233673636659218,
-0.697978576320819));
#80058=CARTESIAN_POINT('Ctrl Pts',(-0.0377982973546973,0.234153815987307,
-0.698170504273831));
#80059=CARTESIAN_POINT('Ctrl Pts',(-0.0356473144743005,0.234490915060856,
-0.698317994985194));
#80060=CARTESIAN_POINT('Ctrl Pts',(-0.0281718628651947,0.235557226866814,
-0.698832794847702));
#80061=CARTESIAN_POINT('Ctrl Pts',(-0.0228278158251959,0.236135011834267,
-0.699204746382527));
#80062=CARTESIAN_POINT('Ctrl Pts',(-0.000445459285731659,0.237788072973295,
-0.700779755513132));
#80063=CARTESIAN_POINT('Ctrl Pts',(0.0166622754813853,0.237203667853011,
-0.702029844000345));
#80064=CARTESIAN_POINT('Ctrl Pts',(0.0405931708206377,0.233783461845906,
-0.703790846568692));
#80065=CARTESIAN_POINT('Ctrl Pts',(0.0475819246709634,0.232461793583376,
-0.704305869388053));
#80066=CARTESIAN_POINT('Ctrl Pts',(0.0571675330652086,0.230198522675884,
-0.705005415207937));
#80067=CARTESIAN_POINT('Ctrl Pts',(0.0598229510699037,0.229522771377182,
-0.705198447491975));
#80068=CARTESIAN_POINT('Ctrl Pts',(0.0644447600567318,0.228260947380078,
-0.705532435567961));
#80069=CARTESIAN_POINT('Ctrl Pts',(0.0664163334730075,0.227695099974509,
-0.705674267603045));
#80070=CARTESIAN_POINT('Ctrl Pts',(0.0693612119259817,0.226808403973138,
-0.70588490445148));
#80071=CARTESIAN_POINT('Ctrl Pts',(0.0703401242585132,0.226506725838501,
-0.705954719961399));
#80072=CARTESIAN_POINT('Ctrl Pts',(0.0721083366194157,0.225949234892154,
-0.706080422039977));
#80073=CARTESIAN_POINT('Ctrl Pts',(0.072898273271877,0.225695615293672,
-0.706136427678752));
#80074=CARTESIAN_POINT('Ctrl Pts',(0.0746798392025913,0.225113290362607,
-0.706262403854519));
#80075=CARTESIAN_POINT('Ctrl Pts',(0.075670643568685,0.224782173861577,
-0.706332234169308));
#80076=CARTESIAN_POINT('Ctrl Pts',(0.0786987506030232,0.223747920836769,
-0.706545036710449));
#80077=CARTESIAN_POINT('Ctrl Pts',(0.0807287486399363,0.223023530972261,
-0.706686841963383));
#80078=CARTESIAN_POINT('Ctrl Pts',(0.0970899928584773,0.216932461884938,
-0.707824970126772));
#80079=CARTESIAN_POINT('Ctrl Pts',(0.110882979325758,0.210217160741557,
-0.708756077641373));
#80080=CARTESIAN_POINT('Ctrl Pts',(0.137195436773496,0.194090992522556,
-0.710648992683725));
#80081=CARTESIAN_POINT('Ctrl Pts',(0.149623442868847,0.184679837298448,
-0.711607558388222));
#80082=CARTESIAN_POINT('Ctrl Pts',(0.163093244088333,0.172221935031071,
-0.7127975238538));
#80083=CARTESIAN_POINT('Ctrl Pts',(0.165112479337283,0.170287020256893,
-0.712980309158533));
#80084=CARTESIAN_POINT('Ctrl Pts',(0.168270974463446,0.167151417801917,
-0.713273657640761));
#80085=CARTESIAN_POINT('Ctrl Pts',(0.169432733221153,0.165973690686213,
-0.713383219847253));
#80086=CARTESIAN_POINT('Ctrl Pts',(0.171611135338577,0.163718638867498,
-0.713591906253986));
#80087=CARTESIAN_POINT('Ctrl Pts',(0.172630195928064,0.162643751087149,
-0.713690918537525));
#80088=CARTESIAN_POINT('Ctrl Pts',(0.17493119070244,0.160170712417427,-0.71391772663532));
#80089=CARTESIAN_POINT('Ctrl Pts',(0.176206539543232,0.158766601198959,
-0.714045792985131));
#80090=CARTESIAN_POINT('Ctrl Pts',(0.17951259201194,0.15503785653193,-0.714384131193657));
#80091=CARTESIAN_POINT('Ctrl Pts',(0.181514938595392,0.152688680535317,
-0.714595545447361));
#80092=CARTESIAN_POINT('Ctrl Pts',(0.193888879589917,0.137583964803688,
-0.715944562212651));
#80093=CARTESIAN_POINT('Ctrl Pts',(0.202954760662182,0.123820158254631,
-0.717132842792232));
#80094=CARTESIAN_POINT('Ctrl Pts',(0.216812064825179,0.097113011537336,
-0.7193289511933));
#80095=CARTESIAN_POINT('Ctrl Pts',(0.222042744192121,0.0844718863378857,
-0.720327920555699));
#80096=CARTESIAN_POINT('Ctrl Pts',(0.226743498802375,0.0695928095778601,
-0.721414273719591));
#80097=CARTESIAN_POINT('Ctrl Pts',(0.22730732017159,0.067728547901772,-0.721548810022305));
#80098=CARTESIAN_POINT('Ctrl Pts',(0.228126802174816,0.0648933733869678,
-0.721750815913295));
#80099=CARTESIAN_POINT('Ctrl Pts',(0.228399352843517,0.0639274862112577,
-0.721819181754972));
#80100=CARTESIAN_POINT('Ctrl Pts',(0.228886252368911,0.0621591019328021,
-0.721943484782441));
#80101=CARTESIAN_POINT('Ctrl Pts',(0.229102521954586,0.0613571915278185,
-0.721999525647994));
#80102=CARTESIAN_POINT('Ctrl Pts',(0.229587383506215,0.0595210518266504,
-0.722127107771786));
#80103=CARTESIAN_POINT('Ctrl Pts',(0.229853204084155,0.0584861261977165,
-0.722198491767631));
#80104=CARTESIAN_POINT('Ctrl Pts',(0.230664600932059,0.0552360987627232,
-0.722421116651515));
#80105=CARTESIAN_POINT('Ctrl Pts',(0.231185237300466,0.0530148254907443,
-0.722571029091603));
#80106=CARTESIAN_POINT('Ctrl Pts',(0.234427060631319,0.0382264749576697,
-0.723556356512882));
#80107=CARTESIAN_POINT('Ctrl Pts',(0.236154792639585,0.0254618914173424,
-0.724346825836072));
#80108=CARTESIAN_POINT('Ctrl Pts',(0.237154285285275,0.00670265809831208,
-0.725499371379098));
#80109=CARTESIAN_POINT('Ctrl Pts',(0.237247710422204,0.000776829243992221,
-0.725862000528685));
#80110=CARTESIAN_POINT('Ctrl Pts',(0.23694500390142,-0.0131708122621528,
-0.726722141205528));
#80111=CARTESIAN_POINT('Ctrl Pts',(0.236363617371624,-0.0211809168341281,
-0.727221406317558));
#80112=CARTESIAN_POINT('Ctrl Pts',(0.234727607699095,-0.0343931519318241,
-0.728067359657244));
#80113=CARTESIAN_POINT('Ctrl Pts',(0.233902584853899,-0.0396170787934021,
-0.72840768701051));
#80114=CARTESIAN_POINT('Ctrl Pts',(0.23250614692182,-0.0468753790175062,
-0.728891052473623));
#80115=CARTESIAN_POINT('Ctrl Pts',(0.232081073999932,-0.0489365317085573,
-0.729029505816284));
#80116=CARTESIAN_POINT('Ctrl Pts',(0.231303508083531,-0.0524686071292961,
-0.729268949468528));
#80117=CARTESIAN_POINT('Ctrl Pts',(0.230964264410336,-0.0539423393184799,
-0.729369513516864));
#80118=CARTESIAN_POINT('Ctrl Pts',(0.230244226842506,-0.05693891877784,
-0.729575384869119));
#80119=CARTESIAN_POINT('Ctrl Pts',(0.229862362327056,-0.0584614287091833,
-0.729680722025409));
#80120=CARTESIAN_POINT('Ctrl Pts',(0.22885917611664,-0.0622993167888613,
-0.729948175063598));
#80121=CARTESIAN_POINT('Ctrl Pts',(0.228217822408551,-0.064609226644583,
-0.730110927716206));
#80122=CARTESIAN_POINT('Ctrl Pts',(0.225544880266468,-0.0736992740187871,
-0.730758682700036));
#80123=CARTESIAN_POINT('Ctrl Pts',(0.223245419651537,-0.0803961492509822,
-0.731252187816021));
#80124=CARTESIAN_POINT('Ctrl Pts',(0.214960011534496,-0.10141459503311,
-0.732854003245396));
#80125=CARTESIAN_POINT('Ctrl Pts',(0.207867439663697,-0.115255197440044,
-0.733992714310863));
#80126=CARTESIAN_POINT('Ctrl Pts',(0.195866530126652,-0.133913372891324,
-0.735607075104717));
#80127=CARTESIAN_POINT('Ctrl Pts',(0.192022152731297,-0.139369986256464,
-0.736089517425925));
#80128=CARTESIAN_POINT('Ctrl Pts',(0.186346247045105,-0.146744653083869,
-0.736749688956695));
#80129=CARTESIAN_POINT('Ctrl Pts',(0.184705177473427,-0.14880495842335,
-0.736935051888818));
#80130=CARTESIAN_POINT('Ctrl Pts',(0.181764392455744,-0.152373379639254,
-0.737257156581974));
#80131=CARTESIAN_POINT('Ctrl Pts',(0.180479393967894,-0.153893242832383,
-0.737394695947567));
#80132=CARTESIAN_POINT('Ctrl Pts',(0.17851218865146,-0.156161466525623,
-0.737600260082383));
#80133=CARTESIAN_POINT('Ctrl Pts',(0.177844108671842,-0.1569218857589,-0.737669227495669));
#80134=CARTESIAN_POINT('Ctrl Pts',(0.1766193214997,-0.1582980887841,-0.737794102894248));
#80135=CARTESIAN_POINT('Ctrl Pts',(0.176064236033842,-0.158915243053559,
-0.73785012097879));
#80136=CARTESIAN_POINT('Ctrl Pts',(0.174794150653348,-0.160312523602193,
-0.737977000538946));
#80137=CARTESIAN_POINT('Ctrl Pts',(0.174077158499177,-0.161090792169538,
-0.738047712102788));
#80138=CARTESIAN_POINT('Ctrl Pts',(0.171835681275349,-0.163491391400436,
-0.738266051820637));
#80139=CARTESIAN_POINT('Ctrl Pts',(0.170293497032524,-0.165097129488348,
-0.738412423267754));
#80140=CARTESIAN_POINT('Ctrl Pts',(0.158647759741697,-0.17688594891788,
-0.739491693605409));
#80141=CARTESIAN_POINT('Ctrl Pts',(0.147660216672685,-0.186156711101084,
-0.740367942588498));
#80142=CARTESIAN_POINT('Ctrl Pts',(0.122471100144973,-0.203767829853502,
-0.742252702928717));
#80143=CARTESIAN_POINT('Ctrl Pts',(0.108106343461762,-0.211739056874006,
-0.743259151887015));
#80144=CARTESIAN_POINT('Ctrl Pts',(0.0904553046373063,-0.219266248232256,
-0.744503574079788));
#80145=CARTESIAN_POINT('Ctrl Pts',(0.0878557140438428,-0.220320725713338,
-0.744686913416427));
#80146=CARTESIAN_POINT('Ctrl Pts',(0.0836926301445601,-0.221924011954446,
-0.744980942043255));
#80147=CARTESIAN_POINT('Ctrl Pts',(0.082140983340077,-0.222502993337991,
-0.74509062208691));
#80148=CARTESIAN_POINT('Ctrl Pts',(0.079190711674247,-0.223568791690181,
-0.745299400619212));
#80149=CARTESIAN_POINT('Ctrl Pts',(0.0777933370708359,-0.224058853808182,
-0.74539838578155));
#80150=CARTESIAN_POINT('Ctrl Pts',(0.0745988010599739,-0.225145697791662,
-0.745624945197424));
#80151=CARTESIAN_POINT('Ctrl Pts',(0.0727989170514584,-0.225734099481807,
-0.745752787798189));
#80152=CARTESIAN_POINT('Ctrl Pts',(0.068057861652633,-0.227221402946516,
-0.746090126726254));
#80153=CARTESIAN_POINT('Ctrl Pts',(0.0651059974755016,-0.228084734357983,
-0.746300754531325));
#80154=CARTESIAN_POINT('Ctrl Pts',(0.0460115203232367,-0.233268430733042,
-0.747667549970748));
#80155=CARTESIAN_POINT('Ctrl Pts',(0.0294699329641209,-0.235929135672803,
-0.748876284902607));
#80156=CARTESIAN_POINT('Ctrl Pts',(-0.000450035284266839,-0.237544880996643,
-0.751063461568662));
#80157=CARTESIAN_POINT('Ctrl Pts',(-0.013727327331866,-0.237148477525913,
-0.752032725103823));
#80158=CARTESIAN_POINT('Ctrl Pts',(-0.0289269556793946,-0.235413172793825,
-0.753099022095125));
#80159=CARTESIAN_POINT('Ctrl Pts',(-0.0309480029171191,-0.235156017355622,
-0.753239879208319));
#80160=CARTESIAN_POINT('Ctrl Pts',(-0.0339772225012229,-0.2347308513634,
-0.753449365379745));
#80161=CARTESIAN_POINT('Ctrl Pts',(-0.0349879725537008,-0.234582322660133,
-0.753518989499361));
#80162=CARTESIAN_POINT('Ctrl Pts',(-0.0368178645813363,-0.234301331434553,
-0.753644503126043));
#80163=CARTESIAN_POINT('Ctrl Pts',(-0.0376372954166165,-0.234171097933388,
-0.75370050968628));
#80164=CARTESIAN_POINT('Ctrl Pts',(-0.0394897921660676,-0.233866702156411,
-0.753826681377299));
#80165=CARTESIAN_POINT('Ctrl Pts',(-0.0405224042354136,-0.233689993199257,
-0.753896704163329));
#80166=CARTESIAN_POINT('Ctrl Pts',(-0.0436908304922455,-0.233126153236949,
-0.754110708647462));
#80167=CARTESIAN_POINT('Ctrl Pts',(-0.0458225967628157,-0.232716528062168,
-0.754253504176947));
#80168=CARTESIAN_POINT('Ctrl Pts',(-0.0626830524583758,-0.229236064178477,
-0.755375602730882));
#80169=CARTESIAN_POINT('Ctrl Pts',(-0.0770968331509615,-0.224798890260848,
-0.756292022945539));
#80170=CARTESIAN_POINT('Ctrl Pts',(-0.0953643953620943,-0.217209587021275,
-0.757505226182876));
#80171=CARTESIAN_POINT('Ctrl Pts',(-0.0996789223548126,-0.21526375420334,
-0.757795655804547));
#80172=CARTESIAN_POINT('Ctrl Pts',(-0.114093881390425,-0.208236321503507,
-0.758786382857383));
#80173=CARTESIAN_POINT('Ctrl Pts',(-0.123887091487939,-0.202562881419221,
-0.759495123866013));
#80174=CARTESIAN_POINT('Ctrl Pts',(-0.135438908112064,-0.194718673629606,
-0.760402061029963));
#80175=CARTESIAN_POINT('Ctrl Pts',(-0.137614665101858,-0.193187118388579,
-0.760576160564215));
#80176=CARTESIAN_POINT('Ctrl Pts',(-0.141077287895743,-0.190661535795931,
-0.760858848743168));
#80177=CARTESIAN_POINT('Ctrl Pts',(-0.142380539295186,-0.189690284939572,
-0.760966562446334));
#80178=CARTESIAN_POINT('Ctrl Pts',(-0.144857710766146,-0.187804256751526,
-0.761173901067231));
#80179=CARTESIAN_POINT('Ctrl Pts',(-0.14603320861826,-0.186891671910509,
-0.761273436860246));
#80180=CARTESIAN_POINT('Ctrl Pts',(-0.148705600975533,-0.184776383337047,
-0.761502414107902));
#80181=CARTESIAN_POINT('Ctrl Pts',(-0.150196616516627,-0.183566455571589,
-0.761632139405864));
#80182=CARTESIAN_POINT('Ctrl Pts',(-0.15495227656492,-0.179610606194345,
-0.762052423205687));
#80183=CARTESIAN_POINT('Ctrl Pts',(-0.158157421693699,-0.176794806959135,
-0.762345786150206));
#80184=CARTESIAN_POINT('Ctrl Pts',(-0.174700717364953,-0.161451109919493,
-0.763915565279011));
#80185=CARTESIAN_POINT('Ctrl Pts',(-0.186629735940235,-0.147498905900202,
-0.76525254706866));
#80186=CARTESIAN_POINT('Ctrl Pts',(-0.202395590662303,-0.124045783968887,
-0.767312497208922));
#80187=CARTESIAN_POINT('Ctrl Pts',(-0.20742993936851,-0.11543045729609,
-0.768034470365256));
#80188=CARTESIAN_POINT('Ctrl Pts',(-0.212932754758037,-0.104483649791722,
-0.768890955541647));
#80189=CARTESIAN_POINT('Ctrl Pts',(-0.213928520410646,-0.102429391454638,
-0.769049149074406));
#80190=CARTESIAN_POINT('Ctrl Pts',(-0.215346756242341,-0.09939264262794,
-0.769278974305295));
#80191=CARTESIAN_POINT('Ctrl Pts',(-0.21579245643712,-0.0984212308811093,
-0.769351894779467));
#80192=CARTESIAN_POINT('Ctrl Pts',(-0.216540175153328,-0.0967620652989943,
-0.76947538770417));
#80193=CARTESIAN_POINT('Ctrl Pts',(-0.216845512364745,-0.0960758479588558,
-0.769526156731377));
#80194=CARTESIAN_POINT('Ctrl Pts',(-0.217537019213532,-0.0945016583608133,
-0.769641915119431));
#80195=CARTESIAN_POINT('Ctrl Pts',(-0.217921016690719,-0.0936127594339133,
-0.769706773694072));
#80196=CARTESIAN_POINT('Ctrl Pts',(-0.218975374785192,-0.0911304238207894,
-0.769886557328217));
#80197=CARTESIAN_POINT('Ctrl Pts',(-0.219633790319206,-0.0895319355612892,
-0.77000079869276));
#80198=CARTESIAN_POINT('Ctrl Pts',(-0.22460517327538,-0.0770775342941728,
-0.770880156858521));
#80199=CARTESIAN_POINT('Ctrl Pts',(-0.22812886775872,-0.0659220982807263,
-0.771605297876332));
#80200=CARTESIAN_POINT('Ctrl Pts',(-0.233916099083184,-0.0414351821100818,
-0.773153112735934));
#80201=CARTESIAN_POINT('Ctrl Pts',(-0.235892217846397,-0.0280795464162583,
-0.773971664702166));
#80202=CARTESIAN_POINT('Ctrl Pts',(-0.237022625879822,-0.00978702504729879,
-0.775122709844574));
#80203=CARTESIAN_POINT('Ctrl Pts',(-0.237173198549217,-0.00493765826265566,
-0.775430490916757));
#80204=CARTESIAN_POINT('Ctrl Pts',(-0.237176321307005,0.00354594764316934,
-0.77597615790983));
#80205=CARTESIAN_POINT('Ctrl Pts',(-0.237094172917024,0.00717858131304308,
-0.776212119449384));
#80206=CARTESIAN_POINT('Ctrl Pts',(-0.236844378892338,0.0126545945124642,
-0.776572023971867));
#80207=CARTESIAN_POINT('Ctrl Pts',(-0.236738543718849,0.0145003507130851,
-0.776694054263467));
#80208=CARTESIAN_POINT('Ctrl Pts',(-0.236509392449921,0.0178176308153644,
-0.776914757519388));
#80209=CARTESIAN_POINT('Ctrl Pts',(-0.23639389035667,0.01928961167207,-0.777013181726927));
#80210=CARTESIAN_POINT('Ctrl Pts',(-0.236117235945196,0.0224380909768913,
-0.77722480229707));
#80211=CARTESIAN_POINT('Ctrl Pts',(-0.235951955408882,0.024114135323785,
-0.777338122733985));
#80212=CARTESIAN_POINT('Ctrl Pts',(-0.235449435426202,0.0287084214039525,
-0.777650652975377));
#80213=CARTESIAN_POINT('Ctrl Pts',(-0.235075815729186,0.031622296198115,
-0.777850986499745));
#80214=CARTESIAN_POINT('Ctrl Pts',(-0.23239536169275,0.0498381481449627,
-0.779117175203863));
#80215=CARTESIAN_POINT('Ctrl Pts',(-0.228650028799432,0.0648879872156889,
-0.780228297654479));
#80216=CARTESIAN_POINT('Ctrl Pts',(-0.218405834054344,0.0936967215075056,
-0.78245693669531));
#80217=CARTESIAN_POINT('Ctrl Pts',(-0.211995954671028,0.107414938899316,
-0.78356799163188));
#80218=CARTESIAN_POINT('Ctrl Pts',(-0.2032236080024,0.122298174456709,-0.784774058630043));
#80219=CARTESIAN_POINT('Ctrl Pts',(-0.202097460001408,0.124150295255836,
-0.784924108303636));
#80220=CARTESIAN_POINT('Ctrl Pts',(-0.200389876753717,0.126873851099288,
-0.785144411453641));
#80221=CARTESIAN_POINT('Ctrl Pts',(-0.199827841005109,0.127757234087742,
-0.785215811599965));
#80222=CARTESIAN_POINT('Ctrl Pts',(-0.198809953066832,0.129333953760501,
-0.785343111757685));
#80223=CARTESIAN_POINT('Ctrl Pts',(-0.198356294400421,0.130028649017712,
-0.785399147393608));
#80224=CARTESIAN_POINT('Ctrl Pts',(-0.197335623114046,0.131573847006154,
-0.7855236712991));
#80225=CARTESIAN_POINT('Ctrl Pts',(-0.19676674965107,0.132423078405076,
-0.785592035657926));
#80226=CARTESIAN_POINT('Ctrl Pts',(-0.19504613101071,0.134956099842965,
-0.785795813032913));
#80227=CARTESIAN_POINT('Ctrl Pts',(-0.193878100474194,0.136628785209857,
-0.785930198237594));
#80228=CARTESIAN_POINT('Ctrl Pts',(-0.184799900621261,0.149278382478264,
-0.786946831425683));
#80229=CARTESIAN_POINT('Ctrl Pts',(-0.175983970036034,0.159576878659336,
-0.787777426648224));
#80230=CARTESIAN_POINT('Ctrl Pts',(-0.154639014385431,0.180576965926637,
-0.789614163443029));
#80231=CARTESIAN_POINT('Ctrl Pts',(-0.14177996248732,0.190839287104341,
-0.790617268570057));
#80232=CARTESIAN_POINT('Ctrl Pts',(-0.125365621644718,0.20135783012493,
-0.79187398431795));
#80233=CARTESIAN_POINT('Ctrl Pts',(-0.122733673070178,0.202972803435727,
-0.792074691715093));
#80234=CARTESIAN_POINT('Ctrl Pts',(-0.118434953456661,0.205496330072761,
-0.792401696018708));
#80235=CARTESIAN_POINT('Ctrl Pts',(-0.116787441787272,0.206437092032937,
-0.792526834378161));
#80236=CARTESIAN_POINT('Ctrl Pts',(-0.113833868078978,0.208076969109135,
-0.792750939416655));
#80237=CARTESIAN_POINT('Ctrl Pts',(-0.112532194435493,0.208783810773455,
-0.792849624430142));
#80238=CARTESIAN_POINT('Ctrl Pts',(-0.109763066733463,0.210254098341952,
-0.793059438338978));
#80239=CARTESIAN_POINT('Ctrl Pts',(-0.108294081455782,0.211014474314036,
-0.793170668878473));
#80240=CARTESIAN_POINT('Ctrl Pts',(-0.104321243936692,0.213018483310317,
-0.793471359079341));
#80241=CARTESIAN_POINT('Ctrl Pts',(-0.101803224320464,0.214233280622895,
-0.793661804240626));
#80242=CARTESIAN_POINT('Ctrl Pts',(-0.0851960266152346,0.221886385936839,
-0.794917486609948));
#80243=CARTESIAN_POINT('Ctrl Pts',(-0.0705288967850475,0.22697454678074,
-0.796028446405133));
#80244=CARTESIAN_POINT('Ctrl Pts',(-0.0509872451510689,0.23167557173731,
-0.797493011601209));
#80245=CARTESIAN_POINT('Ctrl Pts',(-0.0464728068161583,0.232623102023117,
-0.797830002151534));
#80246=CARTESIAN_POINT('Ctrl Pts',(-0.0419357988072473,0.233438148988973,
-0.798166224572096));
#80247=CARTESIAN_POINT('',(-0.237109827361837,0.000214302678508487,-0.79565902906244));
#80248=CARTESIAN_POINT('Ctrl Pts',(-0.0419725940269774,0.233652521193878,
-0.817841625530982));
#80249=CARTESIAN_POINT('Ctrl Pts',(-0.052691146551867,0.231825004311616,
-0.817110064103221));
#80250=CARTESIAN_POINT('Ctrl Pts',(-0.139632908759117,0.210569229449833,
-0.811093729209133));
#80251=CARTESIAN_POINT('Ctrl Pts',(-0.22545258634803,0.119877253208548,
-0.803699530386285));
#80252=CARTESIAN_POINT('Ctrl Pts',(-0.237291832349283,0.0207557962214839,
-0.797036892991199));
#80253=CARTESIAN_POINT('Ctrl Pts',(-0.237109827361837,0.000214302678508487,
-0.79565902906244));
#80254=CARTESIAN_POINT('Ctrl Pts',(-0.237174905727117,0.000211467096690729,
-0.795696433125957));
#80255=CARTESIAN_POINT('Ctrl Pts',(-0.237183570743107,-0.00950694481013415,
-0.795099524121233));
#80256=CARTESIAN_POINT('Ctrl Pts',(-0.236594901708461,-0.0192163662911197,
-0.794499015434566));
#80257=CARTESIAN_POINT('Ctrl Pts',(-0.234853264355434,-0.0334220249162563,
-0.793591602292384));
#80258=CARTESIAN_POINT('Ctrl Pts',(-0.234161842675524,-0.0379646516319011,
-0.793297117129415));
#80259=CARTESIAN_POINT('Ctrl Pts',(-0.232991163280162,-0.0443944688046205,
-0.792872515283452));
#80260=CARTESIAN_POINT('Ctrl Pts',(-0.232619907358163,-0.0463004251536392,
-0.792745675415652));
#80261=CARTESIAN_POINT('Ctrl Pts',(-0.231927291970332,-0.0496373047693558,
-0.792521771257462));
#80262=CARTESIAN_POINT('Ctrl Pts',(-0.231615981515141,-0.0510702235320288,
-0.792425024249665));
#80263=CARTESIAN_POINT('Ctrl Pts',(-0.230960616551684,-0.0539574595370931,
-0.792228824920733));
#80264=CARTESIAN_POINT('Ctrl Pts',(-0.230616063924194,-0.0554115937654241,
-0.792129360808724));
#80265=CARTESIAN_POINT('Ctrl Pts',(-0.229873022859243,-0.0584204565614054,
-0.791922154891479));
#80266=CARTESIAN_POINT('Ctrl Pts',(-0.229472449671661,-0.0599745863349541,
-0.791814350645875));
#80267=CARTESIAN_POINT('Ctrl Pts',(-0.22839047461548,-0.0640027871121505,
-0.791532841402084));
#80268=CARTESIAN_POINT('Ctrl Pts',(-0.227684652809592,-0.0664700205364123,
-0.791358358494667));
#80269=CARTESIAN_POINT('Ctrl Pts',(-0.224384687695233,-0.077335281477275,
-0.790580521099673));
#80270=CARTESIAN_POINT('Ctrl Pts',(-0.221365207361706,-0.0855958276906676,
-0.78996362248931));
#80271=CARTESIAN_POINT('Ctrl Pts',(-0.21191323810314,-0.107583193448354,
-0.788252258217256));
#80272=CARTESIAN_POINT('Ctrl Pts',(-0.204612912815062,-0.120891934098815,
-0.787136939922067));
#80273=CARTESIAN_POINT('Ctrl Pts',(-0.191659696691151,-0.139931064890045,
-0.785467694818033));
#80274=CARTESIAN_POINT('Ctrl Pts',(-0.186901989987256,-0.146225215028108,
-0.784902570338719));
#80275=CARTESIAN_POINT('Ctrl Pts',(-0.18070583495538,-0.153624534668491,
-0.784231721414135));
#80276=CARTESIAN_POINT('Ctrl Pts',(-0.179557446660631,-0.154965222698083,
-0.784109900299498));
#80277=CARTESIAN_POINT('Ctrl Pts',(-0.177735861010109,-0.157044395839245,
-0.783920717238714));
#80278=CARTESIAN_POINT('Ctrl Pts',(-0.177072810544419,-0.157791629723499,
-0.783852673171487));
#80279=CARTESIAN_POINT('Ctrl Pts',(-0.175849814478085,-0.159152484582014,
-0.783728689310069));
#80280=CARTESIAN_POINT('Ctrl Pts',(-0.175291355754397,-0.159767365998479,
-0.783672649127169));
#80281=CARTESIAN_POINT('Ctrl Pts',(-0.174003716286925,-0.161170220039398,
-0.783544734773989));
#80282=CARTESIAN_POINT('Ctrl Pts',(-0.173272403664542,-0.16195618959638,
-0.783473021590144));
#80283=CARTESIAN_POINT('Ctrl Pts',(-0.17100674495327,-0.164358265995882,
-0.783253603660484));
#80284=CARTESIAN_POINT('Ctrl Pts',(-0.169454889654996,-0.165957788812911,
-0.78310714472481));
#80285=CARTESIAN_POINT('Ctrl Pts',(-0.158274679900464,-0.177161047115611,
-0.782076702621502));
#80286=CARTESIAN_POINT('Ctrl Pts',(-0.147857320472774,-0.185944131613457,
-0.781243350392742));
#80287=CARTESIAN_POINT('Ctrl Pts',(-0.127351052415479,-0.200414141010939,
-0.779704140511035));
#80288=CARTESIAN_POINT('Ctrl Pts',(-0.117489796512099,-0.206349810329616,
-0.779000549495292));
#80289=CARTESIAN_POINT('Ctrl Pts',(-0.101318976654128,-0.214547146283394,
-0.777858103836911));
#80290=CARTESIAN_POINT('Ctrl Pts',(-0.0952774781192003,-0.217297498570509,
-0.777433781701499));
#80291=CARTESIAN_POINT('Ctrl Pts',(-0.0870150278964188,-0.220648066866,
-0.77685209289067));
#80292=CARTESIAN_POINT('Ctrl Pts',(-0.0848888392242636,-0.221474758996812,
-0.776702299506462));
#80293=CARTESIAN_POINT('Ctrl Pts',(-0.0813026221925531,-0.222809903727811,
-0.776449297925693));
#80294=CARTESIAN_POINT('Ctrl Pts',(-0.0798489213170164,-0.223334993109952,
-0.776346647789129));
#80295=CARTESIAN_POINT('Ctrl Pts',(-0.0769638557515132,-0.224345335497279,
-0.776142688458797));
#80296=CARTESIAN_POINT('Ctrl Pts',(-0.0755327782592826,-0.224831189734997,
-0.776041404801921));
#80297=CARTESIAN_POINT('Ctrl Pts',(-0.0723520621148056,-0.225877255555812,
-0.775815995957368));
#80298=CARTESIAN_POINT('Ctrl Pts',(-0.0706003757388539,-0.226430877058226,
-0.775691661881254));
#80299=CARTESIAN_POINT('Ctrl Pts',(-0.0644760839380083,-0.228288490011239,
-0.775256183001657));
#80300=CARTESIAN_POINT('Ctrl Pts',(-0.0600726618567288,-0.229486536465834,
-0.77494167094121));
#80301=CARTESIAN_POINT('Ctrl Pts',(-0.0342912756779752,-0.235708068884862,
-0.773091154058116));
#80302=CARTESIAN_POINT('Ctrl Pts',(-0.012334723404674,-0.23786911401318,
-0.771465216336041));
#80303=CARTESIAN_POINT('Ctrl Pts',(0.0142702793627001,-0.236791460666137,
-0.769543698707242));
#80304=CARTESIAN_POINT('Ctrl Pts',(0.0189351741726104,-0.236464164594614,
-0.76920921404585));
#80305=CARTESIAN_POINT('Ctrl Pts',(0.0266148865212963,-0.235696594005048,
-0.768665484015001));
#80306=CARTESIAN_POINT('Ctrl Pts',(0.0296362452449061,-0.235335785030437,
-0.768453355713495));
#80307=CARTESIAN_POINT('Ctrl Pts',(0.0338346405148792,-0.234752269905424,
-0.768161824163811));
#80308=CARTESIAN_POINT('Ctrl Pts',(0.0350180576949475,-0.234578658262423,
-0.768080009261075));
#80309=CARTESIAN_POINT('Ctrl Pts',(0.0370359409354392,-0.234267016299158,
-0.767941176819243));
#80310=CARTESIAN_POINT('Ctrl Pts',(0.0378710642517986,-0.234133462864492,
-0.767883917651591));
#80311=CARTESIAN_POINT('Ctrl Pts',(0.039621576743821,-0.233843908322147,
-0.767764331222161));
#80312=CARTESIAN_POINT('Ctrl Pts',(0.0405367861275198,-0.233686995460666,
-0.767702054533213));
#80313=CARTESIAN_POINT('Ctrl Pts',(0.0430192709528315,-0.233246349788409,
-0.767533740606762));
#80314=CARTESIAN_POINT('Ctrl Pts',(0.0445846808497148,-0.2329521923832,
-0.767428266699933));
#80315=CARTESIAN_POINT('Ctrl Pts',(0.0524348418444053,-0.231395029778182,
-0.766902127638843));
#80316=CARTESIAN_POINT('Ctrl Pts',(0.0586700948759226,-0.229893253939525,
-0.76649320281935));
#80317=CARTESIAN_POINT('Ctrl Pts',(0.0662048283548098,-0.227751887474845,
-0.76600167283361));
#80318=CARTESIAN_POINT('Ctrl Pts',(0.0675687648985846,-0.227350970230419,
-0.765912804064903));
#80319=CARTESIAN_POINT('Ctrl Pts',(0.0899020344941972,-0.220567567022637,
-0.764458242766159));
#80320=CARTESIAN_POINT('Ctrl Pts',(0.109889800372382,-0.211321289523077,
-0.763153778113318));
#80321=CARTESIAN_POINT('Ctrl Pts',(0.131722773197877,-0.197274995830279,
-0.761488973731165));
#80322=CARTESIAN_POINT('Ctrl Pts',(0.135064870568817,-0.195002027196108,
-0.761227066196734));
#80323=CARTESIAN_POINT('Ctrl Pts',(0.139891081222704,-0.191536104288281,
-0.76083729983917));
#80324=CARTESIAN_POINT('Ctrl Pts',(0.141421617645303,-0.190408822182136,
-0.760711925659996));
#80325=CARTESIAN_POINT('Ctrl Pts',(0.14412042064837,-0.188370589690317,
-0.760487583921135));
#80326=CARTESIAN_POINT('Ctrl Pts',(0.145294026137241,-0.187466851755349,
-0.760388900747177));
#80327=CARTESIAN_POINT('Ctrl Pts',(0.147757850932039,-0.185532543362412,
-0.760179286483267));
#80328=CARTESIAN_POINT('Ctrl Pts',(0.149045921789106,-0.18449937701233,
-0.760068255638467));
#80329=CARTESIAN_POINT('Ctrl Pts',(0.152476097930082,-0.181688657168324,
-0.759768596998929));
#80330=CARTESIAN_POINT('Ctrl Pts',(0.154597815934039,-0.17988674978199,
-0.759578994951345));
#80331=CARTESIAN_POINT('Ctrl Pts',(0.167450880452792,-0.168575689988455,
-0.758403419182736));
#80332=CARTESIAN_POINT('Ctrl Pts',(0.177331528405163,-0.158148535889789,
-0.75737876480446));
#80333=CARTESIAN_POINT('Ctrl Pts',(0.19376050250694,-0.137322632022481,
-0.755449329762304));
#80334=CARTESIAN_POINT('Ctrl Pts',(0.200562681729688,-0.127181996869711,
-0.754553017852833));
#80335=CARTESIAN_POINT('Ctrl Pts',(0.209265022608862,-0.111761060622614,
-0.75328367448168));
#80336=CARTESIAN_POINT('Ctrl Pts',(0.211806899978007,-0.106865486382851,
-0.752893510079721));
#80337=CARTESIAN_POINT('Ctrl Pts',(0.214809111322174,-0.100554454992311,
-0.752410318534097));
#80338=CARTESIAN_POINT('Ctrl Pts',(0.215429827972977,-0.0992176507569932,
-0.752309066816212));
#80339=CARTESIAN_POINT('Ctrl Pts',(0.216410519045071,-0.0970529879635057,
-0.752146975166385));
#80340=CARTESIAN_POINT('Ctrl Pts',(0.216778287851915,-0.0962287338101404,
-0.752085685914123));
#80341=CARTESIAN_POINT('Ctrl Pts',(0.217482753559935,-0.0946253290524609,
-0.751967324707513));
#80342=CARTESIAN_POINT('Ctrl Pts',(0.217819986106068,-0.0938464420023404,
-0.751910223227109));
#80343=CARTESIAN_POINT('Ctrl Pts',(0.21864740524201,-0.0919069100884264,
-0.751768973313796));
#80344=CARTESIAN_POINT('Ctrl Pts',(0.219132547910465,-0.0907441158534499,
-0.751685122162888));
#80345=CARTESIAN_POINT('Ctrl Pts',(0.220829804977394,-0.0865831153656113,
-0.751387829635319));
#80346=CARTESIAN_POINT('Ctrl Pts',(0.221989897870175,-0.0835639057725772,
-0.751177203677069));
#80347=CARTESIAN_POINT('Ctrl Pts',(0.228898777052709,-0.0644226445820406,
-0.749867963497479));
#80348=CARTESIAN_POINT('Ctrl Pts',(0.23295052181949,-0.0477400874244471,
-0.748839220775789));
#80349=CARTESIAN_POINT('Ctrl Pts',(0.2362326420317,-0.0226512805388733,
-0.74728005788235));
#80350=CARTESIAN_POINT('Ctrl Pts',(0.236873409534906,-0.0144884324855405,
-0.746771477834052));
#80351=CARTESIAN_POINT('Ctrl Pts',(0.237188001756677,-0.00266660625486337,
-0.746020367335511));
#80352=CARTESIAN_POINT('Ctrl Pts',(0.237200971930077,0.000977646550547964,
-0.745786873236991));
#80353=CARTESIAN_POINT('Ctrl Pts',(0.237072432994858,0.00757426651137478,
-0.745359648491185));
#80354=CARTESIAN_POINT('Ctrl Pts',(0.236959701431725,0.010526473306441,
-0.745166795065436));
#80355=CARTESIAN_POINT('Ctrl Pts',(0.236695990931515,0.0151603322331561,
-0.744861109222533));
#80356=CARTESIAN_POINT('Ctrl Pts',(0.236582146687212,0.0168438540210009,
-0.744749432854298));
#80357=CARTESIAN_POINT('Ctrl Pts',(0.236335087941687,0.0199971080462435,
-0.744539035603704));
#80358=CARTESIAN_POINT('Ctrl Pts',(0.236206100040325,0.0214670970900954,
-0.744440451623429));
#80359=CARTESIAN_POINT('Ctrl Pts',(0.235885195639102,0.0247699651876454,
-0.744217775165685));
#80360=CARTESIAN_POINT('Ctrl Pts',(0.235685618385446,0.0266019858427822,
-0.744093448440545));
#80361=CARTESIAN_POINT('Ctrl Pts',(0.235017783912248,0.0321328838702285,
-0.743715549810751));
#80362=CARTESIAN_POINT('Ctrl Pts',(0.234483658093562,0.0358230699105591,
-0.743459944580654));
#80363=CARTESIAN_POINT('Ctrl Pts',(0.230715549343527,0.0581330366572575,
-0.741892646899228));
#80364=CARTESIAN_POINT('Ctrl Pts',(0.225352893163457,0.076321280890389,
-0.740513586993792));
#80365=CARTESIAN_POINT('Ctrl Pts',(0.213879115252791,0.103009220083144,
-0.73839550128084));
#80366=CARTESIAN_POINT('Ctrl Pts',(0.209270984531721,0.112075288506107,
-0.737659156215842));
#80367=CARTESIAN_POINT('Ctrl Pts',(0.20292265519373,0.122799326892156,-0.736787793651319));
#80368=CARTESIAN_POINT('Ctrl Pts',(0.201721300988386,0.124762960779748,
-0.736628249504553));
#80369=CARTESIAN_POINT('Ctrl Pts',(0.199918736181254,0.127615159527899,
-0.736396863250624));
#80370=CARTESIAN_POINT('Ctrl Pts',(0.199339824249572,0.128517565326425,
-0.736323707961385));
#80371=CARTESIAN_POINT('Ctrl Pts',(0.198344866478263,0.130045603410437,
-0.736199966154704));
#80372=CARTESIAN_POINT('Ctrl Pts',(0.197931941809173,0.130673224091904,
-0.736149180673524));
#80373=CARTESIAN_POINT('Ctrl Pts',(0.196981561896402,0.132102902952194,
-0.736033592095689));
#80374=CARTESIAN_POINT('Ctrl Pts',(0.196442184261917,0.132903653149059,
-0.735968917779509));
#80375=CARTESIAN_POINT('Ctrl Pts',(0.194930145149593,0.135119082237537,
-0.73579010040145));
#80376=CARTESIAN_POINT('Ctrl Pts',(0.19394696846424,0.136526560475476,-0.735676629559511));
#80377=CARTESIAN_POINT('Ctrl Pts',(0.186701717207357,0.146662345511946,
-0.734859472681156));
#80378=CARTESIAN_POINT('Ctrl Pts',(0.179867522040419,0.154968089685708,
-0.734189516803673));
#80379=CARTESIAN_POINT('Ctrl Pts',(0.171514596426131,0.163819276462219,
-0.733439291905644));
#80380=CARTESIAN_POINT('Ctrl Pts',(0.170527020822667,0.164847042260522,
-0.733351585801587));
#80381=CARTESIAN_POINT('Ctrl Pts',(0.162741367645642,0.172804699767231,
-0.732667307776094));
#80382=CARTESIAN_POINT('Ctrl Pts',(0.155533027485139,0.179320077836887,
-0.732075486152717));
#80383=CARTESIAN_POINT('Ctrl Pts',(0.142718693961479,0.189547040782069,
-0.731058517166502));
#80384=CARTESIAN_POINT('Ctrl Pts',(0.137317809386962,0.193495518692476,
-0.730639364687499));
#80385=CARTESIAN_POINT('Ctrl Pts',(0.127885098388096,0.199797578191137,
-0.729915321819036));
#80386=CARTESIAN_POINT('Ctrl Pts',(0.123937464666749,0.202270044446317,
-0.729614560020163));
#80387=CARTESIAN_POINT('Ctrl Pts',(0.118188578525612,0.205639167167795,
-0.729178185644532));
#80388=CARTESIAN_POINT('Ctrl Pts',(0.116444586969378,0.206631713257822,
-0.729046017603098));
#80389=CARTESIAN_POINT('Ctrl Pts',(0.113379146882102,0.208325194034733,
-0.728813955615001));
#80390=CARTESIAN_POINT('Ctrl Pts',(0.112063253908587,0.209035988208327,
-0.728714418841939));
#80391=CARTESIAN_POINT('Ctrl Pts',(0.109324243271386,0.210482199589635,
-0.728507352556175));
#80392=CARTESIAN_POINT('Ctrl Pts',(0.10790022507186,0.211215737393647,-0.728399763247817));
#80393=CARTESIAN_POINT('Ctrl Pts',(0.104188824945857,0.213080220173569,
-0.728119463688626));
#80394=CARTESIAN_POINT('Ctrl Pts',(0.101890479069181,0.214188750556311,
-0.72794598801542));
#80395=CARTESIAN_POINT('Ctrl Pts',(0.0918328649533584,0.218841193512923,
-0.727187028668554));
#80396=CARTESIAN_POINT('Ctrl Pts',(0.0839043062420878,0.222001756949136,
-0.726588852080559));
#80397=CARTESIAN_POINT('Ctrl Pts',(0.0556350911330214,0.231539822584417,
-0.724457845182605));
#80398=CARTESIAN_POINT('Ctrl Pts',(0.0346231366805335,0.235599420765083,
-0.722867160341234));
#80399=CARTESIAN_POINT('Ctrl Pts',(0.0101497653412854,0.236979439200232,
-0.72113770438752));
#80400=CARTESIAN_POINT('Ctrl Pts',(0.00694325102918205,0.237095057059841,
-0.720913758441859));
#80401=CARTESIAN_POINT('Ctrl Pts',(0.00251482073951898,0.237164807630886,
-0.720608984977922));
#80402=CARTESIAN_POINT('Ctrl Pts',(0.00129428535896178,0.237174609283586,
-0.720525458491378));
#80403=CARTESIAN_POINT('Ctrl Pts',(-0.000776229268319339,0.237175252642923,
-0.720384627420986));
#80404=CARTESIAN_POINT('Ctrl Pts',(-0.00162617263924265,0.237170948166812,
-0.7203270638331));
#80405=CARTESIAN_POINT('Ctrl Pts',(-0.00339484677249993,0.237152482204098,
-0.720207813836742));
#80406=CARTESIAN_POINT('Ctrl Pts',(-0.00431354279396595,0.237137551266237,
-0.720146169317013));
#80407=CARTESIAN_POINT('Ctrl Pts',(-0.00677979150403611,0.237083131871023,
-0.719981425867255));
#80408=CARTESIAN_POINT('Ctrl Pts',(-0.0083271139171756,0.237033829817099,
-0.719878850377708));
#80409=CARTESIAN_POINT('Ctrl Pts',(-0.0156375495891087,0.236729223125891,
-0.719397463961534));
#80410=CARTESIAN_POINT('Ctrl Pts',(-0.0213910559553792,0.236278845228366,
-0.719028103608231));
#80411=CARTESIAN_POINT('Ctrl Pts',(-0.0320841269560271,0.235047929974299,
-0.718349970038989));
#80412=CARTESIAN_POINT('Ctrl Pts',(-0.0370242168771452,0.234320486803334,
-0.718040032741223));
#80413=CARTESIAN_POINT('Ctrl Pts',(-0.0419358371735614,0.233438142096686,
-0.71773215975824));
#80414=CARTESIAN_POINT('Origin',(0.,0.,-1.7456589891905));
#80415=CARTESIAN_POINT('',(-0.0419358081412419,0.233438147312176,-0.598166693585937));
#80416=CARTESIAN_POINT('',(-0.0419358257187831,0.233438144154472,-0.618049599588275));
#80417=CARTESIAN_POINT('',(-0.0419358257166344,0.233438144154858,-1.7456589891905));
#80418=CARTESIAN_POINT('',(-0.237174993928743,-0.0001557562965092,-0.676096353182709));
#80419=CARTESIAN_POINT('Ctrl Pts',(-0.0419358081412227,0.233438147312179,
-0.598166693585938));
#80420=CARTESIAN_POINT('Ctrl Pts',(-0.0254221450267922,0.236404731034887,
-0.599196757273924));
#80421=CARTESIAN_POINT('Ctrl Pts',(-0.00862997878185331,0.237612619833391,
-0.600218908972521));
#80422=CARTESIAN_POINT('Ctrl Pts',(0.0119921080420857,0.236902656990329,
-0.601544371140064));
#80423=CARTESIAN_POINT('Ctrl Pts',(0.0158198069622217,0.236677862496629,
-0.601793151172967));
#80424=CARTESIAN_POINT('Ctrl Pts',(0.0214968765434211,0.23620613017656,
-0.60216707457608));
#80425=CARTESIAN_POINT('Ctrl Pts',(0.0233516142688545,0.236029984145217,
-0.602290022757764));
#80426=CARTESIAN_POINT('Ctrl Pts',(0.0266734177630653,0.235674973507113,
-0.602511720379031));
#80427=CARTESIAN_POINT('Ctrl Pts',(0.0281412653325034,0.23550421093767,
-0.602610211349407));
#80428=CARTESIAN_POINT('Ctrl Pts',(0.0312689983012018,0.235110686713298,
-0.602821248214161));
#80429=CARTESIAN_POINT('Ctrl Pts',(0.0329283042571606,0.234884039030316,
-0.602933911226548));
#80430=CARTESIAN_POINT('Ctrl Pts',(0.0374468861669076,0.234218016968055,
-0.603242705178056));
#80431=CARTESIAN_POINT('Ctrl Pts',(0.040300665144993,0.233743885183556,
-0.603439915385624));
#80432=CARTESIAN_POINT('Ctrl Pts',(0.0585602015538563,0.230365896083917,
-0.604716348384372));
#80433=CARTESIAN_POINT('Ctrl Pts',(0.0736519686150716,0.225993287091945,
-0.605842255293825));
#80434=CARTESIAN_POINT('Ctrl Pts',(0.102101467728049,0.214596245297013,
-0.608076415713036));
#80435=CARTESIAN_POINT('Ctrl Pts',(0.115445624116596,0.207722496911975,
-0.609177482037637));
#80436=CARTESIAN_POINT('Ctrl Pts',(0.129882729989079,0.198462041042995,
-0.610374961558479));
#80437=CARTESIAN_POINT('Ctrl Pts',(0.131696184824981,0.197263329130861,
-0.610525449874029));
#80438=CARTESIAN_POINT('Ctrl Pts',(0.134359360904778,0.195449843766908,
-0.610746267349269));
#80439=CARTESIAN_POINT('Ctrl Pts',(0.135221840899336,0.194854132980955,
-0.610817750646774));
#80440=CARTESIAN_POINT('Ctrl Pts',(0.136759936686426,0.193776646679321,
-0.610945136366521));
#80441=CARTESIAN_POINT('Ctrl Pts',(0.137437002081487,0.193297024291547,
-0.611001175275601));
#80442=CARTESIAN_POINT('Ctrl Pts',(0.138941630224246,0.192219266786862,
-0.611125630498796));
#80443=CARTESIAN_POINT('Ctrl Pts',(0.139767860574496,0.191619331958714,
-0.611193923701551));
#80444=CARTESIAN_POINT('Ctrl Pts',(0.142228711015798,0.189808096342956,
-0.611397268602092));
#80445=CARTESIAN_POINT('Ctrl Pts',(0.14385169473178,0.188581044319087,-0.611531298938028));
#80446=CARTESIAN_POINT('Ctrl Pts',(0.155723433502437,0.179362986695429,
-0.612512767818748));
#80447=CARTESIAN_POINT('Ctrl Pts',(0.165317106780871,0.170561464048922,
-0.613312587419873));
#80448=CARTESIAN_POINT('Ctrl Pts',(0.185685693554085,0.148532550951544,
-0.615153658607073));
#80449=CARTESIAN_POINT('Ctrl Pts',(0.195851971144819,0.134844448967748,
-0.61619079048841));
#80450=CARTESIAN_POINT('Ctrl Pts',(0.206018158725287,0.117549417105015,
-0.617484360355525));
#80451=CARTESIAN_POINT('Ctrl Pts',(0.207517777186748,0.114881321239951,
-0.617683337203257));
#80452=CARTESIAN_POINT('Ctrl Pts',(0.209858952545478,0.110520451363784,
-0.618008079954614));
#80453=CARTESIAN_POINT('Ctrl Pts',(0.210732664128625,0.108845275777767,
-0.618132713877082));
#80454=CARTESIAN_POINT('Ctrl Pts',(0.212255097573913,0.105839244220124,
-0.618356260416211));
#80455=CARTESIAN_POINT('Ctrl Pts',(0.21291155406122,0.104512401373171,-0.618454896715161));
#80456=CARTESIAN_POINT('Ctrl Pts',(0.2142770926733,0.101686081651301,-0.618664972572333));
#80457=CARTESIAN_POINT('Ctrl Pts',(0.214982949032665,0.100185143755965,
-0.61877651720911));
#80458=CARTESIAN_POINT('Ctrl Pts',(0.216844954679859,0.0961154568577069,
-0.619078980509639));
#80459=CARTESIAN_POINT('Ctrl Pts',(0.217971147074729,0.093533380531618,
-0.619270904883523));
#80460=CARTESIAN_POINT('Ctrl Pts',(0.225327756282748,0.0758116349300416,
-0.620588836354732));
#80461=CARTESIAN_POINT('Ctrl Pts',(0.230020923519952,0.0600848518164682,
-0.621766366989002));
#80462=CARTESIAN_POINT('Ctrl Pts',(0.235717451081462,0.0299140326794427,
-0.624005869970449));
#80463=CARTESIAN_POINT('Ctrl Pts',(0.237094742794941,0.0156114064133701,
-0.625058306584018));
#80464=CARTESIAN_POINT('Ctrl Pts',(0.237183531140776,-0.000956382651459844,
-0.626215759581499));
#80465=CARTESIAN_POINT('Ctrl Pts',(0.23716408975447,-0.00318394967359194,
-0.626370049883849));
#80466=CARTESIAN_POINT('Ctrl Pts',(0.237089120648149,-0.00646913497271217,
-0.626595318404422));
#80467=CARTESIAN_POINT('Ctrl Pts',(0.237057890662872,-0.00752711226960892,
-0.626667516378383));
#80468=CARTESIAN_POINT('Ctrl Pts',(0.236989533019771,-0.00941439762022854,
-0.626795643777125));
#80469=CARTESIAN_POINT('Ctrl Pts',(0.236955133153033,-0.0102437581127221,
-0.626851717077923));
#80470=CARTESIAN_POINT('Ctrl Pts',(0.236869132238768,-0.0120838279260917,
-0.626975609732613));
#80471=CARTESIAN_POINT('Ctrl Pts',(0.236815416311022,-0.0130944032460889,
-0.627043312639457));
#80472=CARTESIAN_POINT('Ctrl Pts',(0.236636943089448,-0.0160901910361994,
-0.627243088790108));
#80473=CARTESIAN_POINT('Ctrl Pts',(0.236493675453163,-0.0180742687312584,
-0.627374193136596));
#80474=CARTESIAN_POINT('Ctrl Pts',(0.236102893316887,-0.022678874836118,
-0.627676144350482));
#80475=CARTESIAN_POINT('Ctrl Pts',(0.235836682221959,-0.0252975913978463,
-0.627846124830268));
#80476=CARTESIAN_POINT('Ctrl Pts',(0.234742661646349,-0.0345293345070006,
-0.62844089282821));
#80477=CARTESIAN_POINT('Ctrl Pts',(0.233679764606343,-0.0411117012407693,
-0.62885690197077));
#80478=CARTESIAN_POINT('Ctrl Pts',(0.229229620746353,-0.0628146747479831,
-0.63022648121314));
#80479=CARTESIAN_POINT('Ctrl Pts',(0.224639485495002,-0.0776466328464153,
-0.631161557424502));
#80480=CARTESIAN_POINT('Ctrl Pts',(0.215881452904409,-0.0984768579057991,
-0.632580891960774));
#80481=CARTESIAN_POINT('Ctrl Pts',(0.212833942722427,-0.104900864653528,
-0.633034050834307));
#80482=CARTESIAN_POINT('Ctrl Pts',(0.208377679281489,-0.113298212396497,
-0.633653354842134));
#80483=CARTESIAN_POINT('Ctrl Pts',(0.207220420950265,-0.115401207132185,
-0.6338107861835));
#80484=CARTESIAN_POINT('Ctrl Pts',(0.205253617800437,-0.118850321237735,
-0.6340730813022));
#80485=CARTESIAN_POINT('Ctrl Pts',(0.2044622455822,-0.120206640454447,-0.634177293001574));
#80486=CARTESIAN_POINT('Ctrl Pts',(0.20288262444362,-0.122853193269345,
-0.6343827998943));
#80487=CARTESIAN_POINT('Ctrl Pts',(0.202095389948195,-0.124143947000845,
-0.634484054651069));
#80488=CARTESIAN_POINT('Ctrl Pts',(0.200184120121785,-0.127211313384452,
-0.634727194825757));
#80489=CARTESIAN_POINT('Ctrl Pts',(0.199048714417582,-0.128980653574054,
-0.634869493261507));
#80490=CARTESIAN_POINT('Ctrl Pts',(0.194983686028365,-0.135133793066106,
-0.635371747363606));
#80491=CARTESIAN_POINT('Ctrl Pts',(0.191931734639848,-0.139434506144744,
-0.635736208131257));
#80492=CARTESIAN_POINT('Ctrl Pts',(0.183898819826625,-0.149990305384879,
-0.636665798194291));
#80493=CARTESIAN_POINT('Ctrl Pts',(0.178740416319221,-0.156101601947246,
-0.637236961096213));
#80494=CARTESIAN_POINT('Ctrl Pts',(0.162893501051262,-0.173058544879358,
-0.638915688254464));
#80495=CARTESIAN_POINT('Ctrl Pts',(0.151457539839905,-0.183150655761056,
-0.640039666721596));
#80496=CARTESIAN_POINT('Ctrl Pts',(0.13509613273099,-0.195002232324807,
-0.641484270233975));
#80497=CARTESIAN_POINT('Ctrl Pts',(0.130967052994491,-0.197799076981264,
-0.64183628707571));
#80498=CARTESIAN_POINT('Ctrl Pts',(0.125505612222618,-0.201252325275129,
-0.642283043813516));
#80499=CARTESIAN_POINT('Ctrl Pts',(0.124251299019681,-0.202029136752836,
-0.642384399980747));
#80500=CARTESIAN_POINT('Ctrl Pts',(0.122217637220845,-0.203262503360613,
-0.642546629224881));
#80501=CARTESIAN_POINT('Ctrl Pts',(0.121442810269847,-0.203726385190649,
-0.642607952739965));
#80502=CARTESIAN_POINT('Ctrl Pts',(0.119925862543786,-0.204622838186182,
-0.642727037779076));
#80503=CARTESIAN_POINT('Ctrl Pts',(0.119184014324925,-0.205055819654559,
-0.642784822840843));
#80504=CARTESIAN_POINT('Ctrl Pts',(0.117341439604361,-0.206117865386348,
-0.642927270717096));
#80505=CARTESIAN_POINT('Ctrl Pts',(0.116237969485084,-0.206742164319824,
-0.643011635539818));
#80506=CARTESIAN_POINT('Ctrl Pts',(0.112027475051262,-0.209079923734588,
-0.643330184690371));
#80507=CARTESIAN_POINT('Ctrl Pts',(0.108886975712574,-0.210732530503391,
-0.643560886242645));
#80508=CARTESIAN_POINT('Ctrl Pts',(0.100485327899274,-0.214915677979137,
-0.644163197051283));
#80509=CARTESIAN_POINT('Ctrl Pts',(0.0951656623110755,-0.217323619336894,
-0.644529540295748));
#80510=CARTESIAN_POINT('Ctrl Pts',(0.0734052644079443,-0.226220971319432,
-0.645989150630036));
#80511=CARTESIAN_POINT('Ctrl Pts',(0.0563525568726708,-0.231059862047319,
-0.647050118704931));
#80512=CARTESIAN_POINT('Ctrl Pts',(0.0326517920539688,-0.235002604092262,
-0.64856554051873));
#80513=CARTESIAN_POINT('Ctrl Pts',(0.0263442896189105,-0.235792983379444,
-0.648972092401514));
#80514=CARTESIAN_POINT('Ctrl Pts',(0.0177048424013525,-0.236524597525799,
-0.649537507771648));
#80515=CARTESIAN_POINT('Ctrl Pts',(0.0153939593854007,-0.236686231269615,
-0.649689563931334));
#80516=CARTESIAN_POINT('Ctrl Pts',(0.0116853925224909,-0.236891085300731,
-0.649935068895511));
#80517=CARTESIAN_POINT('Ctrl Pts',(0.0102890119420583,-0.236955841424199,
-0.650027844177806));
#80518=CARTESIAN_POINT('Ctrl Pts',(0.00739135622624884,-0.237064556770727,
-0.650221100073976));
#80519=CARTESIAN_POINT('Ctrl Pts',(0.00589007661193041,-0.237106606914802,
-0.65032163580469));
#80520=CARTESIAN_POINT('Ctrl Pts',(0.0023451099182259,-0.237172211847015,
-0.650560044518362));
#80521=CARTESIAN_POINT('Ctrl Pts',(0.00030134593148767,-0.237183613155478,
-0.650698289079158));
#80522=CARTESIAN_POINT('Ctrl Pts',(-0.00662944787624838,-0.237132699095051,
-0.651169931887045));
#80523=CARTESIAN_POINT('Ctrl Pts',(-0.0115140257062346,-0.236945748439082,
-0.651507131789606));
#80524=CARTESIAN_POINT('Ctrl Pts',(-0.0235319717630752,-0.236113305609175,
-0.652349115436499));
#80525=CARTESIAN_POINT('Ctrl Pts',(-0.0306482200249554,-0.235295383454555,
-0.652858545101209));
#80526=CARTESIAN_POINT('Ctrl Pts',(-0.0515773785350495,-0.23192428909589,
-0.654385705086018));
#80527=CARTESIAN_POINT('Ctrl Pts',(-0.0652123119607416,-0.228465379814004,
-0.655420086630226));
#80528=CARTESIAN_POINT('Ctrl Pts',(-0.0852700433744059,-0.221434103803698,
-0.656956059504935));
#80529=CARTESIAN_POINT('Ctrl Pts',(-0.0919674338717087,-0.218737410346294,
-0.657471028387694));
#80530=CARTESIAN_POINT('Ctrl Pts',(-0.100023740761862,-0.215057948624918,
-0.658084992788055));
#80531=CARTESIAN_POINT('Ctrl Pts',(-0.10150839749602,-0.214361180242974,
-0.658197896359277));
#80532=CARTESIAN_POINT('Ctrl Pts',(-0.103831569298598,-0.213241336199695,
-0.658374051223744));
#80533=CARTESIAN_POINT('Ctrl Pts',(-0.104674970217722,-0.212828599896492,
-0.658437894269272));
#80534=CARTESIAN_POINT('Ctrl Pts',(-0.106270291710927,-0.212036117764972,
-0.658558419102347));
#80535=CARTESIAN_POINT('Ctrl Pts',(-0.10702264465679,-0.211657373339644,
-0.65861515412681));
#80536=CARTESIAN_POINT('Ctrl Pts',(-0.108818387676643,-0.2107413493865,
-0.658750349768238));
#80537=CARTESIAN_POINT('Ctrl Pts',(-0.109859833910577,-0.210200320822271,
-0.658828578959192));
#80538=CARTESIAN_POINT('Ctrl Pts',(-0.11345639737131,-0.208297883409675,
-0.659098269207776));
#80539=CARTESIAN_POINT('Ctrl Pts',(-0.115990686519285,-0.206897377477604,
-0.659287478418883));
#80540=CARTESIAN_POINT('Ctrl Pts',(-0.122276027636513,-0.203272150498366,
-0.659756273393061));
#80541=CARTESIAN_POINT('Ctrl Pts',(-0.125992653494476,-0.200989675967165,
-0.66003305837453));
#80542=CARTESIAN_POINT('Ctrl Pts',(-0.144382831962948,-0.188985075673307,
-0.661411338882494));
#80543=CARTESIAN_POINT('Ctrl Pts',(-0.158004883305195,-0.177753415174447,
-0.662465008083218));
#80544=CARTESIAN_POINT('Ctrl Pts',(-0.176035409497053,-0.159161404786691,
-0.664081942404345));
#80545=CARTESIAN_POINT('Ctrl Pts',(-0.18149448785661,-0.152906988412833,
-0.664608077367209));
#80546=CARTESIAN_POINT('Ctrl Pts',(-0.188185156633312,-0.144377302101673,
-0.66531310005692));
#80547=CARTESIAN_POINT('Ctrl Pts',(-0.189723601015048,-0.142349615176432,
-0.665479810184046));
#80548=CARTESIAN_POINT('Ctrl Pts',(-0.192175986657686,-0.139006954004205,
-0.665753440965162));
#80549=CARTESIAN_POINT('Ctrl Pts',(-0.193109792681398,-0.137706756798118,
-0.665859588495997));
#80550=CARTESIAN_POINT('Ctrl Pts',(-0.194891057151493,-0.135172839099616,
-0.666065962731003));
#80551=CARTESIAN_POINT('Ctrl Pts',(-0.195740141373546,-0.133940350403645,
-0.66616612093219));
#80552=CARTESIAN_POINT('Ctrl Pts',(-0.197702763545825,-0.131032983914976,
-0.666401919341045));
#80553=CARTESIAN_POINT('Ctrl Pts',(-0.198806759563053,-0.12935183611636,
-0.666537908407954));
#80554=CARTESIAN_POINT('Ctrl Pts',(-0.202409960729904,-0.123709829521019,
-0.666993235027753));
#80555=CARTESIAN_POINT('Ctrl Pts',(-0.204813079676133,-0.11968922743183,
-0.667316025101611));
#80556=CARTESIAN_POINT('Ctrl Pts',(-0.210380587762926,-0.109715160684738,
-0.66811322386183));
#80557=CARTESIAN_POINT('Ctrl Pts',(-0.213413072176007,-0.10369308188169,
-0.668591649728554));
#80558=CARTESIAN_POINT('Ctrl Pts',(-0.221146560693454,-0.086554646524819,
-0.669943005404033));
#80559=CARTESIAN_POINT('Ctrl Pts',(-0.225261943314332,-0.0751966571714988,
-0.670827943183893));
#80560=CARTESIAN_POINT('Ctrl Pts',(-0.230594554077849,-0.0560309185231766,
-0.672275595529859));
#80561=CARTESIAN_POINT('Ctrl Pts',(-0.232318998884028,-0.0483860977031188,
-0.672841283419945));
#80562=CARTESIAN_POINT('Ctrl Pts',(-0.23416464690543,-0.0377821103525075,
-0.673599178279029));
#80563=CARTESIAN_POINT('Ctrl Pts',(-0.234613658122349,-0.0348855709440824,
-0.67380348000132));
#80564=CARTESIAN_POINT('Ctrl Pts',(-0.235172281465171,-0.0307806264262929,
-0.674088505595738));
#80565=CARTESIAN_POINT('Ctrl Pts',(-0.235326475929421,-0.029578688570418,
-0.674171417730161));
#80566=CARTESIAN_POINT('Ctrl Pts',(-0.235571977813158,-0.0275414203955394,
-0.674310973167934));
#80567=CARTESIAN_POINT('Ctrl Pts',(-0.235668069094306,-0.0267067008142211,
-0.674367874033798));
#80568=CARTESIAN_POINT('Ctrl Pts',(-0.235844305886976,-0.0251007016344489,
-0.674476797423961));
#80569=CARTESIAN_POINT('Ctrl Pts',(-0.235925107203615,-0.0243295227284101,
-0.674528858597173));
#80570=CARTESIAN_POINT('Ctrl Pts',(-0.236093302054964,-0.0226445566463216,
-0.674642106499908));
#80571=CARTESIAN_POINT('Ctrl Pts',(-0.236179176032279,-0.0217306257910065,
-0.674703210718419));
#80572=CARTESIAN_POINT('Ctrl Pts',(-0.236377821313897,-0.0194760413468157,
-0.674853207377661));
#80573=CARTESIAN_POINT('Ctrl Pts',(-0.236484497302592,-0.0181348649376064,
-0.674941789389455));
#80574=CARTESIAN_POINT('Ctrl Pts',(-0.236972764746139,-0.0112560792173358,
-0.675393144633294));
#80575=CARTESIAN_POINT('Ctrl Pts',(-0.237171311127635,-0.00570685717802064,
-0.675747402338223));
#80576=CARTESIAN_POINT('Ctrl Pts',(-0.23717494907381,-0.000155424694679885,
-0.676096452130946));
#80577=CARTESIAN_POINT('Ctrl Pts',(-0.237174948853082,-0.000155761157073058,
-0.676096430975656));
#80578=CARTESIAN_POINT('Ctrl Pts',(-0.237176131619272,0.00164521744310811,
-0.676209668702917));
#80579=CARTESIAN_POINT('Ctrl Pts',(-0.237156800878312,0.00344619272531007,
-0.6763223419202));
#80580=CARTESIAN_POINT('Ctrl Pts',(-0.236632262479393,0.0271514288203653,
-0.677799910882799));
#80581=CARTESIAN_POINT('Ctrl Pts',(-0.233114967187122,0.0488821808950842,
-0.679103892791132));
#80582=CARTESIAN_POINT('Ctrl Pts',(-0.225475340087641,0.0736829308826454,
-0.680768049409323));
#80583=CARTESIAN_POINT('Ctrl Pts',(-0.224187565790029,0.0775128089572374,
-0.681029881008752));
#80584=CARTESIAN_POINT('Ctrl Pts',(-0.222150985036203,0.0830935264079915,
-0.681419577313486));
#80585=CARTESIAN_POINT('Ctrl Pts',(-0.221477872125114,0.0848713502481855,
-0.681544959336536));
#80586=CARTESIAN_POINT('Ctrl Pts',(-0.220242232828114,0.0880200814149191,
-0.681769334959095));
#80587=CARTESIAN_POINT('Ctrl Pts',(-0.219688086723308,0.0893941845715376,
-0.681868044308226));
#80588=CARTESIAN_POINT('Ctrl Pts',(-0.218488931293419,0.0922892005166868,
-0.682077735640644));
#80589=CARTESIAN_POINT('Ctrl Pts',(-0.217840835400568,0.0938087406520756,
-0.682188817634891));
#80590=CARTESIAN_POINT('Ctrl Pts',(-0.216057395657699,0.0978720691405405,
-0.682488669923413));
#80591=CARTESIAN_POINT('Ctrl Pts',(-0.214893052349189,0.100402764109508,
-0.682678416226039));
#80592=CARTESIAN_POINT('Ctrl Pts',(-0.207670117940391,0.115400282809999,
-0.683821390903903));
#80593=CARTESIAN_POINT('Ctrl Pts',(-0.200573694635737,0.127334903380162,
-0.684810557140656));
#80594=CARTESIAN_POINT('Ctrl Pts',(-0.186601645312739,0.146741038340641,
-0.686548379433072));
#80595=CARTESIAN_POINT('Ctrl Pts',(-0.180212864392938,0.15451999834099,
-0.687286219524909));
#80596=CARTESIAN_POINT('Ctrl Pts',(-0.169734318855455,0.165741673566535,
-0.688397856163317));
#80597=CARTESIAN_POINT('Ctrl Pts',(-0.165990068450785,0.169491431897337,
-0.688778278300537));
#80598=CARTESIAN_POINT('Ctrl Pts',(-0.160464972112714,0.174665779451608,
-0.689312879864408));
#80599=CARTESIAN_POINT('Ctrl Pts',(-0.158784487460708,0.176194861345632,
-0.689472141933913));
#80600=CARTESIAN_POINT('Ctrl Pts',(-0.155799362502275,0.178833640589542,
-0.689748883834113));
#80601=CARTESIAN_POINT('Ctrl Pts',(-0.154504210802291,0.17995377636246,
-0.689866982724218));
#80602=CARTESIAN_POINT('Ctrl Pts',(-0.152461338841841,0.181682276015678,
-0.690050059905405));
#80603=CARTESIAN_POINT('Ctrl Pts',(-0.151721878280214,0.182300249569067,
-0.690115685402815));
#80604=CARTESIAN_POINT('Ctrl Pts',(-0.150337771614902,0.18344270390224,
-0.690237297219541));
#80605=CARTESIAN_POINT('Ctrl Pts',(-0.149694126168726,0.183968311996618,
-0.690293359573696));
#80606=CARTESIAN_POINT('Ctrl Pts',(-0.14821110017765,0.185166430862028,
-0.69042142577379));
#80607=CARTESIAN_POINT('Ctrl Pts',(-0.147369893469756,0.185836627026,-0.690493267371959));
#80608=CARTESIAN_POINT('Ctrl Pts',(-0.144764757480524,0.187883345862392,
-0.690713404002494));
#80609=CARTESIAN_POINT('Ctrl Pts',(-0.142985828835886,0.189240694085377,
-0.690860441850481));
#80610=CARTESIAN_POINT('Ctrl Pts',(-0.130517234159927,0.198478188423581,
-0.691870589540606));
#80611=CARTESIAN_POINT('Ctrl Pts',(-0.119200025047789,0.205474535221661,
-0.692685528778348));
#80612=CARTESIAN_POINT('Ctrl Pts',(-0.0969139759614693,0.216787395682156,
-0.694218519411117));
#80613=CARTESIAN_POINT('Ctrl Pts',(-0.08609487775866,0.221306899623514,
-0.694934605455638));
#80614=CARTESIAN_POINT('Ctrl Pts',(-0.0686238496959238,0.227129330944396,
-0.696094590288248));
#80615=CARTESIAN_POINT('Ctrl Pts',(-0.0621742311787725,0.228978859401097,
-0.696523336191721));
#80616=CARTESIAN_POINT('Ctrl Pts',(-0.0534293545572765,0.231089870871603,
-0.697110187416785));
#80617=CARTESIAN_POINT('Ctrl Pts',(-0.0511957778673838,0.231594939659332,
-0.697260540388271));
#80618=CARTESIAN_POINT('Ctrl Pts',(-0.04744093726038,0.232387033733086,
-0.697514239950016));
#80619=CARTESIAN_POINT('Ctrl Pts',(-0.0459235145597242,0.232691655616345,
-0.697617021929088));
#80620=CARTESIAN_POINT('Ctrl Pts',(-0.0435815719511394,0.233137999666587,
-0.697776085609751));
#80621=CARTESIAN_POINT('Ctrl Pts',(-0.0427590860370097,0.233290250153061,
-0.697832030395872));
#80622=CARTESIAN_POINT('Ctrl Pts',(-0.0419358257124646,0.233438144155607,
-0.69788811322923));
#80623=CARTESIAN_POINT('Ctrl Pts',(-0.0419358371735614,0.233438142096686,
-0.71773215975824));
#80624=CARTESIAN_POINT('Ctrl Pts',(-0.0497809610582963,0.232028810121706,
-0.717240407231273));
#80625=CARTESIAN_POINT('Ctrl Pts',(-0.0575534454763789,0.230224291883822,
-0.716753801969153));
#80626=CARTESIAN_POINT('Ctrl Pts',(-0.0777437884470259,0.224449250421988,
-0.715462294220634));
#80627=CARTESIAN_POINT('Ctrl Pts',(-0.0899463043198536,0.219843497183554,
-0.714652378345264));
#80628=CARTESIAN_POINT('Ctrl Pts',(-0.104290403395135,0.213034414205457,
-0.713623231945516));
#80629=CARTESIAN_POINT('Ctrl Pts',(-0.106849984504534,0.211762200464446,
-0.713436507906509));
#80630=CARTESIAN_POINT('Ctrl Pts',(-0.110865054017541,0.209675224037858,
-0.713138344505617));
#80631=CARTESIAN_POINT('Ctrl Pts',(-0.112336063979543,0.208890804653252,
-0.713027965765718));
#80632=CARTESIAN_POINT('Ctrl Pts',(-0.115095743069493,0.207381619634535,
-0.712818663123878));
#80633=CARTESIAN_POINT('Ctrl Pts',(-0.116386148092833,0.206660181450482,
-0.712719861125174));
#80634=CARTESIAN_POINT('Ctrl Pts',(-0.119296637216579,0.204997083302212,
-0.712494841744148));
#80635=CARTESIAN_POINT('Ctrl Pts',(-0.120912458625922,0.20404820218007,
-0.712368369180192));
#80636=CARTESIAN_POINT('Ctrl Pts',(-0.125092352936989,0.201526503145301,
-0.71203705987452));
#80637=CARTESIAN_POINT('Ctrl Pts',(-0.12763797860691,0.199923918561245,
-0.711831156067895));
#80638=CARTESIAN_POINT('Ctrl Pts',(-0.144989126303658,0.188534129067977,
-0.710398330320745));
#80639=CARTESIAN_POINT('Ctrl Pts',(-0.15868331935262,0.177161924747622,
-0.709111149375821));
#80640=CARTESIAN_POINT('Ctrl Pts',(-0.179634174439599,0.155368957725207,
-0.706904462847015));
#80641=CARTESIAN_POINT('Ctrl Pts',(-0.187565676274929,0.145695333283181,
-0.705994121694069));
#80642=CARTESIAN_POINT('Ctrl Pts',(-0.195812214687322,0.133840792063366,
-0.704988726080134));
#80643=CARTESIAN_POINT('Ctrl Pts',(-0.196905748387745,0.132226729162066,
-0.704854051504146));
#80644=CARTESIAN_POINT('Ctrl Pts',(-0.198532033526139,0.129761396000316,
-0.704651893581959));
#80645=CARTESIAN_POINT('Ctrl Pts',(-0.199079455958728,0.128919969499633,
-0.704583511755803));
#80646=CARTESIAN_POINT('Ctrl Pts',(-0.200069889246839,0.127376251390834,
-0.704459211648246));
#80647=CARTESIAN_POINT('Ctrl Pts',(-0.200514564652106,0.126675093865161,
-0.704403189354044));
#80648=CARTESIAN_POINT('Ctrl Pts',(-0.201522544378047,0.125067118944162,
-0.704275692053643));
#80649=CARTESIAN_POINT('Ctrl Pts',(-0.202083418431739,0.124158818606778,
-0.704204373731682));
#80650=CARTESIAN_POINT('Ctrl Pts',(-0.203821306968238,0.121301440608357,
-0.703982102936987));
#80651=CARTESIAN_POINT('Ctrl Pts',(-0.204976439902245,0.119339116326712,
-0.703832473244526));
#80652=CARTESIAN_POINT('Ctrl Pts',(-0.212561699531826,0.106018213238358,
-0.70283474663507));
#80653=CARTESIAN_POINT('Ctrl Pts',(-0.218073788449209,0.0941607532235971,
-0.70203302924614));
#80654=CARTESIAN_POINT('Ctrl Pts',(-0.226678090051916,0.0707789930563413,
-0.70050466134681));
#80655=CARTESIAN_POINT('Ctrl Pts',(-0.229933024046881,0.0593582772207219,
-0.699779855484976));
#80656=CARTESIAN_POINT('Ctrl Pts',(-0.23323330035082,0.0432988444536064,
-0.698747429124093));
#80657=CARTESIAN_POINT('Ctrl Pts',(-0.234018790889593,0.0388299380059672,
-0.69845888792319));
#80658=CARTESIAN_POINT('Ctrl Pts',(-0.235181894355,0.030881757958909,-0.697941394202021));
#80659=CARTESIAN_POINT('Ctrl Pts',(-0.235611580532224,0.0274114480724389,
-0.697714014523));
#80660=CARTESIAN_POINT('Ctrl Pts',(-0.236145818593704,0.0221442059688947,
-0.697366102018109));
#80661=CARTESIAN_POINT('Ctrl Pts',(-0.23630690264025,0.0203534017962825,
-0.697247330401912));
#80662=CARTESIAN_POINT('Ctrl Pts',(-0.236562873147734,0.0170926033191336,
-0.697030101135011));
#80663=CARTESIAN_POINT('Ctrl Pts',(-0.236664456661271,0.0156232143271007,
-0.696931857921645));
#80664=CARTESIAN_POINT('Ctrl Pts',(-0.236855074759771,0.012434542356552,
-0.69671785016859));
#80665=CARTESIAN_POINT('Ctrl Pts',(-0.236939088379264,0.0107150553093824,
-0.696601934500364));
#80666=CARTESIAN_POINT('Ctrl Pts',(-0.237119375959961,0.00596467357892588,
-0.69628021117362));
#80667=CARTESIAN_POINT('Ctrl Pts',(-0.237176249981581,0.00293270419723155,
-0.696073195639592));
#80668=CARTESIAN_POINT('Ctrl Pts',(-0.237173375069643,-0.0039267215022098,
-0.695600864395705));
#80669=CARTESIAN_POINT('Ctrl Pts',(-0.237079128968467,-0.00775324162117441,
-0.695334562375428));
#80670=CARTESIAN_POINT('Ctrl Pts',(-0.236460123592357,-0.0204210329279014,
-0.694443552130688));
#80671=CARTESIAN_POINT('Ctrl Pts',(-0.23553286031713,-0.029234452003265,
-0.693808094571009));
#80672=CARTESIAN_POINT('Ctrl Pts',(-0.232027304357261,-0.0508463405152379,
-0.692219132727626));
#80673=CARTESIAN_POINT('Ctrl Pts',(-0.228881506087228,-0.0635238651221662,
-0.691259090747293));
#80674=CARTESIAN_POINT('Ctrl Pts',(-0.222895001689386,-0.0812525098720437,
-0.689915947723244));
#80675=CARTESIAN_POINT('Ctrl Pts',(-0.22088802153123,-0.0865600686243203,
-0.689514018016929));
#80676=CARTESIAN_POINT('Ctrl Pts',(-0.218096355597563,-0.0932112264920674,
-0.689014758242921));
#80677=CARTESIAN_POINT('Ctrl Pts',(-0.217486401012915,-0.0946256770487317,
-0.688908846944395));
#80678=CARTESIAN_POINT('Ctrl Pts',(-0.216491349620017,-0.096872685689174,
-0.68874112913286));
#80679=CARTESIAN_POINT('Ctrl Pts',(-0.216115140610536,-0.0977090976504158,
-0.68867881808495));
#80680=CARTESIAN_POINT('Ctrl Pts',(-0.215380602657762,-0.0993171707701197,
-0.688559279495476));
#80681=CARTESIAN_POINT('Ctrl Pts',(-0.215022961774339,-0.100089112015394,
-0.688502015529004));
#80682=CARTESIAN_POINT('Ctrl Pts',(-0.214140212545222,-0.101967890829651,
-0.688362901099698));
#80683=CARTESIAN_POINT('Ctrl Pts',(-0.213610658090264,-0.103072636042486,
-0.688281317520654));
#80684=CARTESIAN_POINT('Ctrl Pts',(-0.211649654915818,-0.10708360739301,
-0.687985729717637));
#80685=CARTESIAN_POINT('Ctrl Pts',(-0.21016719184699,-0.109964673282344,
-0.687774595004255));
#80686=CARTESIAN_POINT('Ctrl Pts',(-0.198457035282409,-0.131620056804292,
-0.68618981993618));
#80687=CARTESIAN_POINT('Ctrl Pts',(-0.185791137629021,-0.148966148066146,
-0.684925302574473));
#80688=CARTESIAN_POINT('Ctrl Pts',(-0.165144446418681,-0.170440453499752,
-0.683066374212442));
#80689=CARTESIAN_POINT('Ctrl Pts',(-0.159001190135598,-0.176185229856029,
-0.682533581290394));
#80690=CARTESIAN_POINT('Ctrl Pts',(-0.150610429427199,-0.183234838187202,
-0.681820936514482));
#80691=CARTESIAN_POINT('Ctrl Pts',(-0.148628041200286,-0.184846454987654,
-0.681653613557027));
#80692=CARTESIAN_POINT('Ctrl Pts',(-0.145360461258616,-0.187416341160832,
-0.681379252808125));
#80693=CARTESIAN_POINT('Ctrl Pts',(-0.144090873772623,-0.188394183864958,
-0.681272996589062));
#80694=CARTESIAN_POINT('Ctrl Pts',(-0.14161763865643,-0.190259457206785,
-0.681066605371749));
#80695=CARTESIAN_POINT('Ctrl Pts',(-0.14041531253571,-0.191148519388809,
-0.680966540739044));
#80696=CARTESIAN_POINT('Ctrl Pts',(-0.137581413691669,-0.193202885525309,
-0.680731266241497));
#80697=CARTESIAN_POINT('Ctrl Pts',(-0.135943333132698,-0.194358972308561,
-0.680595711665435));
#80698=CARTESIAN_POINT('Ctrl Pts',(-0.130460587147331,-0.198125236627198,
-0.680143331100566));
#80699=CARTESIAN_POINT('Ctrl Pts',(-0.126554091645045,-0.200643043347481,
-0.67982311295567));
#80700=CARTESIAN_POINT('Ctrl Pts',(-0.116868907982918,-0.20648991825204,
-0.679033770493161));
#80701=CARTESIAN_POINT('Ctrl Pts',(-0.111019142644893,-0.209693025059665,
-0.678560733097515));
#80702=CARTESIAN_POINT('Ctrl Pts',(-0.0963130041397121,-0.216957573281092,
-0.677382369391234));
#80703=CARTESIAN_POINT('Ctrl Pts',(-0.0873264861444057,-0.220727999368955,
-0.67667121862558));
#80704=CARTESIAN_POINT('Ctrl Pts',(-0.0767708078064536,-0.224411026785209,
-0.675855343415898));
#80705=CARTESIAN_POINT('Ctrl Pts',(-0.075403057561884,-0.224874286686873,
-0.675750002718781));
#80706=CARTESIAN_POINT('Ctrl Pts',(-0.063836581913,-0.228674484062525,-0.674862673465194));
#80707=CARTESIAN_POINT('Ctrl Pts',(-0.0534252491664702,-0.231328603825695,
-0.674086164177664));
#80708=CARTESIAN_POINT('Ctrl Pts',(-0.0411805023556501,-0.233578881526921,
-0.673221892608352));
#80709=CARTESIAN_POINT('Ctrl Pts',(-0.0394887006923036,-0.233870841732882,
-0.673103559393579));
#80710=CARTESIAN_POINT('Ctrl Pts',(-0.0368407293192654,-0.23429825721371,
-0.672920183032073));
#80711=CARTESIAN_POINT('Ctrl Pts',(-0.0358866887351938,-0.234446280253622,
-0.672854485188488));
#80712=CARTESIAN_POINT('Ctrl Pts',(-0.0341886597303467,-0.234699127815619,
-0.672738245038672));
#80713=CARTESIAN_POINT('Ctrl Pts',(-0.0334450657983187,-0.234806244908847,
-0.672687579562099));
#80714=CARTESIAN_POINT('Ctrl Pts',(-0.031639065265474,-0.235057651669759,
-0.67256508935813));
#80715=CARTESIAN_POINT('Ctrl Pts',(-0.030576172226623,-0.235198273509777,
-0.672493468784139));
#80716=CARTESIAN_POINT('Ctrl Pts',(-0.0272283710684135,-0.235618112574036,
-0.672269255998134));
#80717=CARTESIAN_POINT('Ctrl Pts',(-0.024940252569674,-0.235871286780743,
-0.672118019671748));
#80718=CARTESIAN_POINT('Ctrl Pts',(-0.0125357968794163,-0.237061271821679,
-0.67130720664883));
#80719=CARTESIAN_POINT('Ctrl Pts',(-0.00236979563541106,-0.237380756664839,
-0.670675071047823));
#80720=CARTESIAN_POINT('Ctrl Pts',(0.02667528972997,-0.236426702984017,
-0.668885040097899));
#80721=CARTESIAN_POINT('Ctrl Pts',(0.0454205656265901,-0.233551008332624,
-0.667743562940171));
#80722=CARTESIAN_POINT('Ctrl Pts',(0.067214476873861,-0.227482030501407,
-0.666289018797446));
#80723=CARTESIAN_POINT('Ctrl Pts',(0.0707792206248311,-0.226398232287836,
-0.666047108111816));
#80724=CARTESIAN_POINT('Ctrl Pts',(0.0760663453928736,-0.22465370204087,
-0.665681531292506));
#80725=CARTESIAN_POINT('Ctrl Pts',(0.0778090522498146,-0.224056077380419,
-0.66555991619019));
#80726=CARTESIAN_POINT('Ctrl Pts',(0.0809347093315071,-0.222943335459164,
-0.665339686154698));
#80727=CARTESIAN_POINT('Ctrl Pts',(0.0823201623337703,-0.222435493357917,
-0.665241315814294));
#80728=CARTESIAN_POINT('Ctrl Pts',(0.0852798943336163,-0.221319155664848,
-0.665029503822648));
#80729=CARTESIAN_POINT('Ctrl Pts',(0.0868525896664512,-0.220706720457173,
-0.664915935210272));
#80730=CARTESIAN_POINT('Ctrl Pts',(0.091161461730791,-0.218975583762136,
-0.664601894799887));
#80731=CARTESIAN_POINT('Ctrl Pts',(0.0938833887148409,-0.217822465192704,
-0.664400280638196));
#80732=CARTESIAN_POINT('Ctrl Pts',(0.0999136342908254,-0.215133784179527,
-0.663946145673182));
#80733=CARTESIAN_POINT('Ctrl Pts',(0.10320945973299,-0.213572199422351,
-0.663692800221025));
#80734=CARTESIAN_POINT('Ctrl Pts',(0.11378908353738,-0.208257419717737,
-0.662862591075651));
#80735=CARTESIAN_POINT('Ctrl Pts',(0.120914175099086,-0.204202958413524,
-0.662276542144161));
#80736=CARTESIAN_POINT('Ctrl Pts',(0.142297045516728,-0.190523261239037,
-0.660438921805837));
#80737=CARTESIAN_POINT('Ctrl Pts',(0.155729030114944,-0.179711021292023,
-0.659165269547456));
#80738=CARTESIAN_POINT('Ctrl Pts',(0.170111737662663,-0.165299756541713,
-0.657728510122017));
#80739=CARTESIAN_POINT('Ctrl Pts',(0.17230418013173,-0.163013142683692,
-0.657507333299815));
#80740=CARTESIAN_POINT('Ctrl Pts',(0.175296570385308,-0.159764368448068,
-0.657203212197398));
#80741=CARTESIAN_POINT('Ctrl Pts',(0.176135609654607,-0.158838874959991,
-0.657117684094636));
#80742=CARTESIAN_POINT('Ctrl Pts',(0.177531046905761,-0.157274997801759,
-0.656975071066078));
#80743=CARTESIAN_POINT('Ctrl Pts',(0.178091401725699,-0.156640193654241,
-0.656917701760471));
#80744=CARTESIAN_POINT('Ctrl Pts',(0.179244294060752,-0.15531994246384,
-0.656799479952646));
#80745=CARTESIAN_POINT('Ctrl Pts',(0.179836321832816,-0.154634080651831,
-0.656738663496734));
#80746=CARTESIAN_POINT('Ctrl Pts',(0.181391283892511,-0.15281165422978,
-0.656578589403994));
#80747=CARTESIAN_POINT('Ctrl Pts',(0.182347484216062,-0.151669360193929,
-0.656479804818328));
#80748=CARTESIAN_POINT('Ctrl Pts',(0.186916659113732,-0.146105263366896,
-0.656005629259628));
#80749=CARTESIAN_POINT('Ctrl Pts',(0.190380220469429,-0.141562596827126,
-0.655639608548447));
#80750=CARTESIAN_POINT('Ctrl Pts',(0.201233263612913,-0.126208338461148,
-0.654453832250033));
#80751=CARTESIAN_POINT('Ctrl Pts',(0.207892159793196,-0.11490980851155,
-0.653660126171383));
#80752=CARTESIAN_POINT('Ctrl Pts',(0.219333967335642,-0.0912109707662079,
-0.652041796883372));
#80753=CARTESIAN_POINT('Ctrl Pts',(0.224076500957956,-0.0788447051066105,
-0.651219416223988));
#80754=CARTESIAN_POINT('Ctrl Pts',(0.228538139955312,-0.0634823452933401,
-0.650181677229295));
#80755=CARTESIAN_POINT('Ctrl Pts',(0.229265604869487,-0.0608027215825348,
-0.650000171513463));
#80756=CARTESIAN_POINT('Ctrl Pts',(0.230350043845137,-0.0565115876114314,
-0.649708414154583));
#80757=CARTESIAN_POINT('Ctrl Pts',(0.230737541783148,-0.0549080031897362,
-0.649599144672579));
#80758=CARTESIAN_POINT('Ctrl Pts',(0.231441221123417,-0.051856887477658,
-0.649390721187275));
#80759=CARTESIAN_POINT('Ctrl Pts',(0.231760630050444,-0.0504101755747332,
-0.649291675901047));
#80760=CARTESIAN_POINT('Ctrl Pts',(0.232459409331316,-0.047098058220372,
-0.64906437461256));
#80761=CARTESIAN_POINT('Ctrl Pts',(0.232829913564717,-0.0452309082106214,
-0.648935843310124));
#80762=CARTESIAN_POINT('Ctrl Pts',(0.233919441232704,-0.0393716734037575,
-0.648531170491749));
#80763=CARTESIAN_POINT('Ctrl Pts',(0.23455852191895,-0.0353656605317828,
-0.648252548093306));
#80764=CARTESIAN_POINT('Ctrl Pts',(0.236472466262991,-0.0210108475294014,
-0.647246683151982));
#80765=CARTESIAN_POINT('Ctrl Pts',(0.237167278972143,-0.0105979302036642,
-0.646502588272292));
#80766=CARTESIAN_POINT('Ctrl Pts',(0.237188334714832,0.0180657516161505,
-0.644425580965743));
#80767=CARTESIAN_POINT('Ctrl Pts',(0.235097651825952,0.0362466276559837,
-0.643072523006146));
#80768=CARTESIAN_POINT('Ctrl Pts',(0.230437222458539,0.0561748729503284,
-0.641642806018916));
#80769=CARTESIAN_POINT('Ctrl Pts',(0.229900148569626,0.0583339731404771,
-0.641488710495671));
#80770=CARTESIAN_POINT('Ctrl Pts',(0.22906301165779,0.0615080160677536,
-0.641263682237236));
#80771=CARTESIAN_POINT('Ctrl Pts',(0.228786428497264,0.062528950040999,
-0.641191533018034));
#80772=CARTESIAN_POINT('Ctrl Pts',(0.228280681744097,0.0643474906123157,
-0.641063472246041));
#80773=CARTESIAN_POINT('Ctrl Pts',(0.228054152340937,0.0651457816736615,
-0.641007417178605));
#80774=CARTESIAN_POINT('Ctrl Pts',(0.22754206427591,0.0669149735573436,
-0.640883543102224));
#80775=CARTESIAN_POINT('Ctrl Pts',(0.227254477446639,0.0678852507958265,
-0.640815840694982));
#80776=CARTESIAN_POINT('Ctrl Pts',(0.22638298457389,0.0707579312079799,
-0.640616008007378));
#80777=CARTESIAN_POINT('Ctrl Pts',(0.22578132051995,0.0726549136375739,
-0.640484847731503));
#80778=CARTESIAN_POINT('Ctrl Pts',(0.221873288167833,0.0844588710812766,
-0.639672402924839));
#80779=CARTESIAN_POINT('Ctrl Pts',(0.217939021690352,0.0941471862273387,
-0.639021682597547));
#80780=CARTESIAN_POINT('Ctrl Pts',(0.205368938778352,0.120050599719358,
-0.637247352033516));
#80781=CARTESIAN_POINT('Ctrl Pts',(0.195472413233766,0.13556931214982,-0.636139691031507));
#80782=CARTESIAN_POINT('Ctrl Pts',(0.181484080917818,0.152741545198905,
-0.634721382224162));
#80783=CARTESIAN_POINT('Ctrl Pts',(0.179011082511387,0.155632519264186,
-0.634475376237373));
#80784=CARTESIAN_POINT('Ctrl Pts',(0.175210457091288,0.159865033102803,
-0.634103317586575));
#80785=CARTESIAN_POINT('Ctrl Pts',(0.173934535455955,0.16125231819046,-0.63397937597583));
#80786=CARTESIAN_POINT('Ctrl Pts',(0.171692310623751,0.163632669259151,
-0.633763121960138));
#80787=CARTESIAN_POINT('Ctrl Pts',(0.170733576172517,0.164632760426267,
-0.633671133465988));
#80788=CARTESIAN_POINT('Ctrl Pts',(0.168711424152924,0.166705480475458,
-0.633478062703468));
#80789=CARTESIAN_POINT('Ctrl Pts',(0.16764641503315,0.167776462011229,-0.633376913412475));
#80790=CARTESIAN_POINT('Ctrl Pts',(0.165079425871609,0.17030900047167,-0.633134331201958));
#80791=CARTESIAN_POINT('Ctrl Pts',(0.163568182593125,0.171760943294273,
-0.632992489780897));
#80792=CARTESIAN_POINT('Ctrl Pts',(0.158218673777876,0.176765910200489,
-0.6324936098271));
#80793=CARTESIAN_POINT('Ctrl Pts',(0.154282539011918,0.180211615868024,
-0.632132145934058));
#80794=CARTESIAN_POINT('Ctrl Pts',(0.144123526002445,0.188527954813937,
-0.631212341802383));
#80795=CARTESIAN_POINT('Ctrl Pts',(0.137765448175933,0.193222776378575,
-0.630648132597597));
#80796=CARTESIAN_POINT('Ctrl Pts',(0.118612623209255,0.205938788591801,
-0.628985964176629));
#80797=CARTESIAN_POINT('Ctrl Pts',(0.105272048381554,0.21306695670932,-0.627871504673812));
#80798=CARTESIAN_POINT('Ctrl Pts',(0.086527055803709,0.220889796031191,
-0.626417135630659));
#80799=CARTESIAN_POINT('Ctrl Pts',(0.0816438535334476,0.222740934141769,
-0.626048074958132));
#80800=CARTESIAN_POINT('Ctrl Pts',(0.0752866581696856,0.224913629020329,
-0.625583407315999));
#80801=CARTESIAN_POINT('Ctrl Pts',(0.0738655759217275,0.225384334859567,
-0.625480535055415));
#80802=CARTESIAN_POINT('Ctrl Pts',(0.0715758433478631,0.226118780816097,
-0.625316486020974));
#80803=CARTESIAN_POINT('Ctrl Pts',(0.0707099969692648,0.226391035129728,
-0.625254840991053));
#80804=CARTESIAN_POINT('Ctrl Pts',(0.0690247620257171,0.226910324144542,
-0.625135641701001));
#80805=CARTESIAN_POINT('Ctrl Pts',(0.0682055703903536,0.227157903607117,
-0.625078059468311));
#80806=CARTESIAN_POINT('Ctrl Pts',(0.0661844373101452,0.227756819698458,
-0.624936839032766));
#80807=CARTESIAN_POINT('Ctrl Pts',(0.0649809966951789,0.228103088320623,
-0.624853487470422));
#80808=CARTESIAN_POINT('Ctrl Pts',(0.0604674581817824,0.229363158416313,
-0.624543422911201));
#80809=CARTESIAN_POINT('Ctrl Pts',(0.0571402086120012,0.230214620378768,
-0.624319959093754));
#80810=CARTESIAN_POINT('Ctrl Pts',(0.0483776114019962,0.232255316823351,
-0.623741924689744));
#80811=CARTESIAN_POINT('Ctrl Pts',(0.0429167050884711,0.233326145086436,
-0.623392109630557));
#80812=CARTESIAN_POINT('Ctrl Pts',(0.0274435196089473,0.235798566131327,
-0.622417597690498));
#80813=CARTESIAN_POINT('Ctrl Pts',(0.017372204448269,0.236753730539024,
-0.621802360808144));
#80814=CARTESIAN_POINT('Ctrl Pts',(-0.00611972685676392,0.237474197682057,
-0.620357482006399));
#80815=CARTESIAN_POINT('Ctrl Pts',(-0.0195188929546864,0.236749640504096,
-0.619524916046828));
#80816=CARTESIAN_POINT('Ctrl Pts',(-0.0355422385575826,0.234513292344952,
-0.618475492117298));
#80817=CARTESIAN_POINT('Ctrl Pts',(-0.0382930840154859,0.234079844637703,
-0.61829346440237));
#80818=CARTESIAN_POINT('Ctrl Pts',(-0.0413357597826485,0.233545345668206,
-0.61808983353491));
#80819=CARTESIAN_POINT('Ctrl Pts',(-0.0416358457657131,0.233492033835083,
-0.618069725516726));
#80820=CARTESIAN_POINT('Ctrl Pts',(-0.0419358257187832,0.233438144154472,
-0.618049599588275));
#80821=CARTESIAN_POINT('Origin',(0.,0.,-1.7456589891905));
#80822=CARTESIAN_POINT('',(-0.0419358198037385,0.233438145217075,-0.498265075600824));
#80823=CARTESIAN_POINT('',(-0.0419358519811599,0.233438139436584,-0.517821408604163));
#80824=CARTESIAN_POINT('',(-0.0419358257166344,0.233438144154858,-1.7456589891905));
#80825=CARTESIAN_POINT('Ctrl Pts',(-0.0419358198037385,0.233438145217075,
-0.498265075600824));
#80826=CARTESIAN_POINT('Ctrl Pts',(-0.0375883549594239,0.234219142265114,
-0.498582125924067));
#80827=CARTESIAN_POINT('Ctrl Pts',(-0.0332186597349509,0.234878765261937,
-0.498896098541358));
#80828=CARTESIAN_POINT('Ctrl Pts',(-0.0265571725459339,0.235694609176903,
-0.499365299141105));
#80829=CARTESIAN_POINT('Ctrl Pts',(-0.024278510161308,0.23594021937747,
-0.499524127877175));
#80830=CARTESIAN_POINT('Ctrl Pts',(-0.0209307484076507,0.23625204797198,
-0.499754693432862));
#80831=CARTESIAN_POINT('Ctrl Pts',(-0.0198642672782424,0.236344108021554,
-0.499827730419059));
#80832=CARTESIAN_POINT('Ctrl Pts',(-0.0180482770250548,0.236488487485063,
-0.499951352910418));
#80833=CARTESIAN_POINT('Ctrl Pts',(-0.0172990963333227,0.23654447011165,
-0.500002136128038));
#80834=CARTESIAN_POINT('Ctrl Pts',(-0.01558486823416,0.236664378022562,
-0.500117833281334));
#80835=CARTESIAN_POINT('Ctrl Pts',(-0.0146196822255146,0.236725961645799,
-0.500182617302202));
#80836=CARTESIAN_POINT('Ctrl Pts',(-0.01193345735436,0.236880864072485,
-0.500361988976412));
#80837=CARTESIAN_POINT('Ctrl Pts',(-0.0102116975495199,0.236961331919338,
-0.500475897940956));
#80838=CARTESIAN_POINT('Ctrl Pts',(0.00296514757714645,0.237433270247909,
-0.501340594883976));
#80839=CARTESIAN_POINT('Ctrl Pts',(0.0144357251006429,0.23701272044814,
-0.50205289783394));
#80840=CARTESIAN_POINT('Ctrl Pts',(0.0345366386813281,0.234810301773894,
-0.503297368493959));
#80841=CARTESIAN_POINT('Ctrl Pts',(0.0431815134247895,0.233375263829393,
-0.503831327322732));
#80842=CARTESIAN_POINT('Ctrl Pts',(0.0592174646790345,0.229791597463751,
-0.504845784942641));
#80843=CARTESIAN_POINT('Ctrl Pts',(0.066621554414768,0.227755223370391,
-0.505324091005131));
#80844=CARTESIAN_POINT('Ctrl Pts',(0.0772386537588829,0.224273085124907,
-0.506034857091523));
#80845=CARTESIAN_POINT('Ctrl Pts',(0.0805390933980615,0.223109118840424,
-0.506259383769652));
#80846=CARTESIAN_POINT('Ctrl Pts',(0.086490611084208,0.220860930981155,
-0.506671717218466));
#80847=CARTESIAN_POINT('Ctrl Pts',(0.0891501328898553,0.21980088557117,
-0.506858740091548));
#80848=CARTESIAN_POINT('Ctrl Pts',(0.0933280935790383,0.218047313802549,
-0.50715729059242));
#80849=CARTESIAN_POINT('Ctrl Pts',(0.0948595716735321,0.217385430814567,
-0.507267753223869));
#80850=CARTESIAN_POINT('Ctrl Pts',(0.0977349915773449,0.216106544497265,
-0.50747715981706));
#80851=CARTESIAN_POINT('Ctrl Pts',(0.0990803997808114,0.215493019289291,
-0.50757598119883));
#80852=CARTESIAN_POINT('Ctrl Pts',(0.102116864171814,0.214073901072198,
-0.507800969348095));
#80853=CARTESIAN_POINT('Ctrl Pts',(0.10380427292183,0.213260783179708,-0.507927390576691));
#80854=CARTESIAN_POINT('Ctrl Pts',(0.108172770581271,0.211091588875938,
-0.508258407020709));
#80855=CARTESIAN_POINT('Ctrl Pts',(0.11083796344327,0.20970443871449,-0.508464065781227));
#80856=CARTESIAN_POINT('Ctrl Pts',(0.129099793055952,0.199754335158907,
-0.509899680948459));
#80857=CARTESIAN_POINT('Ctrl Pts',(0.143713405327172,0.189511966330684,
-0.511190243030281));
#80858=CARTESIAN_POINT('Ctrl Pts',(0.166277594503469,0.169574842144839,
-0.513388153288189));
#80859=CARTESIAN_POINT('Ctrl Pts',(0.174863980731367,0.1607062986969,-0.514286391851252));
#80860=CARTESIAN_POINT('Ctrl Pts',(0.184015391639358,0.149647676612415,
-0.515286755274764));
#80861=CARTESIAN_POINT('Ctrl Pts',(0.185288000276779,0.148069068725514,
-0.515426932016381));
#80862=CARTESIAN_POINT('Ctrl Pts',(0.187169976343504,0.1456723044142,-0.515635614672604));
#80863=CARTESIAN_POINT('Ctrl Pts',(0.187794529194794,0.144866266670738,
-0.515705104799717));
#80864=CARTESIAN_POINT('Ctrl Pts',(0.188917871590798,0.143397025590746,
-0.515830487131399));
#80865=CARTESIAN_POINT('Ctrl Pts',(0.189418393817325,0.142735213898974,
-0.515886494974548));
#80866=CARTESIAN_POINT('Ctrl Pts',(0.190544234189313,0.141230227953549,
-0.516012806368266));
#80867=CARTESIAN_POINT('Ctrl Pts',(0.191167438408812,0.140385515873453,
-0.516082966066488));
#80868=CARTESIAN_POINT('Ctrl Pts',(0.193068497315001,0.137772621171741,
-0.516297828033628));
#80869=CARTESIAN_POINT('Ctrl Pts',(0.194327622094212,0.135990867039419,
-0.516441330344064));
#80870=CARTESIAN_POINT('Ctrl Pts',(0.206000307951497,0.118979900380611,
-0.517785796782713));
#80871=CARTESIAN_POINT('Ctrl Pts',(0.214629547991921,0.102599713274845,
-0.518892390619855));
#80872=CARTESIAN_POINT('Ctrl Pts',(0.225780245552282,0.0737021693525357,
-0.520800049852848));
#80873=CARTESIAN_POINT('Ctrl Pts',(0.229354922309966,0.0616846028405787,
-0.52158114330555));
#80874=CARTESIAN_POINT('Ctrl Pts',(0.232530606303196,0.0467854239757479,
-0.522570002945124));
#80875=CARTESIAN_POINT('Ctrl Pts',(0.233051147508421,0.0441193882974078,
-0.522747659297159));
#80876=CARTESIAN_POINT('Ctrl Pts',(0.233811863977681,0.0398330684480232,
-0.52303471191078));
#80877=CARTESIAN_POINT('Ctrl Pts',(0.234081252256196,0.0382181657660059,
-0.523143182460735));
#80878=CARTESIAN_POINT('Ctrl Pts',(0.234563050249881,0.0351334762793155,
-0.523351049241446));
#80879=CARTESIAN_POINT('Ctrl Pts',(0.234778417793315,0.0336642252858814,
-0.523450346847231));
#80880=CARTESIAN_POINT('Ctrl Pts',(0.235237407553536,0.0303140205149874,
-0.523677470688439));
#80881=CARTESIAN_POINT('Ctrl Pts',(0.235472289624631,0.028431992692877,
-0.523805565071687));
#80882=CARTESIAN_POINT('Ctrl Pts',(0.236037995425773,0.0234097251846036,
-0.524148817374211));
#80883=CARTESIAN_POINT('Ctrl Pts',(0.236328712864905,0.0202654467845767,
-0.524365203284477));
#80884=CARTESIAN_POINT('Ctrl Pts',(0.238088962274773,-0.00406197373877007,
-0.526051507546298));
#80885=CARTESIAN_POINT('Ctrl Pts',(0.236769984116047,-0.0253471746040464,
-0.527610539026501));
#80886=CARTESIAN_POINT('Ctrl Pts',(0.231422192653109,-0.0522951858488935,
-0.529607266595906));
#80887=CARTESIAN_POINT('Ctrl Pts',(0.229964238286799,-0.058373595532827,
-0.530058198019026));
#80888=CARTESIAN_POINT('Ctrl Pts',(0.227581831603811,-0.066819727901037,
-0.530679967620756));
#80889=CARTESIAN_POINT('Ctrl Pts',(0.226856966191137,-0.0692407691678647,
-0.53085761864426));
#80890=CARTESIAN_POINT('Ctrl Pts',(0.225511066207966,-0.0734878010213719,
-0.531167711359621));
#80891=CARTESIAN_POINT('Ctrl Pts',(0.224906204401071,-0.0753186410947042,
-0.531300875005119));
#80892=CARTESIAN_POINT('Ctrl Pts',(0.223953934343624,-0.0780872277014383,
-0.531501251890974));
#80893=CARTESIAN_POINT('Ctrl Pts',(0.223622828849311,-0.0790304393703134,
-0.531569340514381));
#80894=CARTESIAN_POINT('Ctrl Pts',(0.223005606492748,-0.0807537642648298,
-0.531693384051082));
#80895=CARTESIAN_POINT('Ctrl Pts',(0.222721348406415,-0.0815344833431992,
-0.531749439668476));
#80896=CARTESIAN_POINT('Ctrl Pts',(0.222060425609967,-0.0833204675690925,
-0.531877364399071));
#80897=CARTESIAN_POINT('Ctrl Pts',(0.221681032699646,-0.084324686719036,
-0.53194907271531));
#80898=CARTESIAN_POINT('Ctrl Pts',(0.220464454834838,-0.0874798958991241,
-0.532173783637711));
#80899=CARTESIAN_POINT('Ctrl Pts',(0.219602653408803,-0.089621334609479,
-0.532325422142099));
#80900=CARTESIAN_POINT('Ctrl Pts',(0.21415101443046,-0.102616723749072,
-0.533242294387226));
#80901=CARTESIAN_POINT('Ctrl Pts',(0.208788204351879,-0.113130023458433,
-0.533970138933407));
#80902=CARTESIAN_POINT('Ctrl Pts',(0.196048695235886,-0.134086300132742,
-0.535476355091687));
#80903=CARTESIAN_POINT('Ctrl Pts',(0.188566378778727,-0.144419277645282,
-0.536252143095314));
#80904=CARTESIAN_POINT('Ctrl Pts',(0.175723333456434,-0.159444999330548,
-0.537494995589133));
#80905=CARTESIAN_POINT('Ctrl Pts',(0.170920926674716,-0.16458256349757,
-0.537943706370263));
#80906=CARTESIAN_POINT('Ctrl Pts',(0.164235279476827,-0.171126168016622,
-0.538553695224271));
#80907=CARTESIAN_POINT('Ctrl Pts',(0.162548954310412,-0.172728773598101,
-0.538706382941143));
#80908=CARTESIAN_POINT('Ctrl Pts',(0.159696518283608,-0.17536083056381,
-0.538962910933206));
#80909=CARTESIAN_POINT('Ctrl Pts',(0.15854334015026,-0.176404104110063,
-0.539066158197234));
#80910=CARTESIAN_POINT('Ctrl Pts',(0.156254269792768,-0.178434436354531,
-0.539270257360314));
#80911=CARTESIAN_POINT('Ctrl Pts',(0.15511907661864,-0.17942217475756,-0.539371074063216));
#80912=CARTESIAN_POINT('Ctrl Pts',(0.152341973058737,-0.181792494464919,
-0.539616795024525));
#80913=CARTESIAN_POINT('Ctrl Pts',(0.150690569890604,-0.183163695690997,
-0.539762153255346));
#80914=CARTESIAN_POINT('Ctrl Pts',(0.144971382117922,-0.187782782379225,
-0.540263138158497));
#80915=CARTESIAN_POINT('Ctrl Pts',(0.140815663005643,-0.190918874807781,
-0.540623091915124));
#80916=CARTESIAN_POINT('Ctrl Pts',(0.122462669202594,-0.203843535584079,
-0.542196497947033));
#80917=CARTESIAN_POINT('Ctrl Pts',(0.107325918587912,-0.212203385980076,
-0.543458867873501));
#80918=CARTESIAN_POINT('Ctrl Pts',(0.0848168176051991,-0.2216061768329,
-0.54523607730703));
#80919=CARTESIAN_POINT('Ctrl Pts',(0.078091824737247,-0.224064432010551,
-0.545754643894827));
#80920=CARTESIAN_POINT('Ctrl Pts',(0.0686417217721561,-0.227041543815893,
-0.546458452923269));
#80921=CARTESIAN_POINT('Ctrl Pts',(0.0660035482354762,-0.227822478254188,
-0.546652301406675));
#80922=CARTESIAN_POINT('Ctrl Pts',(0.0613696016778201,-0.229106930487794,
-0.546987550567844));
#80923=CARTESIAN_POINT('Ctrl Pts',(0.059379783949287,-0.229630693895293,
-0.547129836055955));
#80924=CARTESIAN_POINT('Ctrl Pts',(0.0563882120447176,-0.230376652416537,
-0.5473410078229));
#80925=CARTESIAN_POINT('Ctrl Pts',(0.0553914811282593,-0.230618334815579,
-0.547410912106422));
#80926=CARTESIAN_POINT('Ctrl Pts',(0.0535856686995562,-0.231043816251955,
-0.547536701953626));
#80927=CARTESIAN_POINT('Ctrl Pts',(0.0527771653459403,-0.231229841904709,
-0.547592707521551));
#80928=CARTESIAN_POINT('Ctrl Pts',(0.0509497327318144,-0.231640224902985,
-0.547718594588154));
#80929=CARTESIAN_POINT('Ctrl Pts',(0.049930283151621,-0.231862105539919,
-0.547788336837096));
#80930=CARTESIAN_POINT('Ctrl Pts',(0.046807390723548,-0.232520242965561,
-0.548000590780165));
#80931=CARTESIAN_POINT('Ctrl Pts',(0.0446993908286672,-0.232934669953599,
-0.548141944210076));
#80932=CARTESIAN_POINT('Ctrl Pts',(0.0274407459353899,-0.236084741458193,
-0.549285753559833));
#80933=CARTESIAN_POINT('Ctrl Pts',(0.0120601726350038,-0.237368245572755,
-0.550222132516388));
#80934=CARTESIAN_POINT('Ctrl Pts',(-0.0185666797360126,-0.236937158791131,
-0.552100953068818));
#80935=CARTESIAN_POINT('Ctrl Pts',(-0.0337373252665069,-0.235256567050508,
-0.553039736109136));
#80936=CARTESIAN_POINT('Ctrl Pts',(-0.0515073272439723,-0.231533045447863,
-0.554215673175061));
#80937=CARTESIAN_POINT('Ctrl Pts',(-0.0543619616769597,-0.230879474600708,
-0.554406876652346));
#80938=CARTESIAN_POINT('Ctrl Pts',(-0.0588362220554446,-0.229767511754084,
-0.554710558223767));
#80939=CARTESIAN_POINT('Ctrl Pts',(-0.060464379537721,-0.229344433212693,
-0.554821906503719));
#80940=CARTESIAN_POINT('Ctrl Pts',(-0.0635131079695817,-0.228517497157275,
-0.555032054984985));
#80941=CARTESIAN_POINT('Ctrl Pts',(-0.0649346817345278,-0.228117619507407,
-0.555130722334271));
#80942=CARTESIAN_POINT('Ctrl Pts',(-0.0681301118843269,-0.227186480843713,
-0.555354085823322));
#80943=CARTESIAN_POINT('Ctrl Pts',(-0.0699016497940442,-0.226647674248373,
-0.555479021931647));
#80944=CARTESIAN_POINT('Ctrl Pts',(-0.0744605875897065,-0.225202557562395,
-0.555803477752482));
#80945=CARTESIAN_POINT('Ctrl Pts',(-0.0772377498396402,-0.224265244087222,
-0.556003992587263));
#80946=CARTESIAN_POINT('Ctrl Pts',(-0.0974639087437562,-0.217018513151767,
-0.557486028829603));
#80947=CARTESIAN_POINT('Ctrl Pts',(-0.114133369744747,-0.208733253629731,
-0.558834304664219));
#80948=CARTESIAN_POINT('Ctrl Pts',(-0.139493979346946,-0.192175011021335,
-0.56104463700019));
#80949=CARTESIAN_POINT('Ctrl Pts',(-0.148835034916867,-0.185035115594045,
-0.561898553909415));
#80950=CARTESIAN_POINT('Ctrl Pts',(-0.15910640261384,-0.175900953603726,
-0.562856191099542));
#80951=CARTESIAN_POINT('Ctrl Pts',(-0.16058634673467,-0.174550905855101,
-0.562994642183365));
#80952=CARTESIAN_POINT('Ctrl Pts',(-0.162790040343816,-0.172488878325497,
-0.563201285045851));
#80953=CARTESIAN_POINT('Ctrl Pts',(-0.16352657188922,-0.171790776128469,
-0.563270433751032));
#80954=CARTESIAN_POINT('Ctrl Pts',(-0.164857309801192,-0.1705131574164,
-0.56339548399767));
#80955=CARTESIAN_POINT('Ctrl Pts',(-0.165452971114631,-0.169935234259086,
-0.563451497563454));
#80956=CARTESIAN_POINT('Ctrl Pts',(-0.166799058831083,-0.168615444085486,
-0.563578175788218));
#80957=CARTESIAN_POINT('Ctrl Pts',(-0.167547580644793,-0.167871684142795,
-0.563648692669994));
#80958=CARTESIAN_POINT('Ctrl Pts',(-0.16984864201145,-0.165554538270222,
-0.563865801583666));
#80959=CARTESIAN_POINT('Ctrl Pts',(-0.171384219948038,-0.163964375233955,
-0.564011157143056));
#80960=CARTESIAN_POINT('Ctrl Pts',(-0.182803540994591,-0.151803391812325,
-0.565097882627663));
#80961=CARTESIAN_POINT('Ctrl Pts',(-0.191724735420941,-0.140367884275242,
-0.565981452779055));
#80962=CARTESIAN_POINT('Ctrl Pts',(-0.208254055294894,-0.114637119904861,
-0.567856873775612));
#80963=CARTESIAN_POINT('Ctrl Pts',(-0.215555498941033,-0.100235534255107,
-0.568846493988605));
#80964=CARTESIAN_POINT('Ctrl Pts',(-0.222383403021873,-0.082498606103918,
-0.570077812052136));
#80965=CARTESIAN_POINT('Ctrl Pts',(-0.22337588701495,-0.0797722373792972,
-0.57026728620456));
#80966=CARTESIAN_POINT('Ctrl Pts',(-0.224862561752073,-0.0754428233801306,
-0.570568845477473));
#80967=CARTESIAN_POINT('Ctrl Pts',(-0.225390206946424,-0.0738515107999818,
-0.570679827795996));
#80968=CARTESIAN_POINT('Ctrl Pts',(-0.226351040965419,-0.0708475113464099,
-0.57088966596689));
#80969=CARTESIAN_POINT('Ctrl Pts',(-0.226787986780161,-0.0694361036690015,
-0.570988393188257));
#80970=CARTESIAN_POINT('Ctrl Pts',(-0.227745231768381,-0.0662385893067274,
-0.571212409527991));
#80971=CARTESIAN_POINT('Ctrl Pts',(-0.228257755312397,-0.0644502762147806,
-0.571337944457645));
#80972=CARTESIAN_POINT('Ctrl Pts',(-0.229531271061465,-0.0598008424156719,
-0.571665040179902));
#80973=CARTESIAN_POINT('Ctrl Pts',(-0.230259803064214,-0.0569312468706134,
-0.571867623375197));
#80974=CARTESIAN_POINT('Ctrl Pts',(-0.235097244188112,-0.0362623323546038,
-0.573332326245545));
#80975=CARTESIAN_POINT('Ctrl Pts',(-0.237190554660419,-0.0180574514021879,
-0.574658835074574));
#80976=CARTESIAN_POINT('Ctrl Pts',(-0.237172803082784,0.0026663364785689,
-0.576171385937248));
#80977=CARTESIAN_POINT('Ctrl Pts',(-0.237132321338845,0.0051293477589973,
-0.576351064670178));
#80978=CARTESIAN_POINT('Ctrl Pts',(-0.236734694563812,0.017546042617712,
-0.577255440399193));
#80979=CARTESIAN_POINT('Ctrl Pts',(-0.235789128579883,0.0274719871528137,
-0.577974166226661));
#80980=CARTESIAN_POINT('Ctrl Pts',(-0.233952710119945,0.0390005177114497,
-0.578784514752619));
#80981=CARTESIAN_POINT('Ctrl Pts',(-0.233665119673794,0.0406881214142345,
-0.578902505150956));
#80982=CARTESIAN_POINT('Ctrl Pts',(-0.233186958817902,0.0433215088412519,
-0.579085478400203));
#80983=CARTESIAN_POINT('Ctrl Pts',(-0.233008854426747,0.0442694559772227,
-0.579151111288395));
#80984=CARTESIAN_POINT('Ctrl Pts',(-0.2326816563759,0.0459542434779231,
-0.579267315044433));
#80985=CARTESIAN_POINT('Ctrl Pts',(-0.232534840653077,0.0466914725878568,
-0.579318008233905));
#80986=CARTESIAN_POINT('Ctrl Pts',(-0.232169692325919,0.0484806008444676,
-0.579440668495545));
#80987=CARTESIAN_POINT('Ctrl Pts',(-0.231947714701398,0.0495317317385739,
-0.579512430049519));
#80988=CARTESIAN_POINT('Ctrl Pts',(-0.2312254099009,0.0528406880505038,
-0.579737484619724));
#80989=CARTESIAN_POINT('Ctrl Pts',(-0.230699182093782,0.0550928021906593,
-0.579889407614677));
#80990=CARTESIAN_POINT('Ctrl Pts',(-0.227658898644796,0.0672959440329634,
-0.580707575322966));
#80991=CARTESIAN_POINT('Ctrl Pts',(-0.22453359798498,0.0770845605851778,
-0.581345831714881));
#80992=CARTESIAN_POINT('Ctrl Pts',(-0.21375521406658,0.104550703093417,
-0.583162756291909));
#80993=CARTESIAN_POINT('Ctrl Pts',(-0.20457470143206,0.121537112333389,
-0.584325100980924));
#80994=CARTESIAN_POINT('Ctrl Pts',(-0.191651140315015,0.139754857617948,
-0.58576478929569));
#80995=CARTESIAN_POINT('Ctrl Pts',(-0.189809237127245,0.142246377444869,
-0.585966163085969));
#80996=CARTESIAN_POINT('Ctrl Pts',(-0.186759815583291,0.146206575151737,
-0.586294037921658));
#80997=CARTESIAN_POINT('Ctrl Pts',(-0.185582484971241,0.147698111894396,
-0.58641937011502));
#80998=CARTESIAN_POINT('Ctrl Pts',(-0.183455545628686,0.15032710458339,
-0.586643690360722));
#80999=CARTESIAN_POINT('Ctrl Pts',(-0.182512950409314,0.151470123645603,
-0.586742394691361));
#81000=CARTESIAN_POINT('Ctrl Pts',(-0.180496528876385,0.153869146121517,
-0.586952110885188));
#81001=CARTESIAN_POINT('Ctrl Pts',(-0.179420165310126,0.155122903226704,
-0.587063223091992));
#81002=CARTESIAN_POINT('Ctrl Pts',(-0.176492976072893,0.15846129152175,
-0.587363245771734));
#81003=CARTESIAN_POINT('Ctrl Pts',(-0.17461840129346,0.160524653226724,
-0.58755313418008));
#81004=CARTESIAN_POINT('Ctrl Pts',(-0.162428734019602,0.173475716438283,
-0.588774350092515));
#81005=CARTESIAN_POINT('Ctrl Pts',(-0.151138614504918,0.183395445942116,
-0.589848317462613));
#81006=CARTESIAN_POINT('Ctrl Pts',(-0.12604326829651,0.20154493371799,-0.592103481063444));
#81007=CARTESIAN_POINT('Ctrl Pts',(-0.112182861796049,0.209576580361854,
-0.593281251479492));
#81008=CARTESIAN_POINT('Ctrl Pts',(-0.0957132382716444,0.217014586382776,
-0.594541671383385));
#81009=CARTESIAN_POINT('Ctrl Pts',(-0.0937957946198494,0.217850187839875,
-0.594686356036743));
#81010=CARTESIAN_POINT('Ctrl Pts',(-0.09091578846773,0.219060187155237,
-0.594900355020677));
#81011=CARTESIAN_POINT('Ctrl Pts',(-0.0899614857575037,0.219453816029182,
-0.594970726401677));
#81012=CARTESIAN_POINT('Ctrl Pts',(-0.0882356873261827,0.220152520494593,
-0.595096981663368));
#81013=CARTESIAN_POINT('Ctrl Pts',(-0.0874651348033049,0.220459790088123,
-0.595152990449377));
#81014=CARTESIAN_POINT('Ctrl Pts',(-0.0857283062017472,0.221141837221146,
-0.595278424542304));
#81015=CARTESIAN_POINT('Ctrl Pts',(-0.0847611708582154,0.22151433061782,
-0.595347715595423));
#81016=CARTESIAN_POINT('Ctrl Pts',(-0.0818154273540733,0.222626769923098,
-0.595557171993992));
#81017=CARTESIAN_POINT('Ctrl Pts',(-0.0798292863690017,0.223346655744975,
-0.595696222981916));
#81018=CARTESIAN_POINT('Ctrl Pts',(-0.0698910794199254,0.22679928795754,
-0.59638248911384));
#81019=CARTESIAN_POINT('Ctrl Pts',(-0.0618064595746589,0.229134613958218,
-0.596910738589662));
#81020=CARTESIAN_POINT('Ctrl Pts',(-0.0497394519529199,0.231934880622287,
-0.597678287747428));
#81021=CARTESIAN_POINT('Ctrl Pts',(-0.0458454425556047,0.232735804183639,
-0.597922824468853));
#81022=CARTESIAN_POINT('Ctrl Pts',(-0.041935808141222,0.233438147312179,
-0.598166693585938));
#81023=CARTESIAN_POINT('',(-0.23717495367369,-0.000148239275689535,-0.595517855191994));
#81024=CARTESIAN_POINT('Ctrl Pts',(-0.0419358257187832,0.233438144154472,
-0.618049599588275));
#81025=CARTESIAN_POINT('Ctrl Pts',(-0.043261267264733,0.233200036171422,
-0.617960674506957));
#81026=CARTESIAN_POINT('Ctrl Pts',(-0.0445846388219844,0.23295064713677,
-0.617871399567289));
#81027=CARTESIAN_POINT('Ctrl Pts',(-0.0473589822366303,0.232403316159762,
-0.617683176786025));
#81028=CARTESIAN_POINT('Ctrl Pts',(-0.0488094201177938,0.232103026471708,
-0.617584158513549));
#81029=CARTESIAN_POINT('Ctrl Pts',(-0.0521141759339126,0.231386483710759,
-0.617357098771406));
#81030=CARTESIAN_POINT('Ctrl Pts',(-0.0539664738729612,0.230961493565805,
-0.617228784121711));
#81031=CARTESIAN_POINT('Ctrl Pts',(-0.0597388950774482,0.229563842479385,
-0.616825521116593));
#81032=CARTESIAN_POINT('Ctrl Pts',(-0.0636392294354985,0.228513322098101,
-0.616548116573238));
#81033=CARTESIAN_POINT('Ctrl Pts',(-0.0769248959133572,0.224568437561562,
-0.615585648317777));
#81034=CARTESIAN_POINT('Ctrl Pts',(-0.0861553277255563,0.22119141263378,
-0.614885981884922));
#81035=CARTESIAN_POINT('Ctrl Pts',(-0.100117496526592,0.21507647180833,
-0.613783285543507));
#81036=CARTESIAN_POINT('Ctrl Pts',(-0.105009771953825,0.212730690667721,
-0.613388088063443));
#81037=CARTESIAN_POINT('Ctrl Pts',(-0.12167625656499,0.204024228059665,
-0.612015753684163));
#81038=CARTESIAN_POINT('Ctrl Pts',(-0.132990857487771,0.196836204636743,
-0.611036325282556));
#81039=CARTESIAN_POINT('Ctrl Pts',(-0.145416446004458,0.187379358035906,
-0.609945033831103));
#81040=CARTESIAN_POINT('Ctrl Pts',(-0.147174189294137,0.186001950225975,
-0.609790300561723));
#81041=CARTESIAN_POINT('Ctrl Pts',(-0.149748556034612,0.183925270150464,
-0.609563460954093));
#81042=CARTESIAN_POINT('Ctrl Pts',(-0.150580244910027,0.183244986260299,
-0.609490142375625));
#81043=CARTESIAN_POINT('Ctrl Pts',(-0.152046705492474,0.18202876153103,
-0.609360846359321));
#81044=CARTESIAN_POINT('Ctrl Pts',(-0.152683318982438,0.181495109714958,
-0.609304713393471));
#81045=CARTESIAN_POINT('Ctrl Pts',(-0.154044239389705,0.180342066894852,
-0.609184710844777));
#81046=CARTESIAN_POINT('Ctrl Pts',(-0.15476762772162,0.179721646635547,
-0.609120916605017));
#81047=CARTESIAN_POINT('Ctrl Pts',(-0.156777883706203,0.17797639435524,
-0.608943549582705));
#81048=CARTESIAN_POINT('Ctrl Pts',(-0.158056391158489,0.176841961628248,
-0.60883064551502));
#81049=CARTESIAN_POINT('Ctrl Pts',(-0.160996557754893,0.17417576066291,
-0.608570456465529));
#81050=CARTESIAN_POINT('Ctrl Pts',(-0.162648833598105,0.172633846474256,
-0.608423824387011));
#81051=CARTESIAN_POINT('Ctrl Pts',(-0.168069123482315,0.1674286847578,-0.60794038026738));
#81052=CARTESIAN_POINT('Ctrl Pts',(-0.171737599276426,0.163663675874433,
-0.607609183614968));
#81053=CARTESIAN_POINT('Ctrl Pts',(-0.182083974518938,0.152313710171214,
-0.606652077767214));
#81054=CARTESIAN_POINT('Ctrl Pts',(-0.188406023777705,0.144420304126392,
-0.606036742920574));
#81055=CARTESIAN_POINT('Ctrl Pts',(-0.202174241128331,0.124780841230472,
-0.604563286455234));
#81056=CARTESIAN_POINT('Ctrl Pts',(-0.209128574463145,0.112737973919794,
-0.603702134340606));
#81057=CARTESIAN_POINT('Ctrl Pts',(-0.216165652168537,0.0976327143499137,
-0.602621229964496));
#81058=CARTESIAN_POINT('Ctrl Pts',(-0.217297083025429,0.095087921094545,
-0.60243918985202));
#81059=CARTESIAN_POINT('Ctrl Pts',(-0.219027673533699,0.0910032215589308,
-0.602146776462821));
#81060=CARTESIAN_POINT('Ctrl Pts',(-0.219656025809943,0.0894759084946242,
-0.60203739326548));
#81061=CARTESIAN_POINT('Ctrl Pts',(-0.220817572614232,0.0865665880153049,
-0.60182888234272));
#81062=CARTESIAN_POINT('Ctrl Pts',(-0.221353872650469,0.0851858992293554,
-0.601729864704213));
#81063=CARTESIAN_POINT('Ctrl Pts',(-0.222548634272274,0.0820225412931475,
-0.601502810661118));
#81064=CARTESIAN_POINT('Ctrl Pts',(-0.223198665654398,0.080236819365599,
-0.601374501126548));
#81065=CARTESIAN_POINT('Ctrl Pts',(-0.225162848683154,0.0746323095690608,
-0.600971271365395));
#81066=CARTESIAN_POINT('Ctrl Pts',(-0.226400908304402,0.0707878190028559,
-0.600693895531664));
#81067=CARTESIAN_POINT('Ctrl Pts',(-0.230306603458723,0.0575065138158185,
-0.599732492157616));
#81068=CARTESIAN_POINT('Ctrl Pts',(-0.232486671899685,0.0479378456830597,
-0.599033915382798));
#81069=CARTESIAN_POINT('Ctrl Pts',(-0.236144099433985,0.025563921753949,
-0.597393894565987));
#81070=CARTESIAN_POINT('Ctrl Pts',(-0.237182995334464,0.0127179900854283,
-0.596446869367945));
#81071=CARTESIAN_POINT('Ctrl Pts',(-0.23717495367369,-0.000148239275689535,
-0.595517855191994));
#81072=CARTESIAN_POINT('Ctrl Pts',(-0.237174953469599,-0.000148565452673495,
-0.595517831640184));
#81073=CARTESIAN_POINT('Ctrl Pts',(-0.237170571033214,-0.00714483630179842,
-0.595012661700368));
#81074=CARTESIAN_POINT('Ctrl Pts',(-0.236856620653765,-0.0141383359309857,
-0.594513810019502));
#81075=CARTESIAN_POINT('Ctrl Pts',(-0.236127862419447,-0.0222941772729193,
-0.593946293421482));
#81076=CARTESIAN_POINT('Ctrl Pts',(-0.236012986451005,-0.023479099616672,
-0.593864197745905));
#81077=CARTESIAN_POINT('Ctrl Pts',(-0.235800019478486,-0.0255160103719254,
-0.593723742363697));
#81078=CARTESIAN_POINT('Ctrl Pts',(-0.235706221607482,-0.0263684114726592,
-0.593665166932078));
#81079=CARTESIAN_POINT('Ctrl Pts',(-0.235517961562506,-0.0279979134593863,
-0.593553600840225));
#81080=CARTESIAN_POINT('Ctrl Pts',(-0.235424270861452,-0.0287750957074899,
-0.593500569017096));
#81081=CARTESIAN_POINT('Ctrl Pts',(-0.235228397920248,-0.0303348688435763,
-0.593394513947027));
#81082=CARTESIAN_POINT('Ctrl Pts',(-0.235126155099939,-0.0311174338551282,
-0.593341493704201));
#81083=CARTESIAN_POINT('Ctrl Pts',(-0.234838181567596,-0.0332390836017287,
-0.593198226441276));
#81084=CARTESIAN_POINT('Ctrl Pts',(-0.234644901663677,-0.0345771389395796,
-0.593108390262976));
#81085=CARTESIAN_POINT('Ctrl Pts',(-0.233849768574976,-0.0397676971172572,
-0.592761656087875));
#81086=CARTESIAN_POINT('Ctrl Pts',(-0.233164356334744,-0.0436070071547999,
-0.592508950891954));
#81087=CARTESIAN_POINT('Ctrl Pts',(-0.230668938886948,-0.0558339063420614,
-0.591711224099113));
#81088=CARTESIAN_POINT('Ctrl Pts',(-0.228498361566743,-0.0641412995133093,
-0.591179800987735));
#81089=CARTESIAN_POINT('Ctrl Pts',(-0.220882056361195,-0.0879320307572641,
-0.589643286051157));
#81090=CARTESIAN_POINT('Ctrl Pts',(-0.214275964442334,-0.102988813273946,
-0.588649074421898));
#81091=CARTESIAN_POINT('Ctrl Pts',(-0.203718441821695,-0.121553967374537,
-0.587288910779183));
#81092=CARTESIAN_POINT('Ctrl Pts',(-0.201132701741115,-0.125786331973154,
-0.586969194049667));
#81093=CARTESIAN_POINT('Ctrl Pts',(-0.197290780904103,-0.131653141390029,
-0.586510260190062));
#81094=CARTESIAN_POINT('Ctrl Pts',(-0.196142947705431,-0.133357210134684,
-0.586375013184672));
#81095=CARTESIAN_POINT('Ctrl Pts',(-0.194117171488417,-0.136281929510222,
-0.586139366362959));
#81096=CARTESIAN_POINT('Ctrl Pts',(-0.193249479894379,-0.137509559381093,
-0.58603935737916));
#81097=CARTESIAN_POINT('Ctrl Pts',(-0.191443371428481,-0.140014023842918,
-0.585833013704774));
#81098=CARTESIAN_POINT('Ctrl Pts',(-0.190503713741527,-0.141289865796199,
-0.585726634623225));
#81099=CARTESIAN_POINT('Ctrl Pts',(-0.188066892970437,-0.144530011031782,
-0.585453163990089));
#81100=CARTESIAN_POINT('Ctrl Pts',(-0.186551734289412,-0.14648047635436,
-0.585285376165629));
#81101=CARTESIAN_POINT('Ctrl Pts',(-0.180149392728657,-0.154461740881651,
-0.584585270508451));
#81102=CARTESIAN_POINT('Ctrl Pts',(-0.174998554358182,-0.160273877673241,
-0.584042574976139));
#81103=CARTESIAN_POINT('Ctrl Pts',(-0.15820562877943,-0.177446567665429,
-0.5823334956234));
#81104=CARTESIAN_POINT('Ctrl Pts',(-0.145674155830269,-0.187870316300923,
-0.581135934635838));
#81105=CARTESIAN_POINT('Ctrl Pts',(-0.127503371734501,-0.200066379325894,
-0.579549088820918));
#81106=CARTESIAN_POINT('Ctrl Pts',(-0.122719064259667,-0.203036216333502,
-0.579144104826531));
#81107=CARTESIAN_POINT('Ctrl Pts',(-0.114829122977856,-0.207552971986113,
-0.57850127846909));
#81108=CARTESIAN_POINT('Ctrl Pts',(-0.111787426958215,-0.209206926019219,
-0.578259212400673));
#81109=CARTESIAN_POINT('Ctrl Pts',(-0.107594141871095,-0.211369483997706,
-0.577934308234557));
#81110=CARTESIAN_POINT('Ctrl Pts',(-0.106473272205527,-0.211936312630657,
-0.577848302430748));
#81111=CARTESIAN_POINT('Ctrl Pts',(-0.104580572317317,-0.212874653421189,
-0.577704547922996));
#81112=CARTESIAN_POINT('Ctrl Pts',(-0.103811146385501,-0.213250932359655,
-0.577646514890303));
#81113=CARTESIAN_POINT('Ctrl Pts',(-0.10222329911387,-0.214016820054254,
-0.577527611243384));
#81114=CARTESIAN_POINT('Ctrl Pts',(-0.101404657674275,-0.214405917873048,
-0.577466770938083));
#81115=CARTESIAN_POINT('Ctrl Pts',(-0.0992332517249813,-0.215422761814901,
-0.577306562351128));
#81116=CARTESIAN_POINT('Ctrl Pts',(-0.0978767371693001,-0.216042470729354,
-0.577207668544413));
#81117=CARTESIAN_POINT('Ctrl Pts',(-0.0918028108879673,-0.218748324530533,
-0.576769754274855));
#81118=CARTESIAN_POINT('Ctrl Pts',(-0.0870235789505664,-0.220693205908022,
-0.576438245038698));
#81119=CARTESIAN_POINT('Ctrl Pts',(-0.0680042510002974,-0.227718939208846,
-0.575155353259361));
#81120=CARTESIAN_POINT('Ctrl Pts',(-0.0533549519811368,-0.231589740948118,
-0.574243803806477));
#81121=CARTESIAN_POINT('Ctrl Pts',(-0.0306124204402045,-0.235324710741681,
-0.572822317099033));
#81122=CARTESIAN_POINT('Ctrl Pts',(-0.0227298134306724,-0.23621638676001,
-0.572328895185088));
#81123=CARTESIAN_POINT('Ctrl Pts',(-0.0095847230980491,-0.237039250280026,
-0.571491733839251));
#81124=CARTESIAN_POINT('Ctrl Pts',(-0.00434255531961072,-0.237193188926543,
-0.571154175118985));
#81125=CARTESIAN_POINT('Ctrl Pts',(0.0029977252870206,-0.23716533111237,
-0.570674104885457));
#81126=CARTESIAN_POINT('Ctrl Pts',(0.00509507551264766,-0.237129543453933,
-0.570536093177132));
#81127=CARTESIAN_POINT('Ctrl Pts',(0.00870164498915564,-0.237020134735887,
-0.570297193966059));
#81128=CARTESIAN_POINT('Ctrl Pts',(0.0102111662738607,-0.236959901248115,
-0.570196727977712));
#81129=CARTESIAN_POINT('Ctrl Pts',(0.0132890723122393,-0.236807620780158,
-0.569990860649144));
#81130=CARTESIAN_POINT('Ctrl Pts',(0.0148573210608145,-0.236714402832266,
-0.569885427695738));
#81131=CARTESIAN_POINT('Ctrl Pts',(0.018823949479914,-0.236439050647876,
-0.569617330492226));
#81132=CARTESIAN_POINT('Ctrl Pts',(0.0212206502947203,-0.236236002773485,
-0.569454022828449));
#81133=CARTESIAN_POINT('Ctrl Pts',(0.0307360445602773,-0.235283894054256,
-0.56880018671674));
#81134=CARTESIAN_POINT('Ctrl Pts',(0.0378216918353701,-0.23424926143078,
-0.568300944889594));
#81135=CARTESIAN_POINT('Ctrl Pts',(0.0600180576564708,-0.229974873993864,
-0.566697618462069));
#81136=CARTESIAN_POINT('Ctrl Pts',(0.0748641676677131,-0.225578977197656,
-0.565563841336754));
#81137=CARTESIAN_POINT('Ctrl Pts',(0.0953396875244777,-0.217270745662714,
-0.563955934867405));
#81138=CARTESIAN_POINT('Ctrl Pts',(0.101396255566271,-0.214511173094511,
-0.56347492500311));
#81139=CARTESIAN_POINT('Ctrl Pts',(0.109673318024955,-0.210310851647791,
-0.562816505942914));
#81140=CARTESIAN_POINT('Ctrl Pts',(0.111997678700695,-0.209082309646988,
-0.562631500235571));
#81141=CARTESIAN_POINT('Ctrl Pts',(0.116042399495685,-0.20685765861291,
-0.562309958084017));
#81142=CARTESIAN_POINT('Ctrl Pts',(0.117771533730135,-0.205878109318699,
-0.562172627484544));
#81143=CARTESIAN_POINT('Ctrl Pts',(0.120361894354139,-0.204367360289341,
-0.56196732250584));
#81144=CARTESIAN_POINT('Ctrl Pts',(0.121232319573422,-0.203852221841296,
-0.561898408625373));
#81145=CARTESIAN_POINT('Ctrl Pts',(0.122810871420843,-0.202904310265034,
-0.561773602227446));
#81146=CARTESIAN_POINT('Ctrl Pts',(0.123520040234958,-0.202473378419569,
-0.561717600021444));
#81147=CARTESIAN_POINT('Ctrl Pts',(0.125128531446269,-0.201484369996454,
-0.561590723830709));
#81148=CARTESIAN_POINT('Ctrl Pts',(0.126026395111273,-0.200923987061535,
-0.561520000033162));
#81149=CARTESIAN_POINT('Ctrl Pts',(0.128802767844681,-0.199165238637102,
-0.561301517375187));
#81150=CARTESIAN_POINT('Ctrl Pts',(0.130668224430713,-0.197946359622002,
-0.561155017910066));
#81151=CARTESIAN_POINT('Ctrl Pts',(0.144398683263895,-0.188696245190025,
-0.560076776764178));
#81152=CARTESIAN_POINT('Ctrl Pts',(0.15553291219144,-0.179629829442218,
-0.559201530061659));
#81153=CARTESIAN_POINT('Ctrl Pts',(0.168966584928727,-0.166499574943449,
-0.55804959600846));
#81154=CARTESIAN_POINT('Ctrl Pts',(0.172063182665283,-0.16329750678787,
-0.557776502456426));
#81155=CARTESIAN_POINT('Ctrl Pts',(0.180518784697646,-0.154046200394293,
-0.557003911623883));
#81156=CARTESIAN_POINT('Ctrl Pts',(0.185661164826487,-0.14780791880536,
-0.556501472186896));
#81157=CARTESIAN_POINT('Ctrl Pts',(0.193639478498566,-0.137054513971805,
-0.555650774396388));
#81158=CARTESIAN_POINT('Ctrl Pts',(0.196659656027989,-0.132684439403903,
-0.555308976907627));
#81159=CARTESIAN_POINT('Ctrl Pts',(0.200669800806683,-0.126443874884412,
-0.554823898612598));
#81160=CARTESIAN_POINT('Ctrl Pts',(0.201785435705773,-0.124655765678032,
-0.554685248479597));
#81161=CARTESIAN_POINT('Ctrl Pts',(0.2036605072712,-0.121559310652525,-0.554445594362856));
#81162=CARTESIAN_POINT('Ctrl Pts',(0.204431540988378,-0.120258110317989,
-0.55434501904546));
#81163=CARTESIAN_POINT('Ctrl Pts',(0.205976522316863,-0.117592992638369,
-0.554139241449768));
#81164=CARTESIAN_POINT('Ctrl Pts',(0.206749491963677,-0.116228598168285,
-0.554034010386121));
#81165=CARTESIAN_POINT('Ctrl Pts',(0.208666928367412,-0.112764410568471,
-0.553767065634044));
#81166=CARTESIAN_POINT('Ctrl Pts',(0.209793249284913,-0.110654828689662,
-0.553604719697252));
#81167=CARTESIAN_POINT('Ctrl Pts',(0.214102231794804,-0.102281828780174,
-0.552960986520942));
#81168=CARTESIAN_POINT('Ctrl Pts',(0.217037558936247,-0.0958958745226785,
-0.552471232167991));
#81169=CARTESIAN_POINT('Ctrl Pts',(0.225549943492971,-0.0749757395474853,
-0.550870359882693));
#81170=CARTESIAN_POINT('Ctrl Pts',(0.22998163644367,-0.0600207486190322,
-0.549728371006473));
#81171=CARTESIAN_POINT('Ctrl Pts',(0.234177667245787,-0.0381770367935283,
-0.548109687204103));
#81172=CARTESIAN_POINT('Ctrl Pts',(0.235160681997152,-0.031561539969732,
-0.547626259335225));
#81173=CARTESIAN_POINT('Ctrl Pts',(0.236139905032703,-0.0222907727159821,
-0.546964905663577));
#81174=CARTESIAN_POINT('Ctrl Pts',(0.236373139771617,-0.0196640111848082,
-0.546779319352579));
#81175=CARTESIAN_POINT('Ctrl Pts',(0.236705579665014,-0.015047140340816,
-0.546456875225081));
#81176=CARTESIAN_POINT('Ctrl Pts',(0.236823603878279,-0.0130586819255909,
-0.546319217429605));
#81177=CARTESIAN_POINT('Ctrl Pts',(0.236963813573957,-0.0100576591424868,
-0.546113525185883));
#81178=CARTESIAN_POINT('Ctrl Pts',(0.237004585284174,-0.00904610966653566,
-0.546044546128703));
#81179=CARTESIAN_POINT('Ctrl Pts',(0.237066989210801,-0.00720498548137484,
-0.545919677059108));
#81180=CARTESIAN_POINT('Ctrl Pts',(0.237090745836903,-0.0063755370884557,
-0.545863676665504));
#81181=CARTESIAN_POINT('Ctrl Pts',(0.237134872344849,-0.00448895970372778,
-0.545736873689137));
#81182=CARTESIAN_POINT('Ctrl Pts',(0.237152527466102,-0.00343180186491667,
-0.545666220519968));
#81183=CARTESIAN_POINT('Ctrl Pts',(0.23718536327195,-0.000152238589986392,
-0.545448185140647));
#81184=CARTESIAN_POINT('Ctrl Pts',(0.237176377841256,0.00207036045988246,
-0.545302054945404));
#81185=CARTESIAN_POINT('Ctrl Pts',(0.236805863563745,0.0225386779013626,
-0.543968670879194));
#81186=CARTESIAN_POINT('Ctrl Pts',(0.234370786503552,0.0406882938431326,
-0.542873267876422));
#81187=CARTESIAN_POINT('Ctrl Pts',(0.226764188929052,0.0706395626200742,
-0.540970577724566));
#81188=CARTESIAN_POINT('Ctrl Pts',(0.222675799951735,0.0826279229933428,
-0.540181913606909));
#81189=CARTESIAN_POINT('Ctrl Pts',(0.216570648452122,0.0967291974654365,
-0.539184515668556));
#81190=CARTESIAN_POINT('Ctrl Pts',(0.215446794278926,0.0992071633394274,
-0.539006569644532));
#81191=CARTESIAN_POINT('Ctrl Pts',(0.213578524376315,0.103144932803993,
-0.538719181810877));
#81192=CARTESIAN_POINT('Ctrl Pts',(0.212861157193617,0.104617354055069,
-0.538610670091569));
#81193=CARTESIAN_POINT('Ctrl Pts',(0.2114647565378,0.107409684363715,-0.538402811921996));
#81194=CARTESIAN_POINT('Ctrl Pts',(0.210788467752124,0.108730884496113,
-0.538303564940414));
#81195=CARTESIAN_POINT('Ctrl Pts',(0.209221111752811,0.111723290956537,
-0.53807667978722));
#81196=CARTESIAN_POINT('Ctrl Pts',(0.208322347445643,0.113390328241956,
-0.537948775078477));
#81197=CARTESIAN_POINT('Ctrl Pts',(0.205406906734066,0.118646237104622,
-0.537540588909763));
#81198=CARTESIAN_POINT('Ctrl Pts',(0.203316807541324,0.122193285513064,
-0.53725772417659));
#81199=CARTESIAN_POINT('Ctrl Pts',(0.191353001000619,0.141339300531332,
-0.535688868771899));
#81200=CARTESIAN_POINT('Ctrl Pts',(0.179777465363339,0.155796684328052,
-0.534340476054183));
#81201=CARTESIAN_POINT('Ctrl Pts',(0.159516208535676,0.175803767857263,
-0.532264712286895));
#81202=CARTESIAN_POINT('Ctrl Pts',(0.151946522763103,0.182386070587964,
-0.531538773433789));
#81203=CARTESIAN_POINT('Ctrl Pts',(0.142164478862654,0.189859093628788,
-0.530678194329031));
#81204=CARTESIAN_POINT('Ctrl Pts',(0.140326431730872,0.191221620126433,
-0.530519639398288));
#81205=CARTESIAN_POINT('Ctrl Pts',(0.137600564696794,0.193181803138787,
-0.530289405587618));
#81206=CARTESIAN_POINT('Ctrl Pts',(0.136728020222686,0.193800343306433,
-0.530216431323708));
#81207=CARTESIAN_POINT('Ctrl Pts',(0.135235727363386,0.194843123120728,
-0.530092891104572));
#81208=CARTESIAN_POINT('Ctrl Pts',(0.134618110535349,0.195270348380001,
-0.530042127949405));
#81209=CARTESIAN_POINT('Ctrl Pts',(0.133200402178315,0.196241099073671,
-0.529926445585333));
#81210=CARTESIAN_POINT('Ctrl Pts',(0.132399004028769,0.196782671800986,
-0.529861656500242));
#81211=CARTESIAN_POINT('Ctrl Pts',(0.130159456182275,0.19827624930605,-0.529682205389604));
#81212=CARTESIAN_POINT('Ctrl Pts',(0.12871416865677,0.199217515003067,-0.529568223258868));
#81213=CARTESIAN_POINT('Ctrl Pts',(0.117527278183369,0.206330575616943,
-0.528698854616319));
#81214=CARTESIAN_POINT('Ctrl Pts',(0.107356168235146,0.211801066195356,
-0.527982430923913));
#81215=CARTESIAN_POINT('Ctrl Pts',(0.0963342165446225,0.216730223379704,
-0.527239474662252));
#81216=CARTESIAN_POINT('Ctrl Pts',(0.0958415504323145,0.216948538175205,
-0.527206333863953));
#81217=CARTESIAN_POINT('Ctrl Pts',(0.0867021829958203,0.220961252137059,
-0.526592741027069));
#81218=CARTESIAN_POINT('Ctrl Pts',(0.0778373824196349,0.224237557498435,
-0.526017005720486));
#81219=CARTESIAN_POINT('Ctrl Pts',(0.0622043465669194,0.228976228976599,
-0.525004832202367));
#81220=CARTESIAN_POINT('Ctrl Pts',(0.0555241199896826,0.230687138434034,
-0.524573342802406));
#81221=CARTESIAN_POINT('Ctrl Pts',(0.0441227348075537,0.233083258425263,
-0.523830302763292));
#81222=CARTESIAN_POINT('Ctrl Pts',(0.0394381383633985,0.233921459956155,
-0.523523191092661));
#81223=CARTESIAN_POINT('Ctrl Pts',(0.0327306075814457,0.234914410486938,
-0.52307924688592));
#81224=CARTESIAN_POINT('Ctrl Pts',(0.0307258166930042,0.235185026514933,
-0.522946030726012));
#81225=CARTESIAN_POINT('Ctrl Pts',(0.0272307318153744,0.235611358650051,
-0.522712753333736));
#81226=CARTESIAN_POINT('Ctrl Pts',(0.0257419485388233,0.235778661015362,
-0.522613060676727));
#81227=CARTESIAN_POINT('Ctrl Pts',(0.0228563769567727,0.236075272275144,
-0.522419163805604));
#81228=CARTESIAN_POINT('Ctrl Pts',(0.0214598268016012,0.236206316246989,
-0.522325018369448));
#81229=CARTESIAN_POINT('Ctrl Pts',(0.0177264699098827,0.236523250326617,
-0.522072490182803));
#81230=CARTESIAN_POINT('Ctrl Pts',(0.015387982503259,0.236686892306821,
-0.521913421021383));
#81231=CARTESIAN_POINT('Ctrl Pts',(0.00647182722471014,0.237178133753775,
-0.521303332392777));
#81232=CARTESIAN_POINT('Ctrl Pts',(-0.000115500270155912,0.237266356424297,
-0.520845047669498));
#81233=CARTESIAN_POINT('Ctrl Pts',(-0.0185264746784814,0.23674625214578,
-0.519542729368853));
#81234=CARTESIAN_POINT('Ctrl Pts',(-0.0303055268150793,0.235527462097546,
-0.518683880692026));
#81235=CARTESIAN_POINT('Ctrl Pts',(-0.0419358519811635,0.233438139436584,
-0.517821408604163));
#81236=CARTESIAN_POINT('Origin',(0.,0.,-1.7456589891905));
#81237=CARTESIAN_POINT('',(-0.0419358190075303,0.23343814536011,-0.397909151625197));
#81238=CARTESIAN_POINT('',(-0.0419358280420692,0.233438143737107,-0.417646538149483));
#81239=CARTESIAN_POINT('',(-0.0419358257166344,0.233438144154858,-1.7456589891905));
#81240=CARTESIAN_POINT('',(-0.237174999766729,1.05191258440349E-5,-0.475718588717799));
#81241=CARTESIAN_POINT('Ctrl Pts',(-0.0419358190075306,0.23343814536011,
-0.397909151625197));
#81242=CARTESIAN_POINT('Ctrl Pts',(-0.0317267657812627,0.235272143002931,
-0.398629247492366));
#81243=CARTESIAN_POINT('Ctrl Pts',(-0.0214074572156793,0.236434631915132,
-0.399369272295089));
#81244=CARTESIAN_POINT('Ctrl Pts',(0.00738320527071984,0.237776723418298,
-0.401457010517832));
#81245=CARTESIAN_POINT('Ctrl Pts',(0.0258479393168837,0.236483004057781,
-0.402826067786711));
#81246=CARTESIAN_POINT('Ctrl Pts',(0.0461210455182574,0.232657672366057,
-0.404266587768362));
#81247=CARTESIAN_POINT('Ctrl Pts',(0.0482599787164858,0.232223423984624,
-0.404417693361836));
#81248=CARTESIAN_POINT('Ctrl Pts',(0.0514185785498025,0.231536633337051,
-0.4046392343386));
#81249=CARTESIAN_POINT('Ctrl Pts',(0.0524429840939502,0.23130675805443,
-0.404710834404866));
#81250=CARTESIAN_POINT('Ctrl Pts',(0.0542742712242867,0.230883028039117,
-0.404838340543364));
#81251=CARTESIAN_POINT('Ctrl Pts',(0.0550816961518037,0.230691733626287,
-0.404894384312414));
#81252=CARTESIAN_POINT('Ctrl Pts',(0.0568789448163363,0.230255956854864,
-0.405018744253081));
#81253=CARTESIAN_POINT('Ctrl Pts',(0.0578682115086129,0.230009326383489,
-0.405086938427213));
#81254=CARTESIAN_POINT('Ctrl Pts',(0.0608192982060854,0.22925335673267,
-0.405289682272511));
#81255=CARTESIAN_POINT('Ctrl Pts',(0.062776269233406,0.228725226637899,
-0.405423219512599));
#81256=CARTESIAN_POINT('Ctrl Pts',(0.0765161741268056,0.224827583118753,
-0.406355925518777));
#81257=CARTESIAN_POINT('Ctrl Pts',(0.0880307032054034,0.220573889043712,
-0.407112816160427));
#81258=CARTESIAN_POINT('Ctrl Pts',(0.115402750124721,0.207975163111058,
-0.408963351674379));
#81259=CARTESIAN_POINT('Ctrl Pts',(0.130740838185398,0.198691268582307,
-0.410050228211231));
#81260=CARTESIAN_POINT('Ctrl Pts',(0.147263095680553,0.185942314809714,
-0.411396725322285));
#81261=CARTESIAN_POINT('Ctrl Pts',(0.149600985678177,0.184066584642513,
-0.411591683826283));
#81262=CARTESIAN_POINT('Ctrl Pts',(0.153339512501802,0.180948819037631,
-0.411911170446299));
#81263=CARTESIAN_POINT('Ctrl Pts',(0.154762137032554,0.1797335856563,-0.412034627183156));
#81264=CARTESIAN_POINT('Ctrl Pts',(0.157282935565084,0.177528151940406,
-0.412256879616822));
#81265=CARTESIAN_POINT('Ctrl Pts',(0.158386519553255,0.176544263022267,
-0.412355411462506));
#81266=CARTESIAN_POINT('Ctrl Pts',(0.160716663593573,0.174427413304002,
-0.412566143884982));
#81267=CARTESIAN_POINT('Ctrl Pts',(0.161940597171378,0.173291694000308,
-0.412678457851815));
#81268=CARTESIAN_POINT('Ctrl Pts',(0.165234778927277,0.170169562049885,
-0.412985272807564));
#81269=CARTESIAN_POINT('Ctrl Pts',(0.167281080933843,0.168158409614102,
-0.413180829833688));
#81270=CARTESIAN_POINT('Ctrl Pts',(0.171747995182962,0.163605991729049,
-0.41361913320721));
#81271=CARTESIAN_POINT('Ctrl Pts',(0.17414966057941,0.161047160453219,-0.413862619142252));
#81272=CARTESIAN_POINT('Ctrl Pts',(0.181643002601502,0.152699778260872,
-0.414648040684364));
#81273=CARTESIAN_POINT('Ctrl Pts',(0.18650925610152,0.146716327730293,-0.415198089982703));
#81274=CARTESIAN_POINT('Ctrl Pts',(0.196371682246179,0.133304439355165,
-0.416400678330391));
#81275=CARTESIAN_POINT('Ctrl Pts',(0.201256497807493,0.125808279816814,
-0.417054690773567));
#81276=CARTESIAN_POINT('Ctrl Pts',(0.211296143348545,0.108314521535111,
-0.418525580639704));
#81277=CARTESIAN_POINT('Ctrl Pts',(0.21618776935157,0.0981885952475901,
-0.419339669702313));
#81278=CARTESIAN_POINT('Ctrl Pts',(0.220980133269461,0.0861552067457863,
-0.420238886342993));
#81279=CARTESIAN_POINT('Ctrl Pts',(0.221599135776701,0.0845503542282169,
-0.420357450220177));
#81280=CARTESIAN_POINT('Ctrl Pts',(0.222538565721099,0.0820335369102421,
-0.420541116925352));
#81281=CARTESIAN_POINT('Ctrl Pts',(0.222870956498742,0.0811261440211782,
-0.420606877422912));
#81282=CARTESIAN_POINT('Ctrl Pts',(0.223451938448637,0.0795095996800856,
-0.420723188858775));
#81283=CARTESIAN_POINT('Ctrl Pts',(0.223702709728511,0.0788012875589661,
-0.420773863502451));
#81284=CARTESIAN_POINT('Ctrl Pts',(0.224302944833988,0.0770799443931066,
-0.420896327160993));
#81285=CARTESIAN_POINT('Ctrl Pts',(0.224648915304766,0.0760657206086813,
-0.420967912487646));
#81286=CARTESIAN_POINT('Ctrl Pts',(0.225715133389289,0.0728693320672463,
-0.421191830837947));
#81287=CARTESIAN_POINT('Ctrl Pts',(0.226410573852171,0.0706789502045201,
-0.421342813362654));
#81288=CARTESIAN_POINT('Ctrl Pts',(0.229995291247247,0.0587920952940921,
-0.422150687754273));
#81289=CARTESIAN_POINT('Ctrl Pts',(0.232294009029654,0.0489273353770943,
-0.422780358952519));
#81290=CARTESIAN_POINT('Ctrl Pts',(0.237037196548168,0.0204333440642143,
-0.424559824887115));
#81291=CARTESIAN_POINT('Ctrl Pts',(0.237910626745225,0.00162320656105648,
-0.425693173782317));
#81292=CARTESIAN_POINT('Ctrl Pts',(0.236281458244531,-0.0209238098545081,
-0.427145191866027));
#81293=CARTESIAN_POINT('Ctrl Pts',(0.235911642837729,-0.0247472712159931,
-0.427394415795856));
#81294=CARTESIAN_POINT('Ctrl Pts',(0.235224669817445,-0.0304107089922827,
-0.427768876627486));
#81295=CARTESIAN_POINT('Ctrl Pts',(0.234978357855017,-0.0322587588364578,
-0.427891908846852));
#81296=CARTESIAN_POINT('Ctrl Pts',(0.234497786365661,-0.0355661763147119,
-0.428113697962805));
#81297=CARTESIAN_POINT('Ctrl Pts',(0.234271621834312,-0.0370266355786783,
-0.428212195500903));
#81298=CARTESIAN_POINT('Ctrl Pts',(0.233760220369477,-0.0401365397177466,
-0.428423181146927));
#81299=CARTESIAN_POINT('Ctrl Pts',(0.233471141859209,-0.0417852619702745,
-0.4285357857508));
#81300=CARTESIAN_POINT('Ctrl Pts',(0.232635654857207,-0.0462707020427143,
-0.428844248329243));
#81301=CARTESIAN_POINT('Ctrl Pts',(0.232054846738631,-0.0491006375164009,
-0.429041181667275));
#81302=CARTESIAN_POINT('Ctrl Pts',(0.230647547267472,-0.0553734821709733,
-0.429483068607392));
#81303=CARTESIAN_POINT('Ctrl Pts',(0.229795369112122,-0.0588098602010125,
-0.429728780561197));
#81304=CARTESIAN_POINT('Ctrl Pts',(0.22681593787761,-0.0697682278568901,
-0.4305241902922));
#81305=CARTESIAN_POINT('Ctrl Pts',(0.224393821554575,-0.0772040686177263,
-0.431082234557229));
#81306=CARTESIAN_POINT('Ctrl Pts',(0.218471271451999,-0.0927353802134014,
-0.432283580479144));
#81307=CARTESIAN_POINT('Ctrl Pts',(0.214877388010344,-0.100783164098656,
-0.432927873152766));
#81308=CARTESIAN_POINT('Ctrl Pts',(0.205720516194495,-0.11855903740418,
-0.434385998512226));
#81309=CARTESIAN_POINT('Ctrl Pts',(0.19989851080186,-0.128132030393042,
-0.435196995646673));
#81310=CARTESIAN_POINT('Ctrl Pts',(0.192426520690626,-0.138661356039739,
-0.436093329800331));
#81311=CARTESIAN_POINT('Ctrl Pts',(0.191416109038451,-0.140052886982261,
-0.436211864544351));
#81312=CARTESIAN_POINT('Ctrl Pts',(0.189814427230167,-0.142208992147377,
-0.436395496025108));
#81313=CARTESIAN_POINT('Ctrl Pts',(0.189233490750703,-0.142981118661772,
-0.436461250042873));
#81314=CARTESIAN_POINT('Ctrl Pts',(0.188192408239198,-0.144347368324564,
-0.436577555989376));
#81315=CARTESIAN_POINT('Ctrl Pts',(0.187734150674308,-0.144942864449243,
-0.436628231553306));
#81316=CARTESIAN_POINT('Ctrl Pts',(0.186615425696446,-0.146382417226087,
-0.436750705099931));
#81317=CARTESIAN_POINT('Ctrl Pts',(0.185952057020649,-0.147224188845206,
-0.43682229930223));
#81318=CARTESIAN_POINT('Ctrl Pts',(0.183848013998961,-0.14985717242962,
-0.437046274789012));
#81319=CARTESIAN_POINT('Ctrl Pts',(0.182386943663814,-0.151632015481593,
-0.437197304596227));
#81320=CARTESIAN_POINT('Ctrl Pts',(0.174352344697524,-0.161107889310539,
-0.438005693813822));
#81321=CARTESIAN_POINT('Ctrl Pts',(0.16731589362262,-0.168404068336461,
-0.438635794415341));
#81322=CARTESIAN_POINT('Ctrl Pts',(0.145951821760804,-0.187891172976979,
-0.440417107446991));
#81323=CARTESIAN_POINT('Ctrl Pts',(0.130615686373842,-0.198858030215526,
-0.441551878486942));
#81324=CARTESIAN_POINT('Ctrl Pts',(0.110797626131273,-0.209739036233017,
-0.443004327343519));
#81325=CARTESIAN_POINT('Ctrl Pts',(0.107404866139155,-0.211496499678295,
-0.44325226101781));
#81326=CARTESIAN_POINT('Ctrl Pts',(0.102299024186799,-0.213986803282064,
-0.443625159537624));
#81327=CARTESIAN_POINT('Ctrl Pts',(0.100617262931436,-0.214782700421526,
-0.443747947240952));
#81328=CARTESIAN_POINT('Ctrl Pts',(0.0975834953430446,-0.216174987266577,
-0.443969470349743));
#81329=CARTESIAN_POINT('Ctrl Pts',(0.0962349369635496,-0.216778689962615,
-0.444067948984091));
#81330=CARTESIAN_POINT('Ctrl Pts',(0.0933445112548619,-0.218040346946825,
-0.444279084663897));
#81331=CARTESIAN_POINT('Ctrl Pts',(0.0918011396541931,-0.218694629989974,
-0.444391860021977));
#81332=CARTESIAN_POINT('Ctrl Pts',(0.0875687722106209,-0.220436165808188,
-0.444701291613612));
#81333=CARTESIAN_POINT('Ctrl Pts',(0.0848666375347113,-0.22149050905599,
-0.444899034646894));
#81334=CARTESIAN_POINT('Ctrl Pts',(0.0672399178255367,-0.227998357025257,
-0.446190713948813));
#81335=CARTESIAN_POINT('Ctrl Pts',(0.0518212622284608,-0.23198888563968,
-0.447332708186704));
#81336=CARTESIAN_POINT('Ctrl Pts',(0.0215639511476443,-0.236651556718902,
-0.449565000241521));
#81337=CARTESIAN_POINT('Ctrl Pts',(0.00682702320658603,-0.23753404809969,
-0.450647289008711));
#81338=CARTESIAN_POINT('Ctrl Pts',(-0.0100821772995698,-0.236970691288998,
-0.451828654756668));
#81339=CARTESIAN_POINT('Ctrl Pts',(-0.0122658630892032,-0.236867702057497,
-0.45198001066124));
#81340=CARTESIAN_POINT('Ctrl Pts',(-0.0154964764630396,-0.236670537742254,
-0.45220184493084));
#81341=CARTESIAN_POINT('Ctrl Pts',(-0.0165446342782324,-0.236599576077304,
-0.452273492266951));
#81342=CARTESIAN_POINT('Ctrl Pts',(-0.0184198200825886,-0.236460101102001,
-0.452401047239234));
#81343=CARTESIAN_POINT('Ctrl Pts',(-0.0192469952684292,-0.236394209784147,
-0.452457093061742));
#81344=CARTESIAN_POINT('Ctrl Pts',(-0.0210890951357676,-0.236237737991364,
-0.45258141481195));
#81345=CARTESIAN_POINT('Ctrl Pts',(-0.0221037976542683,-0.236144957621462,
-0.452649569190236));
#81346=CARTESIAN_POINT('Ctrl Pts',(-0.0251320036130714,-0.235848380463946,
-0.452852071771195));
#81347=CARTESIAN_POINT('Ctrl Pts',(-0.0271435884547158,-0.235625343390627,
-0.452985411116749));
#81348=CARTESIAN_POINT('Ctrl Pts',(-0.0410187650969288,-0.233906857716986,
-0.453898509300437));
#81349=CARTESIAN_POINT('Ctrl Pts',(-0.0527588509959145,-0.231541647410529,
-0.454638053952543));
#81350=CARTESIAN_POINT('Ctrl Pts',(-0.081833207260524,-0.223356568271885,
-0.456493799154509));
#81351=CARTESIAN_POINT('Ctrl Pts',(-0.0987636935471548,-0.216403528414672,
-0.45760176503617));
#81352=CARTESIAN_POINT('Ctrl Pts',(-0.117321196317661,-0.206146759942251,
-0.458970328473414));
#81353=CARTESIAN_POINT('Ctrl Pts',(-0.119885792636932,-0.204665935659423,
-0.459163005165487));
#81354=CARTESIAN_POINT('Ctrl Pts',(-0.124015415670018,-0.202177196611678,
-0.459479504181893));
#81355=CARTESIAN_POINT('Ctrl Pts',(-0.125597532954304,-0.201198164855224,
-0.459602288867322));
#81356=CARTESIAN_POINT('Ctrl Pts',(-0.128415108292639,-0.199408434206802,
-0.45982380869762));
#81357=CARTESIAN_POINT('Ctrl Pts',(-0.129654830168006,-0.198604603461101,
-0.459922287103312));
#81358=CARTESIAN_POINT('Ctrl Pts',(-0.132284910727145,-0.196864149033034,
-0.460133424656518));
#81359=CARTESIAN_POINT('Ctrl Pts',(-0.133673005024473,-0.195924266640102,
-0.460246202139215));
#81360=CARTESIAN_POINT('Ctrl Pts',(-0.137435399363368,-0.193318144268977,
-0.460555645790244));
#81361=CARTESIAN_POINT('Ctrl Pts',(-0.139789214189776,-0.191622984538444,
-0.460753398900938));
#81362=CARTESIAN_POINT('Ctrl Pts',(-0.154329659723102,-0.180740821885757,
-0.462001905387607));
#81363=CARTESIAN_POINT('Ctrl Pts',(-0.165634784178891,-0.170440176212749,
-0.463096667166265));
#81364=CARTESIAN_POINT('Ctrl Pts',(-0.186216135830429,-0.147693253771091,
-0.465331831430279));
#81365=CARTESIAN_POINT('Ctrl Pts',(-0.195422617626257,-0.135276818324557,
-0.46646686491421));
#81366=CARTESIAN_POINT('Ctrl Pts',(-0.204463497857814,-0.12021341569495,
-0.467693015300844));
#81367=CARTESIAN_POINT('Ctrl Pts',(-0.205543037438675,-0.11835813378653,
-0.467841574297239));
#81368=CARTESIAN_POINT('Ctrl Pts',(-0.207109519474475,-0.115579908537943,
-0.468060128327291));
#81369=CARTESIAN_POINT('Ctrl Pts',(-0.207615765331557,-0.114668053108156,
-0.468131244810757));
#81370=CARTESIAN_POINT('Ctrl Pts',(-0.208513893208211,-0.113024887714944,
-0.468258254284673));
#81371=CARTESIAN_POINT('Ctrl Pts',(-0.208907968994988,-0.112294832705891,
-0.468314279953584));
#81372=CARTESIAN_POINT('Ctrl Pts',(-0.209780797345346,-0.110657354895528,
-0.468439043474671));
#81373=CARTESIAN_POINT('Ctrl Pts',(-0.210257500768808,-0.109748879700463,
-0.468507654649401));
#81374=CARTESIAN_POINT('Ctrl Pts',(-0.211673219549259,-0.107007797666467,
-0.468712936030852));
#81375=CARTESIAN_POINT('Ctrl Pts',(-0.212594307452354,-0.105165972525613,
-0.468848555841296));
#81376=CARTESIAN_POINT('Ctrl Pts',(-0.214690953255747,-0.100833326201437,
-0.469162751974511));
#81377=CARTESIAN_POINT('Ctrl Pts',(-0.215847364245524,-0.0983335232871611,
-0.469340360800791));
#81378=CARTESIAN_POINT('Ctrl Pts',(-0.219856024708428,-0.0892563660339403,
-0.469974153753983));
#81379=CARTESIAN_POINT('Ctrl Pts',(-0.222453436923456,-0.0825702926907982,
-0.470420292817272));
#81380=CARTESIAN_POINT('Ctrl Pts',(-0.230389034410373,-0.0590342197491395,
-0.471952509570555));
#81381=CARTESIAN_POINT('Ctrl Pts',(-0.234145224059022,-0.0417148708401526,
-0.473018460337774));
#81382=CARTESIAN_POINT('Ctrl Pts',(-0.236440546165004,-0.019279789755122,
-0.47445454883603));
#81383=CARTESIAN_POINT('Ctrl Pts',(-0.236787440327543,-0.0144064228236565,
-0.474769392670411));
#81384=CARTESIAN_POINT('Ctrl Pts',(-0.237061123541786,-0.00759790565451577,
-0.475215058726645));
#81385=CARTESIAN_POINT('Ctrl Pts',(-0.237115093450983,-0.00566891181169765,
-0.475341968622919));
#81386=CARTESIAN_POINT('Ctrl Pts',(-0.237165227962936,-0.00248958002820659,
-0.47555229713523));
#81387=CARTESIAN_POINT('Ctrl Pts',(-0.237175055208515,-0.00123952823062238,
-0.475635288893505));
#81388=CARTESIAN_POINT('Ctrl Pts',(-0.237174999766729,1.05191258440349E-5,
-0.475718588717799));
#81389=CARTESIAN_POINT('Ctrl Pts',(-0.23717499976624,1.0530156552288E-5,
-0.475718589452856));
#81390=CARTESIAN_POINT('Ctrl Pts',(-0.237174948687184,0.00116100449970449,
-0.475795253998586));
#81391=CARTESIAN_POINT('Ctrl Pts',(-0.237166526634602,0.00231144960027964,
-0.475872177768488));
#81392=CARTESIAN_POINT('Ctrl Pts',(-0.237123304695454,0.00527237912689858,
-0.476070854539049));
#81393=CARTESIAN_POINT('Ctrl Pts',(-0.237076140530004,0.00708257631464626,
-0.476192988308165));
#81394=CARTESIAN_POINT('Ctrl Pts',(-0.236878960709074,0.0123382190362649,
-0.476549618360509));
#81395=CARTESIAN_POINT('Ctrl Pts',(-0.236674524732556,0.0157810282805962,
-0.47678578196556));
#81396=CARTESIAN_POINT('Ctrl Pts',(-0.235117606002505,0.0349322337340345,
-0.478114321511021));
#81397=CARTESIAN_POINT('Ctrl Pts',(-0.23227662357456,0.0504773375061679,
-0.479252328537395));
#81398=CARTESIAN_POINT('Ctrl Pts',(-0.224035792179592,0.0790985965470245,
-0.481425694060155));
#81399=CARTESIAN_POINT('Ctrl Pts',(-0.218968026705839,0.0922046536630583,
-0.482453287762943));
#81400=CARTESIAN_POINT('Ctrl Pts',(-0.211867864855361,0.106621623481787,
-0.483573513488986));
#81401=CARTESIAN_POINT('Ctrl Pts',(-0.210940617270537,0.108444545454168,
-0.483714924562397));
#81402=CARTESIAN_POINT('Ctrl Pts',(-0.209514248503541,0.111161176174543,
-0.48392506466096));
#81403=CARTESIAN_POINT('Ctrl Pts',(-0.209032760534276,0.112063966267974,
-0.483994797618628));
#81404=CARTESIAN_POINT('Ctrl Pts',(-0.208150265699311,0.113693165538168,
-0.484120418281874));
#81405=CARTESIAN_POINT('Ctrl Pts',(-0.207751277711071,0.114420608546443,
-0.484176424188112));
#81406=CARTESIAN_POINT('Ctrl Pts',(-0.206840686760009,0.11606034995594,
-0.484302484120207));
#81407=CARTESIAN_POINT('Ctrl Pts',(-0.206326858655653,0.116971372701702,
-0.484372397012738));
#81408=CARTESIAN_POINT('Ctrl Pts',(-0.204732579325275,0.119754853165022,
-0.48458571473549));
#81409=CARTESIAN_POINT('Ctrl Pts',(-0.203632506803046,0.121616022270201,
-0.48472794438393));
#81410=CARTESIAN_POINT('Ctrl Pts',(-0.194592140694416,0.136444380172736,
-0.485860013904881));
#81411=CARTESIAN_POINT('Ctrl Pts',(-0.185445969751487,0.14863744590539,
-0.486785537049803));
#81412=CARTESIAN_POINT('Ctrl Pts',(-0.164651975309836,0.171424323933707,
-0.488677612033645));
#81413=CARTESIAN_POINT('Ctrl Pts',(-0.152994632713465,0.181904176188249,
-0.489641117585276));
#81414=CARTESIAN_POINT('Ctrl Pts',(-0.13813676467458,0.192816082915931,
-0.490836695426189));
#81415=CARTESIAN_POINT('Ctrl Pts',(-0.135852834256483,0.194432029091879,
-0.491019553968737));
#81416=CARTESIAN_POINT('Ctrl Pts',(-0.132173578805488,0.196938729538459,
-0.491312992359567));
#81417=CARTESIAN_POINT('Ctrl Pts',(-0.130796546645268,0.197855960938178,
-0.491422570144538));
#81418=CARTESIAN_POINT('Ctrl Pts',(-0.128168842334359,0.199566836420298,
-0.491631268692151));
#81419=CARTESIAN_POINT('Ctrl Pts',(-0.126920107262241,0.200363321358311,
-0.491730277351478));
#81420=CARTESIAN_POINT('Ctrl Pts',(-0.124055679386195,0.202152826793797,
-0.49195705238228));
#81421=CARTESIAN_POINT('Ctrl Pts',(-0.122435389493696,0.203138258350459,
-0.492085088998462));
#81422=CARTESIAN_POINT('Ctrl Pts',(-0.117348365169996,0.206149125047098,
-0.492486426520427));
#81423=CARTESIAN_POINT('Ctrl Pts',(-0.11384205862814,0.208105941418819,
-0.492762149445229));
#81424=CARTESIAN_POINT('Ctrl Pts',(-0.0938456168706689,0.218609051507495,
-0.494330456337261));
#81425=CARTESIAN_POINT('Ctrl Pts',(-0.0764481626599829,0.225282854049497,
-0.495686712086374));
#81426=CARTESIAN_POINT('Ctrl Pts',(-0.0529915936470424,0.231248019875964,
-0.497451181145954));
#81427=CARTESIAN_POINT('Ctrl Pts',(-0.0474817943861408,0.232441842789692,
-0.497860620798539));
#81428=CARTESIAN_POINT('Ctrl Pts',(-0.0419358198037385,0.233438145217075,
-0.498265075600824));
#81429=CARTESIAN_POINT('Ctrl Pts',(-0.0419358519811633,0.233438139436584,
-0.517821408604162));
#81430=CARTESIAN_POINT('Ctrl Pts',(-0.0474363747086211,0.232450001390785,
-0.517413505363854));
#81431=CARTESIAN_POINT('Ctrl Pts',(-0.0529036475820301,0.231267149309306,
-0.5170050099961));
#81432=CARTESIAN_POINT('Ctrl Pts',(-0.0639541237075591,0.228463454109606,
-0.516177751915909));
#81433=CARTESIAN_POINT('Ctrl Pts',(-0.0695269999125132,0.226829637732628,
-0.515759708792094));
#81434=CARTESIAN_POINT('Ctrl Pts',(-0.0783878880691696,0.22387455112594,
-0.51509885600743));
#81435=CARTESIAN_POINT('Ctrl Pts',(-0.0817159586215557,0.222681344036066,
-0.514851553249294));
#81436=CARTESIAN_POINT('Ctrl Pts',(-0.0861979953421363,0.220960377579042,
-0.514520868445073));
#81437=CARTESIAN_POINT('Ctrl Pts',(-0.0873760566340872,0.220497183127309,
-0.514434176928649));
#81438=CARTESIAN_POINT('Ctrl Pts',(-0.0893466811362861,0.219704091872445,
-0.514289608902803));
#81439=CARTESIAN_POINT('Ctrl Pts',(-0.0901412532691321,0.219379287910176,
-0.514231441019731));
#81440=CARTESIAN_POINT('Ctrl Pts',(-0.0916655664153254,0.218746501361038,
-0.514120110990824));
#81441=CARTESIAN_POINT('Ctrl Pts',(-0.0923955502470242,0.218439168339515,
-0.51406690886264));
#81442=CARTESIAN_POINT('Ctrl Pts',(-0.0943806966640465,0.217591663149007,
-0.513922501548323));
#81443=CARTESIAN_POINT('Ctrl Pts',(-0.0956327760756426,0.217044281506648,
-0.513831718758105));
#81444=CARTESIAN_POINT('Ctrl Pts',(-0.100543664870647,0.214846600592293,
-0.513476561634498));
#81445=CARTESIAN_POINT('Ctrl Pts',(-0.104165289009907,0.213114258979825,
-0.513216643371228));
#81446=CARTESIAN_POINT('Ctrl Pts',(-0.120457596759089,0.204806479119431,
-0.512048756835134));
#81447=CARTESIAN_POINT('Ctrl Pts',(-0.132563602642342,0.19718695061971,
-0.511183473043809));
#81448=CARTESIAN_POINT('Ctrl Pts',(-0.155046227311638,0.180024635124865,
-0.509446079772267));
#81449=CARTESIAN_POINT('Ctrl Pts',(-0.16540444082263,0.170556444231113,
-0.508577361498009));
#81450=CARTESIAN_POINT('Ctrl Pts',(-0.176734137257871,0.158191879370237,
-0.507489332179975));
#81451=CARTESIAN_POINT('Ctrl Pts',(-0.178566269267511,0.156120826327559,
-0.507308559973476));
#81452=CARTESIAN_POINT('Ctrl Pts',(-0.181431441977682,0.152765591810468,
-0.507017703061679));
#81453=CARTESIAN_POINT('Ctrl Pts',(-0.18248806497027,0.151501815475246,
-0.506908589691881));
#81454=CARTESIAN_POINT('Ctrl Pts',(-0.184470158768019,0.149080306092478,
-0.506700285174179));
#81455=CARTESIAN_POINT('Ctrl Pts',(-0.185398112555181,0.147924699865153,
-0.506601200855444));
#81456=CARTESIAN_POINT('Ctrl Pts',(-0.187495795921603,0.145261652111095,
-0.506373554833203));
#81457=CARTESIAN_POINT('Ctrl Pts',(-0.188658274194058,0.143748656589063,
-0.506244714806875));
#81458=CARTESIAN_POINT('Ctrl Pts',(-0.192161078473539,0.13907398448482,
-0.505848042663517));
#81459=CARTESIAN_POINT('Ctrl Pts',(-0.194441008678585,0.135868113211522,
-0.505577923443962));
#81460=CARTESIAN_POINT('Ctrl Pts',(-0.207043826142121,0.117179694422902,
-0.504013223461699));
#81461=CARTESIAN_POINT('Ctrl Pts',(-0.215594320143711,0.100583709091513,
-0.502654496642408));
#81462=CARTESIAN_POINT('Ctrl Pts',(-0.225646731605244,0.0737352194672967,
-0.50056445184781));
#81463=CARTESIAN_POINT('Ctrl Pts',(-0.228573212470532,0.0640909969134751,
-0.499834974724211));
#81464=CARTESIAN_POINT('Ctrl Pts',(-0.231402801853073,0.0520574648619317,
-0.49897072711782));
#81465=CARTESIAN_POINT('Ctrl Pts',(-0.231895201443057,0.0498181981701591,
-0.498811834512575));
#81466=CARTESIAN_POINT('Ctrl Pts',(-0.232569772829281,0.0465234041106976,
-0.498581207215899));
#81467=CARTESIAN_POINT('Ctrl Pts',(-0.232777373582377,0.0454732979136019,
-0.498508171077071));
#81468=CARTESIAN_POINT('Ctrl Pts',(-0.233118535025439,0.0436840172180781,
-0.498384562006488));
#81469=CARTESIAN_POINT('Ctrl Pts',(-0.233255702961347,0.0429455681829708,
-0.498333791271857));
#81470=CARTESIAN_POINT('Ctrl Pts',(-0.233561377126923,0.0412552790365975,
-0.498218141215521));
#81471=CARTESIAN_POINT('Ctrl Pts',(-0.233727575216785,0.04030304702857,
-0.498153391556591));
#81472=CARTESIAN_POINT('Ctrl Pts',(-0.234173638929645,0.0376517269303887,
-0.497974158228261));
#81473=CARTESIAN_POINT('Ctrl Pts',(-0.234440836215068,0.0359505277811405,
-0.497860351811799));
#81474=CARTESIAN_POINT('Ctrl Pts',(-0.236334195744034,0.0229754365276078,
-0.497000407236665));
#81475=CARTESIAN_POINT('Ctrl Pts',(-0.23716503959585,0.0115989474799725,
-0.496292275500453));
#81476=CARTESIAN_POINT('Ctrl Pts',(-0.237191861597142,-0.0193587470715879,
-0.494386761147839));
#81477=CARTESIAN_POINT('Ctrl Pts',(-0.234788242447255,-0.0388477650666085,
-0.493204015519732));
#81478=CARTESIAN_POINT('Ctrl Pts',(-0.229333442885873,-0.0605480423193224,
-0.491757564325757));
#81479=CARTESIAN_POINT('Ctrl Pts',(-0.228599223550157,-0.0632636338908996,
-0.491574315511196));
#81480=CARTESIAN_POINT('Ctrl Pts',(-0.227311658198912,-0.0677103437442107,
-0.491270199866006));
#81481=CARTESIAN_POINT('Ctrl Pts',(-0.22678639377019,-0.0694493477119902,
-0.491150236588488));
#81482=CARTESIAN_POINT('Ctrl Pts',(-0.225798883753325,-0.0725879941771109,
-0.490931763194872));
#81483=CARTESIAN_POINT('Ctrl Pts',(-0.225343464352043,-0.0739897000198598,
-0.490833480176166));
#81484=CARTESIAN_POINT('Ctrl Pts',(-0.224332568282615,-0.0770051422215605,
-0.490620458013356));
#81485=CARTESIAN_POINT('Ctrl Pts',(-0.223772681184231,-0.0786173009756907,
-0.490505578316715));
#81486=CARTESIAN_POINT('Ctrl Pts',(-0.222165130873761,-0.0830897944873623,
-0.490184035258809));
#81487=CARTESIAN_POINT('Ctrl Pts',(-0.221079720355334,-0.0859361104186254,
-0.489976137257953));
#81488=CARTESIAN_POINT('Ctrl Pts',(-0.218521157628301,-0.0922759698600765,
-0.489505476684963));
#81489=CARTESIAN_POINT('Ctrl Pts',(-0.21701847390357,-0.095756619461184,
-0.489241795583941));
#81490=CARTESIAN_POINT('Ctrl Pts',(-0.211786229519685,-0.10711955407712,
-0.48836328070516));
#81491=CARTESIAN_POINT('Ctrl Pts',(-0.207705743164228,-0.114831633191772,
-0.487738029556811));
#81492=CARTESIAN_POINT('Ctrl Pts',(-0.196664308342083,-0.133177639686777,
-0.486184792103082));
#81493=CARTESIAN_POINT('Ctrl Pts',(-0.189255644617005,-0.143511100302924,
-0.485250529200367));
#81494=CARTESIAN_POINT('Ctrl Pts',(-0.177075470136653,-0.157905747709544,
-0.483893797334847));
#81495=CARTESIAN_POINT('Ctrl Pts',(-0.172913167082312,-0.162453064112888,
-0.483456129411124));
#81496=CARTESIAN_POINT('Ctrl Pts',(-0.16746906007165,-0.167954101850235,
-0.482920138893986));
#81497=CARTESIAN_POINT('Ctrl Pts',(-0.166348838695005,-0.169063688027147,
-0.482811677001675));
#81498=CARTESIAN_POINT('Ctrl Pts',(-0.164553929112457,-0.170806442289736,
-0.482640882851405));
#81499=CARTESIAN_POINT('Ctrl Pts',(-0.163886481172157,-0.171446952952293,
-0.48257801483154));
#81500=CARTESIAN_POINT('Ctrl Pts',(-0.162600626980336,-0.172666541088275,
-0.48245815277016));
#81501=CARTESIAN_POINT('Ctrl Pts',(-0.161982846085595,-0.173246229111305,
-0.482401115458312));
#81502=CARTESIAN_POINT('Ctrl Pts',(-0.160479178310591,-0.174642105022481,
-0.482263579109867));
#81503=CARTESIAN_POINT('Ctrl Pts',(-0.159590139608728,-0.175454891671309,
-0.482183332203441));
#81504=CARTESIAN_POINT('Ctrl Pts',(-0.156391825620771,-0.178334465188169,
-0.481898276826869));
#81505=CARTESIAN_POINT('Ctrl Pts',(-0.154048173734127,-0.180362820378453,
-0.481696077325965));
#81506=CARTESIAN_POINT('Ctrl Pts',(-0.147975952278621,-0.18541339204013,
-0.481186910370073));
#81507=CARTESIAN_POINT('Ctrl Pts',(-0.144194083644675,-0.18836953127005,
-0.480883400976566));
#81508=CARTESIAN_POINT('Ctrl Pts',(-0.126034239725389,-0.201696715798944,
-0.479474880747289));
#81509=CARTESIAN_POINT('Ctrl Pts',(-0.110612835566416,-0.210549375116307,
-0.478413363290233));
#81510=CARTESIAN_POINT('Ctrl Pts',(-0.0873439737509716,-0.22063838791123,
-0.476824649177911));
#81511=CARTESIAN_POINT('Ctrl Pts',(-0.08019749745354,-0.22333520018733,
-0.476338998764583));
#81512=CARTESIAN_POINT('Ctrl Pts',(-0.0705963671478269,-0.22643800129007,
-0.475682121669746));
#81513=CARTESIAN_POINT('Ctrl Pts',(-0.0682472868567034,-0.227157043876955,
-0.475521084603522));
#81514=CARTESIAN_POINT('Ctrl Pts',(-0.0643680360670255,-0.228278861281466,
-0.475254412055304));
#81515=CARTESIAN_POINT('Ctrl Pts',(-0.0628442151540498,-0.228703054181387,
-0.47514947499829));
#81516=CARTESIAN_POINT('Ctrl Pts',(-0.059862728825461,-0.229500977144621,
-0.47494374245077));
#81517=CARTESIAN_POINT('Ctrl Pts',(-0.0584055222583933,-0.229876139698764,
-0.474842998757251));
#81518=CARTESIAN_POINT('Ctrl Pts',(-0.0549422779374243,-0.230732707765821,
-0.474603067246757));
#81519=CARTESIAN_POINT('Ctrl Pts',(-0.052933362995506,-0.231201848939181,
-0.474463494162119));
#81520=CARTESIAN_POINT('Ctrl Pts',(-0.0460224206253254,-0.232720967451871,
-0.473981852283147));
#81521=CARTESIAN_POINT('Ctrl Pts',(-0.0410936578333632,-0.23364164149369,
-0.473635758173797));
#81522=CARTESIAN_POINT('Ctrl Pts',(-0.0287998332566006,-0.235537056444383,
-0.472765583326596));
#81523=CARTESIAN_POINT('Ctrl Pts',(-0.0214114705284497,-0.236323225247371,
-0.472236432372466));
#81524=CARTESIAN_POINT('Ctrl Pts',(-0.00500772401503966,-0.23729312773985,
-0.471051021716483));
#81525=CARTESIAN_POINT('Ctrl Pts',(0.0040062119849757,-0.237312124539667,
-0.470392508379135));
#81526=CARTESIAN_POINT('Ctrl Pts',(0.0245962114854714,-0.23618193827456,
-0.468888181766194));
#81527=CARTESIAN_POINT('Ctrl Pts',(0.0361323536563384,-0.234694256886078,
-0.468045052995556));
#81528=CARTESIAN_POINT('Ctrl Pts',(0.0492054890819199,-0.232021078533424,
-0.467118600397889));
#81529=CARTESIAN_POINT('Ctrl Pts',(0.0508931145627777,-0.231656755485669,
-0.466999585794828));
#81530=CARTESIAN_POINT('Ctrl Pts',(0.0535201861045875,-0.231059530277086,
-0.466815385709719));
#81531=CARTESIAN_POINT('Ctrl Pts',(0.054462400505281,-0.230839259804835,
-0.466749536432177));
#81532=CARTESIAN_POINT('Ctrl Pts',(0.0561334095516349,-0.230437811227578,
-0.466633167763421));
#81533=CARTESIAN_POINT('Ctrl Pts',(0.0568627035468804,-0.230258935722715,
-0.466582523562648));
#81534=CARTESIAN_POINT('Ctrl Pts',(0.0586281207009968,-0.229817028811714,
-0.466460263420599));
#81535=CARTESIAN_POINT('Ctrl Pts',(0.0596633316924259,-0.229550452471458,
-0.466388849487474));
#81536=CARTESIAN_POINT('Ctrl Pts',(0.0629053871605886,-0.228692179432054,
-0.466165965575008));
#81537=CARTESIAN_POINT('Ctrl Pts',(0.0651055805920964,-0.228075568583827,
-0.466015828782985));
#81538=CARTESIAN_POINT('Ctrl Pts',(0.0768764022367824,-0.224592535889649,
-0.465216946794672));
#81539=CARTESIAN_POINT('Ctrl Pts',(0.0862686413014294,-0.221155047170527,
-0.464594762711305));
#81540=CARTESIAN_POINT('Ctrl Pts',(0.112231371224865,-0.209746084648454,
-0.462847169024363));
#81541=CARTESIAN_POINT('Ctrl Pts',(0.128129273282322,-0.200429900160325,
-0.461738256465763));
#81542=CARTESIAN_POINT('Ctrl Pts',(0.146147297677237,-0.186843778130154,
-0.460292991855457));
#81543=CARTESIAN_POINT('Ctrl Pts',(0.149433723081102,-0.184225918383934,
-0.46002098582327));
#81544=CARTESIAN_POINT('Ctrl Pts',(0.154109529990292,-0.180293861019471,
-0.459620413415811));
#81545=CARTESIAN_POINT('Ctrl Pts',(0.155555397168203,-0.179047875200486,
-0.459494581118363));
#81546=CARTESIAN_POINT('Ctrl Pts',(0.158100075016996,-0.176800892755009,
-0.45926948927998));
#81547=CARTESIAN_POINT('Ctrl Pts',(0.159204822273176,-0.175806751272082,
-0.459170516950115));
#81548=CARTESIAN_POINT('Ctrl Pts',(0.161501654315041,-0.173700472032592,
-0.458962057394118));
#81549=CARTESIAN_POINT('Ctrl Pts',(0.162691757211531,-0.172586297940097,
-0.458852486818846));
#81550=CARTESIAN_POINT('Ctrl Pts',(0.16581135277148,-0.169604791959639,
-0.458561048180622));
#81551=CARTESIAN_POINT('Ctrl Pts',(0.167720735058996,-0.167716857133169,
-0.458378296916408));
#81552=CARTESIAN_POINT('Ctrl Pts',(0.177853310873583,-0.157352009520242,
-0.457384106102446));
#81553=CARTESIAN_POINT('Ctrl Pts',(0.18546547780925,-0.148303524315382,
-0.456547097401718));
#81554=CARTESIAN_POINT('Ctrl Pts',(0.201168075150133,-0.126528911262841,
-0.45460647208975));
#81555=CARTESIAN_POINT('Ctrl Pts',(0.208784357212976,-0.113521997333308,
-0.453495982675036));
#81556=CARTESIAN_POINT('Ctrl Pts',(0.217358324734248,-0.0950560159413913,
-0.452037395009256));
#81557=CARTESIAN_POINT('Ctrl Pts',(0.219436103982255,-0.0901559394699398,
-0.451661069967338));
#81558=CARTESIAN_POINT('Ctrl Pts',(0.221888315157406,-0.0837843883339581,
-0.451188799170902));
#81559=CARTESIAN_POINT('Ctrl Pts',(0.222415806514101,-0.0823738880858151,
-0.451085303282932));
#81560=CARTESIAN_POINT('Ctrl Pts',(0.223240318901954,-0.0801034827217346,
-0.450920501158236));
#81561=CARTESIAN_POINT('Ctrl Pts',(0.223545879012346,-0.0792467537152166,
-0.450858719302756));
#81562=CARTESIAN_POINT('Ctrl Pts',(0.224128986056774,-0.0775816260578697,
-0.450739454934526));
#81563=CARTESIAN_POINT('Ctrl Pts',(0.224407102023338,-0.0767734568742039,
-0.450681942686566));
#81564=CARTESIAN_POINT('Ctrl Pts',(0.22508004407438,-0.0747830718956505,
-0.450541176337997));
#81565=CARTESIAN_POINT('Ctrl Pts',(0.22546993872044,-0.0735991914731807,
-0.450458204608852));
#81566=CARTESIAN_POINT('Ctrl Pts',(0.226885885281138,-0.0691829195967079,
-0.450151305012192));
#81567=CARTESIAN_POINT('Ctrl Pts',(0.227851960497856,-0.0659315420715444,
-0.449930541175777));
#81568=CARTESIAN_POINT('Ctrl Pts',(0.230191148893845,-0.0573920975881784,
-0.44936145706513));
#81569=CARTESIAN_POINT('Ctrl Pts',(0.231451938620924,-0.0520751931532557,
-0.449017710949226));
#81570=CARTESIAN_POINT('Ctrl Pts',(0.234506021520461,-0.036874581640039,
-0.44805283837193));
#81571=CARTESIAN_POINT('Ctrl Pts',(0.235856854352183,-0.0269140399993006,
-0.447441360666662));
#81572=CARTESIAN_POINT('Ctrl Pts',(0.237540433790436,-0.00334335838640604,
-0.445989117417048));
#81573=CARTESIAN_POINT('Ctrl Pts',(0.237341843897199,0.0102672828883438,
-0.445145320104005));
#81574=CARTESIAN_POINT('Ctrl Pts',(0.235698533997672,0.0265710807385324,
-0.444082592714595));
#81575=CARTESIAN_POINT('Ctrl Pts',(0.23536841938081,0.0293517860144907,
-0.443899578232512));
#81576=CARTESIAN_POINT('Ctrl Pts',(0.234765023559825,0.0337654045215603,
-0.44360596868346));
#81577=CARTESIAN_POINT('Ctrl Pts',(0.234523736615272,0.0354024795756392,
-0.44349637820177));
#81578=CARTESIAN_POINT('Ctrl Pts',(0.234034144551942,0.0384992444855046,
-0.443287706248749));
#81579=CARTESIAN_POINT('Ctrl Pts',(0.233789261356166,0.0399594012206306,
-0.443188737350116));
#81580=CARTESIAN_POINT('Ctrl Pts',(0.233199881109878,0.043282624234656,
-0.442962125832387));
#81581=CARTESIAN_POINT('Ctrl Pts',(0.232846701875595,0.0451440270073093,
-0.442834213972802));
#81582=CARTESIAN_POINT('Ctrl Pts',(0.23167723951048,0.0509283012195884,
-0.442433562950964));
#81583=CARTESIAN_POINT('Ctrl Pts',(0.230783860115667,0.0548346761049098,
-0.44215841301894));
#81584=CARTESIAN_POINT('Ctrl Pts',(0.226210987774366,0.0727310457667311,
-0.440875957642474));
#81585=CARTESIAN_POINT('Ctrl Pts',(0.221355918781468,0.0863866515042328,
-0.439832420772612));
#81586=CARTESIAN_POINT('Ctrl Pts',(0.209308573419601,0.112450118617004,
-0.437737996345271));
#81587=CARTESIAN_POINT('Ctrl Pts',(0.202174241546572,0.124822876991005,
-0.436692094656722));
#81588=CARTESIAN_POINT('Ctrl Pts',(0.192684002517075,0.138310743835322,
-0.43553981688051));
#81589=CARTESIAN_POINT('Ctrl Pts',(0.191370603419139,0.140122374148513,
-0.435384821033287));
#81590=CARTESIAN_POINT('Ctrl Pts',(0.189397388534701,0.142764609239526,
-0.435158740443828));
#81591=CARTESIAN_POINT('Ctrl Pts',(0.188757368299707,0.143609750559554,
-0.435086423464367));
#81592=CARTESIAN_POINT('Ctrl Pts',(0.18760623413405,0.1451088222302,-0.434958187119187));
#81593=CARTESIAN_POINT('Ctrl Pts',(0.187097331179468,0.145764392447521,
-0.43490212250994));
#81594=CARTESIAN_POINT('Ctrl Pts',(0.18596151183434,0.147211808867722,-0.434778373972197));
#81595=CARTESIAN_POINT('Ctrl Pts',(0.185332969538141,0.148002334608258,
-0.434710805129797));
#81596=CARTESIAN_POINT('Ctrl Pts',(0.183457409672624,0.150330565343857,
-0.4345117755574));
#81597=CARTESIAN_POINT('Ctrl Pts',(0.18219613187673,0.151856742353953,-0.434381273204359));
#81598=CARTESIAN_POINT('Ctrl Pts',(0.179224250213282,0.155362453789661,
-0.434080933991697));
#81599=CARTESIAN_POINT('Ctrl Pts',(0.177499686395286,0.157329865053322,
-0.433911950848822));
#81600=CARTESIAN_POINT('Ctrl Pts',(0.171310352369061,0.164159412161296,
-0.433322135447074));
#81601=CARTESIAN_POINT('Ctrl Pts',(0.16667529190237,0.168863579460885,-0.432909927488604));
#81602=CARTESIAN_POINT('Ctrl Pts',(0.146598175691034,0.187606747740174,
-0.431211477253744));
#81603=CARTESIAN_POINT('Ctrl Pts',(0.129535996403746,0.199769128416463,
-0.429959671403605));
#81604=CARTESIAN_POINT('Ctrl Pts',(0.108392180397272,0.21097992788225,-0.428416658049038));
#81605=CARTESIAN_POINT('Ctrl Pts',(0.105653876589978,0.212364431400599,
-0.428217188673281));
#81606=CARTESIAN_POINT('Ctrl Pts',(0.101185545933529,0.214515833468829,
-0.427891820819048));
#81607=CARTESIAN_POINT('Ctrl Pts',(0.0994717988380659,0.215315857303474,
-0.427767062057602));
#81608=CARTESIAN_POINT('Ctrl Pts',(0.0964000803457126,0.216705320834227,
-0.427543402880788));
#81609=CARTESIAN_POINT('Ctrl Pts',(0.0950457985746646,0.21730270953729,
-0.427444780326438));
#81610=CARTESIAN_POINT('Ctrl Pts',(0.0921641005951461,0.218541766529488,
-0.427234852314439));
#81611=CARTESIAN_POINT('Ctrl Pts',(0.0906353814136036,0.219180182843437,
-0.427123442951149));
#81612=CARTESIAN_POINT('Ctrl Pts',(0.0864967862554318,0.220857822300506,
-0.426821648550179));
#81613=CARTESIAN_POINT('Ctrl Pts',(0.0838749988925018,0.221866750749245,
-0.426630265010702));
#81614=CARTESIAN_POINT('Ctrl Pts',(0.0780271231807158,0.223998692301575,
-0.426202777279461));
#81615=CARTESIAN_POINT('Ctrl Pts',(0.0747934942543724,0.22509903882262,
-0.425965988385402));
#81616=CARTESIAN_POINT('Ctrl Pts',(0.0644913744791733,0.228358179068569,
-0.425210191062396));
#81617=CARTESIAN_POINT('Ctrl Pts',(0.0573456574394171,0.230256495304766,
-0.424683738611355));
#81618=CARTESIAN_POINT('Ctrl Pts',(0.0412858622062586,0.23372893323647,
-0.423498652320382));
#81619=CARTESIAN_POINT('Ctrl Pts',(0.032346435169881,0.235132798464378,
-0.422837608714053));
#81620=CARTESIAN_POINT('Ctrl Pts',(0.0117668686477449,0.237168679492262,
-0.421328945360437));
#81621=CARTESIAN_POINT('Ctrl Pts',(0.000114663382083139,0.237460498622356,
-0.420483994371155));
#81622=CARTESIAN_POINT('Ctrl Pts',(-0.013237917530875,0.236811572088418,
-0.419555818733266));
#81623=CARTESIAN_POINT('Ctrl Pts',(-0.0149619725548211,0.236708899168758,
-0.419436761457891));
#81624=CARTESIAN_POINT('Ctrl Pts',(-0.0176501399456274,0.236519321989584,
-0.419252509798154));
#81625=CARTESIAN_POINT('Ctrl Pts',(-0.018615062249009,0.236445335448843,
-0.419186651046793));
#81626=CARTESIAN_POINT('Ctrl Pts',(-0.0203278645731972,0.236303454058981,
-0.419070274300169));
#81627=CARTESIAN_POINT('Ctrl Pts',(-0.0210758870510178,0.236237912890664,
-0.419019631392924));
#81628=CARTESIAN_POINT('Ctrl Pts',(-0.0228878334594393,0.236070476613085,
-0.418897385477494));
#81629=CARTESIAN_POINT('Ctrl Pts',(-0.023951396821383,0.235964941355194,
-0.418825984344563));
#81630=CARTESIAN_POINT('Ctrl Pts',(-0.0272851828667561,0.235611363545848,
-0.418603182578419));
#81631=CARTESIAN_POINT('Ctrl Pts',(-0.0295526355931031,0.235337711610666,
-0.418453113735775));
#81632=CARTESIAN_POINT('Ctrl Pts',(-0.0352008980436093,0.234573113764485,
-0.418082165477073));
#81633=CARTESIAN_POINT('Ctrl Pts',(-0.0385749975013287,0.234041897731114,
-0.417863152886784));
#81634=CARTESIAN_POINT('Ctrl Pts',(-0.0419358280420692,0.233438143737107,
-0.417646538149483));
#81635=CARTESIAN_POINT('Origin',(0.,0.,-1.7456589891905));
#81636=CARTESIAN_POINT('',(-0.0419358007114473,0.233438148646895,-0.298061760785893));
#81637=CARTESIAN_POINT('',(-0.0419358257618152,0.233438144146741,-0.318008956663326));
#81638=CARTESIAN_POINT('',(-0.0419358257166344,0.233438144154858,-1.7456589891905));
#81639=CARTESIAN_POINT('Ctrl Pts',(-0.0419358007114439,0.233438148646895,
-0.298061760785893));
#81640=CARTESIAN_POINT('Ctrl Pts',(-0.0297893085885032,0.23562019505175,
-0.298821763567408));
#81641=CARTESIAN_POINT('Ctrl Pts',(-0.0174860841807818,0.236851817310879,
-0.299591780052587));
#81642=CARTESIAN_POINT('Ctrl Pts',(-0.00231027385586464,0.237180603483249,
-0.300575944362926));
#81643=CARTESIAN_POINT('Ctrl Pts',(0.000517444212155474,0.237191288158712,
-0.30076071581006));
#81644=CARTESIAN_POINT('Ctrl Pts',(0.00500531661435507,0.237127995007377,
-0.301056502375512));
#81645=CARTESIAN_POINT('Ctrl Pts',(0.00666572203421282,0.237087129816031,
-0.301166486719452));
#81646=CARTESIAN_POINT('Ctrl Pts',(0.00980455108933783,0.23697687991778,
-0.30137550591229));
#81647=CARTESIAN_POINT('Ctrl Pts',(0.011283027490894,0.236911088718465,
-0.30147442381241));
#81648=CARTESIAN_POINT('Ctrl Pts',(0.0146434567019853,0.23673002476781,
-0.301700355023327));
#81649=CARTESIAN_POINT('Ctrl Pts',(0.0165248249644296,0.236606139511143,
-0.301827631146487));
#81650=CARTESIAN_POINT('Ctrl Pts',(0.0214423077496373,0.236223395172807,
-0.302162445564757));
#81651=CARTESIAN_POINT('Ctrl Pts',(0.0244751778925771,0.235928440765466,
-0.302371087982261));
#81652=CARTESIAN_POINT('Ctrl Pts',(0.0446116223629093,0.233577681224988,
-0.303771171124661));
#81653=CARTESIAN_POINT('Ctrl Pts',(0.0614503940892971,0.229722388557461,
-0.305018912125014));
#81654=CARTESIAN_POINT('Ctrl Pts',(0.0898160050584016,0.219884011388673,
-0.307210581904954));
#81655=CARTESIAN_POINT('Ctrl Pts',(0.101553576667183,0.214715691855634,
-0.308145159063142));
#81656=CARTESIAN_POINT('Ctrl Pts',(0.114605246062226,0.20765776921121,-0.309179293645274));
#81657=CARTESIAN_POINT('Ctrl Pts',(0.116380623189711,0.206668001329654,
-0.309319818881318));
#81658=CARTESIAN_POINT('Ctrl Pts',(0.119028126340582,0.205147087378855,
-0.309528913082343));
#81659=CARTESIAN_POINT('Ctrl Pts',(0.119909853005656,0.204632963056893,
-0.309598471812567));
#81660=CARTESIAN_POINT('Ctrl Pts',(0.121502335724596,0.203690577886412,
-0.309723921279298));
#81661=CARTESIAN_POINT('Ctrl Pts',(0.122214184277925,0.203264267190231,
-0.309779928378966));
#81662=CARTESIAN_POINT('Ctrl Pts',(0.123820596145058,0.202290731803867,
-0.309906167867792));
#81663=CARTESIAN_POINT('Ctrl Pts',(0.124713782161633,0.201741301786073,
-0.309976257179257));
#81664=CARTESIAN_POINT('Ctrl Pts',(0.127449042647001,0.200033638892799,
-0.310190677841086));
#81665=CARTESIAN_POINT('Ctrl Pts',(0.12927890500043,0.198855929514595,-0.310333816342355));
#81666=CARTESIAN_POINT('Ctrl Pts',(0.143531765398326,0.189402797415757,
-0.311448461280709));
#81667=CARTESIAN_POINT('Ctrl Pts',(0.155166284561794,0.179995371079051,
-0.312358127668875));
#81668=CARTESIAN_POINT('Ctrl Pts',(0.177200036976499,0.158444388930571,
-0.314248327045214));
#81669=CARTESIAN_POINT('Ctrl Pts',(0.187413037060893,0.146221559955588,
-0.31522627794353));
#81670=CARTESIAN_POINT('Ctrl Pts',(0.197898272716074,0.130752048413538,
-0.316438274970184));
#81671=CARTESIAN_POINT('Ctrl Pts',(0.199428396994282,0.128406144338102,
-0.316621326644017));
#81672=CARTESIAN_POINT('Ctrl Pts',(0.201796128833071,0.124631627794973,
-0.31691500223915));
#81673=CARTESIAN_POINT('Ctrl Pts',(0.202660965195212,0.123220344145537,
-0.317024621216795));
#81674=CARTESIAN_POINT('Ctrl Pts',(0.204271501626648,0.120529364084131,
-0.317233352126886));
#81675=CARTESIAN_POINT('Ctrl Pts',(0.205020127302784,0.119251504029019,
-0.317332351464893));
#81676=CARTESIAN_POINT('Ctrl Pts',(0.206699401028356,0.11632252715147,-0.317559040102009));
#81677=CARTESIAN_POINT('Ctrl Pts',(0.207622313192363,0.114667115648396,
-0.317686998882905));
#81678=CARTESIAN_POINT('Ctrl Pts',(0.209993279512116,0.110291871343819,
-0.318024856183737));
#81679=CARTESIAN_POINT('Ctrl Pts',(0.211408303113036,0.107554647299553,
-0.318235891834305));
#81680=CARTESIAN_POINT('Ctrl Pts',(0.220093510702782,0.0899200009154866,
-0.319593910405852));
#81681=CARTESIAN_POINT('Ctrl Pts',(0.225837072913105,0.0743249208342053,
-0.320792519713154));
#81682=CARTESIAN_POINT('Ctrl Pts',(0.233194449599296,0.0452918296322218,
-0.322978693785453));
#81683=CARTESIAN_POINT('Ctrl Pts',(0.235378100138485,0.0320658496346263,
-0.323957191538426));
#81684=CARTESIAN_POINT('Ctrl Pts',(0.23659559034029,0.0166931846818326,
-0.325032039068426));
#81685=CARTESIAN_POINT('Ctrl Pts',(0.236730329093093,0.0146590506293287,
-0.325172984316573));
#81686=CARTESIAN_POINT('Ctrl Pts',(0.236893215690123,0.0116029780654488,
-0.325382574634235));
#81687=CARTESIAN_POINT('Ctrl Pts',(0.2369410074006,0.0105822421729668,-0.325452216171253));
#81688=CARTESIAN_POINT('Ctrl Pts',(0.237015650075542,0.00873216322104528,
-0.3255777469698));
#81689=CARTESIAN_POINT('Ctrl Pts',(0.237044747402458,0.00790296359198541,
-0.325633753467595));
#81690=CARTESIAN_POINT('Ctrl Pts',(0.237100729613421,0.00602673356105983,
-0.325759907420457));
#81691=CARTESIAN_POINT('Ctrl Pts',(0.237125031534582,0.0049796610259576,
-0.325829912724129));
#81692=CARTESIAN_POINT('Ctrl Pts',(0.237178362713998,0.00176356806922175,
-0.326043807821247));
#81693=CARTESIAN_POINT('Ctrl Pts',(0.237184573830235,-0.000405786584734266,
-0.326186513199995));
#81694=CARTESIAN_POINT('Ctrl Pts',(0.236997365511169,-0.0176478373770175,
-0.327310400882714));
#81695=CARTESIAN_POINT('Ctrl Pts',(0.23539712196086,-0.0326728870351739,
-0.328228446985695));
#81696=CARTESIAN_POINT('Ctrl Pts',(0.22922884080715,-0.0628838900572946,
-0.330119553265089));
#81697=CARTESIAN_POINT('Ctrl Pts',(0.224546803012788,-0.0779672542575167,
-0.331089803351203));
#81698=CARTESIAN_POINT('Ctrl Pts',(0.217313081367398,-0.0950517779112877,
-0.332293045867123));
#81699=CARTESIAN_POINT('Ctrl Pts',(0.216176194067849,-0.0976097733871866,
-0.332475998376491));
#81700=CARTESIAN_POINT('Ctrl Pts',(0.214295579824038,-0.101647054202413,
-0.332769552101947));
#81701=CARTESIAN_POINT('Ctrl Pts',(0.213581154359888,-0.103139756781484,
-0.332879149852138));
#81702=CARTESIAN_POINT('Ctrl Pts',(0.212197843102551,-0.105953997307736,
-0.333087863937538));
#81703=CARTESIAN_POINT('Ctrl Pts',(0.211532081613161,-0.107276989332966,
-0.333186867930015));
#81704=CARTESIAN_POINT('Ctrl Pts',(0.209985945376274,-0.110279089698537,
-0.333413600520709));
#81705=CARTESIAN_POINT('Ctrl Pts',(0.209097749912335,-0.111954032976298,
-0.333541598990835));
#81706=CARTESIAN_POINT('Ctrl Pts',(0.206712601455663,-0.116324490267696,
-0.333879633991582));
#81707=CARTESIAN_POINT('Ctrl Pts',(0.205183041720243,-0.119001699484301,
-0.334090809600304));
#81708=CARTESIAN_POINT('Ctrl Pts',(0.195124766642023,-0.13583616441064,
-0.335445608342885));
#81709=CARTESIAN_POINT('Ctrl Pts',(0.185189378096135,-0.149096784624521,
-0.336640516861855));
#81710=CARTESIAN_POINT('Ctrl Pts',(0.164833840858079,-0.171061400033419,
-0.338826345686244));
#81711=CARTESIAN_POINT('Ctrl Pts',(0.154888436952225,-0.180116178070267,
-0.339808246668663));
#81712=CARTESIAN_POINT('Ctrl Pts',(0.142610835718936,-0.189521205107273,
-0.340886243862465));
#81713=CARTESIAN_POINT('Ctrl Pts',(0.140976283305255,-0.190740205227509,
-0.341027221409113));
#81714=CARTESIAN_POINT('Ctrl Pts',(0.138499149962718,-0.192538334836794,
-0.341236849740157));
#81715=CARTESIAN_POINT('Ctrl Pts',(0.137668261964386,-0.193133308021363,
-0.341306497512754));
#81716=CARTESIAN_POINT('Ctrl Pts',(0.13615583113173,-0.194201592933205,
-0.341432034339472));
#81717=CARTESIAN_POINT('Ctrl Pts',(0.13547563034235,-0.194676713249751,
-0.341488040696597));
#81718=CARTESIAN_POINT('Ctrl Pts',(0.133931262067865,-0.195743440068335,
-0.341614187851057));
#81719=CARTESIAN_POINT('Ctrl Pts',(0.133065656027571,-0.196332902434561,
-0.341684186568501));
#81720=CARTESIAN_POINT('Ctrl Pts',(0.130395619751379,-0.198125379449999,
-0.341898040608991));
#81721=CARTESIAN_POINT('Ctrl Pts',(0.128578513749884,-0.199309433413533,
-0.342040712173639));
#81722=CARTESIAN_POINT('Ctrl Pts',(0.113995770282891,-0.208529312537002,
-0.343165248683038));
#81723=CARTESIAN_POINT('Ctrl Pts',(0.10050445425452,-0.215356657366352,
-0.344083885091623));
#81724=CARTESIAN_POINT('Ctrl Pts',(0.0719574549628525,-0.226531385666714,
-0.345964079833396));
#81725=CARTESIAN_POINT('Ctrl Pts',(0.0569389721016377,-0.230764414914573,
-0.346922668523748));
#81726=CARTESIAN_POINT('Ctrl Pts',(0.0387637899545327,-0.234003712007533,
-0.348118793231333));
#81727=CARTESIAN_POINT('Ctrl Pts',(0.0359035505199509,-0.234459596772095,
-0.348307944715936));
#81728=CARTESIAN_POINT('Ctrl Pts',(0.031376679006716,-0.235096345591903,
-0.348609107946534));
#81729=CARTESIAN_POINT('Ctrl Pts',(0.0297151904271129,-0.235312122322688,
-0.348720021898876));
#81730=CARTESIAN_POINT('Ctrl Pts',(0.0265843208329051,-0.235685039690455,
-0.348929802641364));
#81731=CARTESIAN_POINT('Ctrl Pts',(0.0251154794176729,-0.235846086615878,
-0.349028541592293));
#81732=CARTESIAN_POINT('Ctrl Pts',(0.0217925963526855,-0.23617902146097,
-0.349252682596646));
#81733=CARTESIAN_POINT('Ctrl Pts',(0.0199378613752886,-0.236342820442584,
-0.349378331574464));
#81734=CARTESIAN_POINT('Ctrl Pts',(0.0151239323796517,-0.236710889589636,
-0.349705930961519));
#81735=CARTESIAN_POINT('Ctrl Pts',(0.0121625701170361,-0.236881508543861,
-0.349908909017341));
#81736=CARTESIAN_POINT('Ctrl Pts',(-0.00899732842890131,-0.237702819168099,
-0.351370133998079));
#81737=CARTESIAN_POINT('Ctrl Pts',(-0.0272112440068833,-0.236311007626842,
-0.352692305438812));
#81738=CARTESIAN_POINT('Ctrl Pts',(-0.0568483972826379,-0.230572894833667,
-0.354895619269897));
#81739=CARTESIAN_POINT('Ctrl Pts',(-0.0684256939039571,-0.227406206223094,
-0.355768100042965));
#81740=CARTESIAN_POINT('Ctrl Pts',(-0.0816212137539605,-0.222697226599945,
-0.356744476529759));
#81741=CARTESIAN_POINT('Ctrl Pts',(-0.0835187791176015,-0.221992548265628,
-0.356884406017405));
#81742=CARTESIAN_POINT('Ctrl Pts',(-0.0863577643822186,-0.220896707593825,
-0.357092796561104));
#81743=CARTESIAN_POINT('Ctrl Pts',(-0.0873060087839281,-0.220523649121268,
-0.3571622379));
#81744=CARTESIAN_POINT('Ctrl Pts',(-0.0890220557447235,-0.219835717711923,
-0.357287572559194));
#81745=CARTESIAN_POINT('Ctrl Pts',(-0.089790632133962,-0.219522918211441,
-0.357343581002454));
#81746=CARTESIAN_POINT('Ctrl Pts',(-0.0915284653788229,-0.218804991071039,
-0.357469943850697));
#81747=CARTESIAN_POINT('Ctrl Pts',(-0.0924966881684012,-0.218397451620967,
-0.357540153849912));
#81748=CARTESIAN_POINT('Ctrl Pts',(-0.0954709386570211,-0.217122217495248,
-0.357755331342528));
#81749=CARTESIAN_POINT('Ctrl Pts',(-0.0974677699745459,-0.216233189185981,
-0.357899093783551));
#81750=CARTESIAN_POINT('Ctrl Pts',(-0.112828832734564,-0.20913810312954,
-0.359001713644842));
#81751=CARTESIAN_POINT('Ctrl Pts',(-0.125602570435149,-0.201725566547404,
-0.359900411589748));
#81752=CARTESIAN_POINT('Ctrl Pts',(-0.150471696916894,-0.184010142553203,
-0.361772908805763));
#81753=CARTESIAN_POINT('Ctrl Pts',(-0.162387222234084,-0.173585055958464,
-0.362744184737375));
#81754=CARTESIAN_POINT('Ctrl Pts',(-0.175192874676087,-0.159900393967547,
-0.363957810890037));
#81755=CARTESIAN_POINT('Ctrl Pts',(-0.177167651876346,-0.157709546972967,
-0.364150354506782));
#81756=CARTESIAN_POINT('Ctrl Pts',(-0.180206689772604,-0.154208865985483,
-0.364455680534753));
#81757=CARTESIAN_POINT('Ctrl Pts',(-0.181298743208269,-0.152923480380442,
-0.364567312004296));
#81758=CARTESIAN_POINT('Ctrl Pts',(-0.183320716388196,-0.150491444160723,
-0.364777704068082));
#81759=CARTESIAN_POINT('Ctrl Pts',(-0.184253824306558,-0.149347540595696,
-0.364876328565223));
#81760=CARTESIAN_POINT('Ctrl Pts',(-0.18632909156537,-0.146754403212297,
-0.365099203826542));
#81761=CARTESIAN_POINT('Ctrl Pts',(-0.187465128034384,-0.145300415219578,
-0.365223690170512));
#81762=CARTESIAN_POINT('Ctrl Pts',(-0.190348086560378,-0.141520485216699,
-0.365546167866041));
#81763=CARTESIAN_POINT('Ctrl Pts',(-0.192069346640967,-0.139175452478701,
-0.365745134118932));
#81764=CARTESIAN_POINT('Ctrl Pts',(-0.206226152748358,-0.11912538256697,
-0.367437797750914));
#81765=CARTESIAN_POINT('Ctrl Pts',(-0.216226212613638,-0.0998294975689819,
-0.369025617893774));
#81766=CARTESIAN_POINT('Ctrl Pts',(-0.225576756778854,-0.0735297021672426,
-0.371054503469704));
#81767=CARTESIAN_POINT('Ctrl Pts',(-0.227446285401341,-0.0675254581974951,
-0.371508238048471));
#81768=CARTESIAN_POINT('Ctrl Pts',(-0.229732408050907,-0.0590036928393934,
-0.372133437064782));
#81769=CARTESIAN_POINT('Ctrl Pts',(-0.230350346826438,-0.0565432039888334,
-0.372311786264622));
#81770=CARTESIAN_POINT('Ctrl Pts',(-0.231369574270329,-0.0521904190140774,
-0.372622969092079));
#81771=CARTESIAN_POINT('Ctrl Pts',(-0.231787406936192,-0.0503022695201936,
-0.37275653137942));
#81772=CARTESIAN_POINT('Ctrl Pts',(-0.232386378680184,-0.0474294544524633,
-0.372957381533114));
#81773=CARTESIAN_POINT('Ctrl Pts',(-0.232584443055373,-0.0464484562307289,
-0.373025550821621));
#81774=CARTESIAN_POINT('Ctrl Pts',(-0.232935556149919,-0.0446508398639056,
-0.37314966958429));
#81775=CARTESIAN_POINT('Ctrl Pts',(-0.23309052732003,-0.0438346544808771,
-0.373205720629513));
#81776=CARTESIAN_POINT('Ctrl Pts',(-0.233435647618594,-0.0419634152558728,
-0.373333544425463));
#81777=CARTESIAN_POINT('Ctrl Pts',(-0.233622935946281,-0.0409078685523452,
-0.37340515741755));
#81778=CARTESIAN_POINT('Ctrl Pts',(-0.234189554032502,-0.0375835646168496,
-0.373629253886288));
#81779=CARTESIAN_POINT('Ctrl Pts',(-0.234543053375111,-0.0353104605006836,
-0.373780383812952));
#81780=CARTESIAN_POINT('Ctrl Pts',(-0.236392755853335,-0.0221589320369147,
-0.374644540480458));
#81781=CARTESIAN_POINT('Ctrl Pts',(-0.237165284880642,-0.0111909665116149,
-0.37532525327104));
#81782=CARTESIAN_POINT('Ctrl Pts',(-0.237191493369619,0.0187185899535097,
-0.377164510361014));
#81783=CARTESIAN_POINT('Ctrl Pts',(-0.234942750240432,0.0375768454921921,
-0.378311200860805));
#81784=CARTESIAN_POINT('Ctrl Pts',(-0.229795218082391,0.0587748961201941,
-0.37972022844811));
#81785=CARTESIAN_POINT('Ctrl Pts',(-0.229062104665875,0.0615701365391166,
-0.379908353209227));
#81786=CARTESIAN_POINT('Ctrl Pts',(-0.227779024317824,0.0661217101173076,
-0.380218886285169));
#81787=CARTESIAN_POINT('Ctrl Pts',(-0.227259349215754,0.0678863192732277,
-0.380340322820557));
#81788=CARTESIAN_POINT('Ctrl Pts',(-0.226285862923904,0.0710553781983971,
-0.380560387944717));
#81789=CARTESIAN_POINT('Ctrl Pts',(-0.225839364538556,0.0724619885642481,
-0.380658774060869));
#81790=CARTESIAN_POINT('Ctrl Pts',(-0.224853275206923,0.0754708108511365,
-0.380870797048019));
#81791=CARTESIAN_POINT('Ctrl Pts',(-0.22430962432184,0.0770715955594267,
-0.380984562659641));
#81792=CARTESIAN_POINT('Ctrl Pts',(-0.222764472840155,0.0814664323528264,
-0.381299630123455));
#81793=CARTESIAN_POINT('Ctrl Pts',(-0.221727594261927,0.0842476261770411,
-0.38150208632574));
#81794=CARTESIAN_POINT('Ctrl Pts',(-0.219294058701362,0.0904186589882814,
-0.381958411186321));
#81795=CARTESIAN_POINT('Ctrl Pts',(-0.217870466972286,0.0937969892427897,
-0.382213116366277));
#81796=CARTESIAN_POINT('Ctrl Pts',(-0.212986009098468,0.104676517985949,
-0.38304953251337));
#81797=CARTESIAN_POINT('Ctrl Pts',(-0.209211739274275,0.112029633332087,
-0.383640581428881));
#81798=CARTESIAN_POINT('Ctrl Pts',(-0.196160273416756,0.134487904265748,
-0.385521508250884));
#81799=CARTESIAN_POINT('Ctrl Pts',(-0.185570382196961,0.148759914260615,
-0.386834955047876));
#81800=CARTESIAN_POINT('Ctrl Pts',(-0.171648423741659,0.163695118860609,
-0.38826959436283));
#81801=CARTESIAN_POINT('Ctrl Pts',(-0.169773365624433,0.165639002527922,
-0.388457540313142));
#81802=CARTESIAN_POINT('Ctrl Pts',(-0.167114535338839,0.168302829685472,
-0.388716303540888));
#81803=CARTESIAN_POINT('Ctrl Pts',(-0.166358584181959,0.16905008718543,
-0.38878902830247));
#81804=CARTESIAN_POINT('Ctrl Pts',(-0.164988781964261,0.170386049085651,
-0.388919252011855));
#81805=CARTESIAN_POINT('Ctrl Pts',(-0.164376740598118,0.170976580654513,
-0.388976887572525));
#81806=CARTESIAN_POINT('Ctrl Pts',(-0.163110170091353,0.172185550590766,
-0.389095010160604));
#81807=CARTESIAN_POINT('Ctrl Pts',(-0.162455274465474,0.172803574285227,
-0.389155466703759));
#81808=CARTESIAN_POINT('Ctrl Pts',(-0.160726859932221,0.174416165033227,
-0.389313456883498));
#81809=CARTESIAN_POINT('Ctrl Pts',(-0.159647608707725,0.175404570720446,
-0.389410539540783));
#81810=CARTESIAN_POINT('Ctrl Pts',(-0.154553642300095,0.179983785697007,
-0.389861871671207));
#81811=CARTESIAN_POINT('Ctrl Pts',(-0.150426187316355,0.183447441148556,
-0.390207809704147));
#81812=CARTESIAN_POINT('Ctrl Pts',(-0.137015780565877,0.193943827601388,
-0.391284185469541));
#81813=CARTESIAN_POINT('Ctrl Pts',(-0.12733098548676,0.20043549773552,-0.391993687697713));
#81814=CARTESIAN_POINT('Ctrl Pts',(-0.105223255307046,0.213002567344061,
-0.393554017526574));
#81815=CARTESIAN_POINT('Ctrl Pts',(-0.0926687609802247,0.218756640405711,
-0.394404727205633));
#81816=CARTESIAN_POINT('Ctrl Pts',(-0.0767126472496483,0.224448478057488,
-0.395496024686669));
#81817=CARTESIAN_POINT('Ctrl Pts',(-0.07371806084191,0.225449762830957,
-0.395701147488995));
#81818=CARTESIAN_POINT('Ctrl Pts',(-0.0688941546345913,0.226956324106241,
-0.396032569872519));
#81819=CARTESIAN_POINT('Ctrl Pts',(-0.067077150095072,0.227499963039657,
-0.396157627081568));
#81820=CARTESIAN_POINT('Ctrl Pts',(-0.063826228876646,0.22843029175073,
-0.396381865089275));
#81821=CARTESIAN_POINT('Ctrl Pts',(-0.0623948167249027,0.228825418947979,
-0.396480766970879));
#81822=CARTESIAN_POINT('Ctrl Pts',(-0.0593775881632067,0.229627879782371,
-0.396689636329218));
#81823=CARTESIAN_POINT('Ctrl Pts',(-0.0577910809438523,0.230032284430195,
-0.396799692364146));
#81824=CARTESIAN_POINT('Ctrl Pts',(-0.0535615332678821,0.231063890482319,
-0.397093766576584));
#81825=CARTESIAN_POINT('Ctrl Pts',(-0.0509117554811016,0.231662149304147,
-0.397278696334734));
#81826=CARTESIAN_POINT('Ctrl Pts',(-0.0461519654293381,0.232651195874028,
-0.397612253452573));
#81827=CARTESIAN_POINT('Ctrl Pts',(-0.0440462491475563,0.233059018734323,
-0.397760292373697));
#81828=CARTESIAN_POINT('Ctrl Pts',(-0.0419358190075303,0.23343814536011,
-0.397909151625197));
#81829=CARTESIAN_POINT('',(-0.237174999987694,-2.41604215922389E-6,-0.395881110820101));
#81830=CARTESIAN_POINT('Ctrl Pts',(-0.0419358280420692,0.233438143737107,
-0.417646538149483));
#81831=CARTESIAN_POINT('Ctrl Pts',(-0.0483941564159259,0.232277941964639,
-0.417230281189441));
#81832=CARTESIAN_POINT('Ctrl Pts',(-0.0548034836274561,0.230849877704686,
-0.416822836231435));
#81833=CARTESIAN_POINT('Ctrl Pts',(-0.0788615774794773,0.224430337698852,
-0.41528836043212));
#81834=CARTESIAN_POINT('Ctrl Pts',(-0.0959667408439773,0.217665948128303,
-0.414181402220041));
#81835=CARTESIAN_POINT('Ctrl Pts',(-0.115849964572538,0.20699919152677,
-0.412736627724306));
#81836=CARTESIAN_POINT('Ctrl Pts',(-0.119523702368301,0.20489987955341,
-0.412462752788253));
#81837=CARTESIAN_POINT('Ctrl Pts',(-0.124774783994876,0.201709931403471,
-0.4120599376928));
#81838=CARTESIAN_POINT('Ctrl Pts',(-0.126398277385047,0.200696582596506,
-0.411933776238562));
#81839=CARTESIAN_POINT('Ctrl Pts',(-0.129261025383699,0.198861204898509,
-0.411708309998145));
#81840=CARTESIAN_POINT('Ctrl Pts',(-0.130505160002671,0.19804695033732,
-0.411609295859604));
#81841=CARTESIAN_POINT('Ctrl Pts',(-0.133095031755873,0.196316944111657,
-0.411400970105855));
#81842=CARTESIAN_POINT('Ctrl Pts',(-0.134439157830142,0.19539893202587,
-0.411291577185917));
#81843=CARTESIAN_POINT('Ctrl Pts',(-0.137965456980013,0.192936929492227,
-0.411001137208692));
#81844=CARTESIAN_POINT('Ctrl Pts',(-0.140131105597443,0.191369794667348,
-0.410819217769311));
#81845=CARTESIAN_POINT('Ctrl Pts',(-0.151519566253012,0.182831756154235,
-0.409843069200494));
#81846=CARTESIAN_POINT('Ctrl Pts',(-0.160248600106373,0.175231116741886,
-0.40902440537741));
#81847=CARTESIAN_POINT('Ctrl Pts',(-0.174632194790189,0.160730212548615,
-0.407549105142471));
#81848=CARTESIAN_POINT('Ctrl Pts',(-0.180518482802464,0.154089818467004,
-0.406900553218716));
#81849=CARTESIAN_POINT('Ctrl Pts',(-0.193047831359062,0.138249370361049,
-0.405427567273631));
#81850=CARTESIAN_POINT('Ctrl Pts',(-0.19943171814169,0.12886970325819,-0.404605931764943));
#81851=CARTESIAN_POINT('Ctrl Pts',(-0.205984989500111,0.117580296747157,
-0.403699690114774));
#81852=CARTESIAN_POINT('Ctrl Pts',(-0.206832732350692,0.116082571212904,
-0.403581062139185));
#81853=CARTESIAN_POINT('Ctrl Pts',(-0.208130962768453,0.113729577578987,
-0.403397329401662));
#81854=CARTESIAN_POINT('Ctrl Pts',(-0.208592632349877,0.112880593069727,
-0.403331566013175));
#81855=CARTESIAN_POINT('Ctrl Pts',(-0.209403901641078,0.111366740061696,
-0.403215270377044));
#81856=CARTESIAN_POINT('Ctrl Pts',(-0.209755537858412,0.110703022431092,
-0.403164614249093));
#81857=CARTESIAN_POINT('Ctrl Pts',(-0.210600800098982,0.109089092487864,
-0.403042224241637));
#81858=CARTESIAN_POINT('Ctrl Pts',(-0.211091152667851,0.108137192851263,
-0.402970693582124));
#81859=CARTESIAN_POINT('Ctrl Pts',(-0.21261191762856,0.105135233741133,
-0.402747059652105));
#81860=CARTESIAN_POINT('Ctrl Pts',(-0.213619074247803,0.103073454206785,
-0.402596302356005));
#81861=CARTESIAN_POINT('Ctrl Pts',(-0.218890923811409,0.09187197693539,
-0.401790705884823));
#81862=CARTESIAN_POINT('Ctrl Pts',(-0.222599727624839,0.0824809305655365,
-0.401162921282223));
#81863=CARTESIAN_POINT('Ctrl Pts',(-0.231717481545343,0.0542449732917915,
-0.399334907779679));
#81864=CARTESIAN_POINT('Ctrl Pts',(-0.235403594222045,0.0349369987405584,
-0.398152900227539));
#81865=CARTESIAN_POINT('Ctrl Pts',(-0.236888596139364,0.012108871306242,
-0.396677277300176));
#81866=CARTESIAN_POINT('Ctrl Pts',(-0.237033915765791,0.00881775525041497,
-0.396462892892614));
#81867=CARTESIAN_POINT('Ctrl Pts',(-0.237136523561489,0.00441408874215108,
-0.396173378021457));
#81868=CARTESIAN_POINT('Ctrl Pts',(-0.237154598636204,0.00330321997630701,
-0.396100119721302));
#81869=CARTESIAN_POINT('Ctrl Pts',(-0.237171630092345,0.00146072643667166,
-0.395978221412552));
#81870=CARTESIAN_POINT('Ctrl Pts',(-0.237175007440005,0.00072915308448074,
-0.395929718572334));
#81871=CARTESIAN_POINT('Ctrl Pts',(-0.237174999987694,-2.41604215922389E-6,
-0.395881110820101));
#81872=CARTESIAN_POINT('Ctrl Pts',(-0.237174999987369,-2.44774490620395E-6,
-0.395881108713671));
#81873=CARTESIAN_POINT('Ctrl Pts',(-0.237174993974579,-0.000585058863951221,
-0.395842398197246));
#81874=CARTESIAN_POINT('Ctrl Pts',(-0.237172841219915,-0.00116766457214191,
-0.395803621328249));
#81875=CARTESIAN_POINT('Ctrl Pts',(-0.237161772411672,-0.00266754656485543,
-0.395703617536787));
#81876=CARTESIAN_POINT('Ctrl Pts',(-0.237149681418993,-0.00358478177326851,
-0.39564229268734));
#81877=CARTESIAN_POINT('Ctrl Pts',(-0.237099735243235,-0.00621563015734606,
-0.395465900968798));
#81878=CARTESIAN_POINT('Ctrl Pts',(-0.237048625224458,-0.00792890424153297,
-0.395350424275536));
#81879=CARTESIAN_POINT('Ctrl Pts',(-0.23685292236543,-0.0127391275306386,
-0.395024435453109));
#81880=CARTESIAN_POINT('Ctrl Pts',(-0.236666173587936,-0.0158339162863413,
-0.394812629851663));
#81881=CARTESIAN_POINT('Ctrl Pts',(-0.234832601539564,-0.0387408175958628,
-0.393228832044568));
#81882=CARTESIAN_POINT('Ctrl Pts',(-0.23076131366614,-0.058276175430853,
-0.391779006268009));
#81883=CARTESIAN_POINT('Ctrl Pts',(-0.221016901985021,-0.0866361353605369,
-0.389592688110286));
#81884=CARTESIAN_POINT('Ctrl Pts',(-0.217121161428312,-0.095982976466006,
-0.388859627519287));
#81885=CARTESIAN_POINT('Ctrl Pts',(-0.211622486291035,-0.107112939240905,
-0.387991666613779));
#81886=CARTESIAN_POINT('Ctrl Pts',(-0.210574986470963,-0.109157842151878,
-0.387832433415779));
#81887=CARTESIAN_POINT('Ctrl Pts',(-0.208995674938438,-0.112133563804,-0.387601409330168));
#81888=CARTESIAN_POINT('Ctrl Pts',(-0.208487040827164,-0.113076444023026,
-0.387528310866675));
#81889=CARTESIAN_POINT('Ctrl Pts',(-0.207610916169756,-0.114674549800816,
-0.387404632389075));
#81890=CARTESIAN_POINT('Ctrl Pts',(-0.207246679373072,-0.115331517079058,
-0.387353853964854));
#81891=CARTESIAN_POINT('Ctrl Pts',(-0.206406909183692,-0.11682936960034,
-0.387238236183036));
#81892=CARTESIAN_POINT('Ctrl Pts',(-0.205929353364056,-0.117669092227257,
-0.387173526025823));
#81893=CARTESIAN_POINT('Ctrl Pts',(-0.20458765041009,-0.119995123437729,
-0.386994510821711));
#81894=CARTESIAN_POINT('Ctrl Pts',(-0.203712433149011,-0.121475023565959,
-0.386880880386286));
#81895=CARTESIAN_POINT('Ctrl Pts',(-0.197027683394357,-0.132502760768627,
-0.386035123330123));
#81896=CARTESIAN_POINT('Ctrl Pts',(-0.190565080013029,-0.141640056492486,
-0.385339569328659));
#81897=CARTESIAN_POINT('Ctrl Pts',(-0.177889010979282,-0.157115773896804,
-0.384107670433089));
#81898=CARTESIAN_POINT('Ctrl Pts',(-0.171920076202272,-0.163625653209715,
-0.383569640121974));
#81899=CARTESIAN_POINT('Ctrl Pts',(-0.160008888310081,-0.175243214047791,
-0.382542961627802));
#81900=CARTESIAN_POINT('Ctrl Pts',(-0.154149743607366,-0.180418600405547,
-0.382056402338797));
#81901=CARTESIAN_POINT('Ctrl Pts',(-0.145281232134576,-0.187504318853361,
-0.381334621668707));
#81902=CARTESIAN_POINT('Ctrl Pts',(-0.142467274622731,-0.189651205457337,
-0.381107628539409));
#81903=CARTESIAN_POINT('Ctrl Pts',(-0.137271783344386,-0.193434170918486,
-0.380691200948543));
#81904=CARTESIAN_POINT('Ctrl Pts',(-0.134906359347164,-0.195091245350535,
-0.380502575621173));
#81905=CARTESIAN_POINT('Ctrl Pts',(-0.131123503851417,-0.197639590092998,
-0.38020207844178));
#81906=CARTESIAN_POINT('Ctrl Pts',(-0.129725833889909,-0.198559785996061,
-0.380091296432875));
#81907=CARTESIAN_POINT('Ctrl Pts',(-0.127076053231611,-0.200264425458137,
-0.379881660685141));
#81908=CARTESIAN_POINT('Ctrl Pts',(-0.125826116327033,-0.201052111875229,
-0.379782933554974));
#81909=CARTESIAN_POINT('Ctrl Pts',(-0.122982905127233,-0.202806950995464,
-0.379558677108675));
#81910=CARTESIAN_POINT('Ctrl Pts',(-0.121385441637704,-0.203767093859447,
-0.379432899391021));
#81911=CARTESIAN_POINT('Ctrl Pts',(-0.117210453102132,-0.206209921428293,
-0.379104666458924));
#81912=CARTESIAN_POINT('Ctrl Pts',(-0.114616133542342,-0.20766309868266,
-0.378901176574523));
#81913=CARTESIAN_POINT('Ctrl Pts',(-0.0960223525775907,-0.21762361395977,
-0.377445516736402));
#81914=CARTESIAN_POINT('Ctrl Pts',(-0.0791241837443924,-0.224319991031289,
-0.376130139497006));
#81915=CARTESIAN_POINT('Ctrl Pts',(-0.0497411862481437,-0.232227129515415,
-0.3739091874719));
#81916=CARTESIAN_POINT('Ctrl Pts',(-0.0376173718029788,-0.23449652921264,
-0.373012471423046));
#81917=CARTESIAN_POINT('Ctrl Pts',(-0.0235130872898481,-0.236013998223146,
-0.372025889664875));
#81918=CARTESIAN_POINT('Ctrl Pts',(-0.0216527479674377,-0.236191938218795,
-0.371896903655876));
#81919=CARTESIAN_POINT('Ctrl Pts',(-0.0188066256142253,-0.236430256340702,
-0.371701506288426));
#81920=CARTESIAN_POINT('Ctrl Pts',(-0.0178222949964452,-0.236506492870208,
-0.371634281665537));
#81921=CARTESIAN_POINT('Ctrl Pts',(-0.0160077947327807,-0.23663563345837,
-0.371511046849067));
#81922=CARTESIAN_POINT('Ctrl Pts',(-0.015177809912862,-0.23669031800133,
-0.371454945134281));
#81923=CARTESIAN_POINT('Ctrl Pts',(-0.0132784714627283,-0.23680542618126,
-0.371327159705849));
#81924=CARTESIAN_POINT('Ctrl Pts',(-0.0122089772759333,-0.236862974432931,
-0.371255634383294));
#81925=CARTESIAN_POINT('Ctrl Pts',(-0.00886793475978442,-0.23702006238442,
-0.371033429807722));
#81926=CARTESIAN_POINT('Ctrl Pts',(-0.00659524485003055,-0.237094187847428,
-0.370884062621256));
#81927=CARTESIAN_POINT('Ctrl Pts',(0.00675570713104867,-0.237337505760676,
-0.370015227401446));
#81928=CARTESIAN_POINT('Ctrl Pts',(0.0178350639157828,-0.236762961152023,
-0.369328709654773));
#81929=CARTESIAN_POINT('Ctrl Pts',(0.0382324760196458,-0.234264594675536,
-0.368065243619044));
#81930=CARTESIAN_POINT('Ctrl Pts',(0.0475526833224055,-0.232551847795849,
-0.36748803611714));
#81931=CARTESIAN_POINT('Ctrl Pts',(0.0634779240609387,-0.228627670120237,
-0.36647197562288));
#81932=CARTESIAN_POINT('Ctrl Pts',(0.0701339394012187,-0.226674388421198,
-0.366038036275399));
#81933=CARTESIAN_POINT('Ctrl Pts',(0.0812158685449806,-0.22288740050702,
-0.365291233632475));
#81934=CARTESIAN_POINT('Ctrl Pts',(0.0856892424813818,-0.221206146781791,
-0.364982872399261));
#81935=CARTESIAN_POINT('Ctrl Pts',(0.091982764675391,-0.218621263392434,
-0.364537440056293));
#81936=CARTESIAN_POINT('Ctrl Pts',(0.0938469744334933,-0.217827525289157,
-0.364404019639248));
#81937=CARTESIAN_POINT('Ctrl Pts',(0.0970719794289436,-0.216405308185208,
-0.364170504774761));
#81938=CARTESIAN_POINT('Ctrl Pts',(0.0984374293911331,-0.215787624576422,
-0.364070781131217));
#81939=CARTESIAN_POINT('Ctrl Pts',(0.101068608136367,-0.214567197463086,
-0.363876911924916));
#81940=CARTESIAN_POINT('Ctrl Pts',(0.102335029862304,-0.213966089124163,
-0.363782825904919));
#81941=CARTESIAN_POINT('Ctrl Pts',(0.105700619898416,-0.212331893952013,
-0.363530671094749));
#81942=CARTESIAN_POINT('Ctrl Pts',(0.107789910343504,-0.21127893596652,
-0.363371919606703));
#81943=CARTESIAN_POINT('Ctrl Pts',(0.115664714784849,-0.207162994895937,
-0.362764878063084));
#81944=CARTESIAN_POINT('Ctrl Pts',(0.121337654230917,-0.203892109137735,
-0.36230941781622));
#81945=CARTESIAN_POINT('Ctrl Pts',(0.141629542878925,-0.191045310288335,
-0.360611635300381));
#81946=CARTESIAN_POINT('Ctrl Pts',(0.155312416164008,-0.18009763042746,
-0.359325138942754));
#81947=CARTESIAN_POINT('Ctrl Pts',(0.171776699757586,-0.163641402702207,
-0.357635966006275));
#81948=CARTESIAN_POINT('Ctrl Pts',(0.17573432256495,-0.159383812274255,
-0.357217517641067));
#81949=CARTESIAN_POINT('Ctrl Pts',(0.181843129396594,-0.152307477944915,
-0.356556107030273));
#81950=CARTESIAN_POINT('Ctrl Pts',(0.184094446661538,-0.149578506136751,
-0.35630864322923));
#81951=CARTESIAN_POINT('Ctrl Pts',(0.187067664509862,-0.145805598354543,
-0.355977780911847));
#81952=CARTESIAN_POINT('Ctrl Pts',(0.187843362624387,-0.144804885670027,
-0.355891068520842));
#81953=CARTESIAN_POINT('Ctrl Pts',(0.189131488712093,-0.143115329341787,
-0.355746475702147));
#81954=CARTESIAN_POINT('Ctrl Pts',(0.189648250690643,-0.142429837514248,
-0.355688303685997));
#81955=CARTESIAN_POINT('Ctrl Pts',(0.190701049408829,-0.141017396395389,
-0.355569472246095));
#81956=CARTESIAN_POINT('Ctrl Pts',(0.191236673278507,-0.140290167843728,
-0.355508840019971));
#81957=CARTESIAN_POINT('Ctrl Pts',(0.192637012331282,-0.138365972917941,
-0.355349805070545));
#81958=CARTESIAN_POINT('Ctrl Pts',(0.193494742432673,-0.137163938068432,
-0.355251864452558));
#81959=CARTESIAN_POINT('Ctrl Pts',(0.197208019048673,-0.131855943819113,
-0.354825130352847));
#81960=CARTESIAN_POINT('Ctrl Pts',(0.199944723020725,-0.127667962240653,
-0.354503383072239));
#81961=CARTESIAN_POINT('Ctrl Pts',(0.210455794275979,-0.110414701567894,
-0.353223602361746));
#81962=CARTESIAN_POINT('Ctrl Pts',(0.217098665669008,-0.0967020480646991,
-0.352307009499785));
#81963=CARTESIAN_POINT('Ctrl Pts',(0.225774312722978,-0.0733013063227795,
-0.350768079017187));
#81964=CARTESIAN_POINT('Ctrl Pts',(0.228597312827624,-0.0639559467898985,
-0.350159990894307));
#81965=CARTESIAN_POINT('Ctrl Pts',(0.231763926708487,-0.050534748710045,
-0.349275668647977));
#81966=CARTESIAN_POINT('Ctrl Pts',(0.232590464665895,-0.0465827352123217,
-0.349014030468047));
#81967=CARTESIAN_POINT('Ctrl Pts',(0.233657086023342,-0.0407425708161299,
-0.348624589016904));
#81968=CARTESIAN_POINT('Ctrl Pts',(0.23397597876732,-0.0388694216129775,
-0.34849926427914));
#81969=CARTESIAN_POINT('Ctrl Pts',(0.234503342971433,-0.0355296578314993,
-0.348274977503675));
#81970=CARTESIAN_POINT('Ctrl Pts',(0.234720647558662,-0.0340645253916771,
-0.34817629932733));
#81971=CARTESIAN_POINT('Ctrl Pts',(0.235151214861497,-0.0309615039651739,
-0.347966660475668));
#81972=CARTESIAN_POINT('Ctrl Pts',(0.235361118564136,-0.0293232366562086,
-0.347855599716007));
#81973=CARTESIAN_POINT('Ctrl Pts',(0.235879016549694,-0.0249164482390856,
-0.34755577235751));
#81974=CARTESIAN_POINT('Ctrl Pts',(0.236155367964125,-0.0221445450537729,
-0.347366029599048));
#81975=CARTESIAN_POINT('Ctrl Pts',(0.23751046768031,-0.00560624734037188,
-0.346226658835146));
#81976=CARTESIAN_POINT('Ctrl Pts',(0.237433928022695,0.00822586002365591,
-0.34524138713463));
#81977=CARTESIAN_POINT('Ctrl Pts',(0.235236684636191,0.0318433002732485,
-0.34351778588038));
#81978=CARTESIAN_POINT('Ctrl Pts',(0.233700000996211,0.0416485604805146,
-0.342790382467661));
#81979=CARTESIAN_POINT('Ctrl Pts',(0.230381028079536,0.0566210787946362,
-0.341679370526248));
#81980=CARTESIAN_POINT('Ctrl Pts',(0.229026726820277,0.06187188684724,-0.341289812628266));
#81981=CARTESIAN_POINT('Ctrl Pts',(0.226539582632591,0.0703077412721777,
-0.340668407658541));
#81982=CARTESIAN_POINT('Ctrl Pts',(0.225516589695409,0.0735230004870905,
-0.34043264699572));
#81983=CARTESIAN_POINT('Ctrl Pts',(0.224022930278894,0.0778925842135554,
-0.340114724893984));
#81984=CARTESIAN_POINT('Ctrl Pts',(0.223611312149806,0.0790664860436689,
-0.340029562707809));
#81985=CARTESIAN_POINT('Ctrl Pts',(0.222901488889101,0.0810409558474153,
-0.339886806265693));
#81986=CARTESIAN_POINT('Ctrl Pts',(0.222608163424756,0.0818432400531308,
-0.33982893632245));
#81987=CARTESIAN_POINT('Ctrl Pts',(0.221993270591163,0.083497288927274,
-0.339709931767458));
#81988=CARTESIAN_POINT('Ctrl Pts',(0.221671124477625,0.0843488120177309,
-0.339648831284284));
#81989=CARTESIAN_POINT('Ctrl Pts',(0.220801782097975,0.0866073475331657,
-0.339487155774716));
#81990=CARTESIAN_POINT('Ctrl Pts',(0.220246031454146,0.0880110535381722,
-0.339387070857342));
#81991=CARTESIAN_POINT('Ctrl Pts',(0.217654855955397,0.0943775137010561,
-0.338934539598695));
#81992=CARTESIAN_POINT('Ctrl Pts',(0.215464683960568,0.0992760354568723,
-0.338590237194432));
#81993=CARTESIAN_POINT('Ctrl Pts',(0.20652272585129,0.117582339628132,-0.337303045731337));
#81994=CARTESIAN_POINT('Ctrl Pts',(0.198669760953754,0.130413305210078,
-0.336397946234262));
#81995=CARTESIAN_POINT('Ctrl Pts',(0.184945088287598,0.148690452585697,
-0.334987773883554));
#81996=CARTESIAN_POINT('Ctrl Pts',(0.179925859152281,0.154726235288953,
-0.334499280238685));
#81997=CARTESIAN_POINT('Ctrl Pts',(0.172215736731027,0.163114413980044,
-0.333774917352308));
#81998=CARTESIAN_POINT('Ctrl Pts',(0.169756198608849,0.165672578046288,
-0.333547346141803));
#81999=CARTESIAN_POINT('Ctrl Pts',(0.165188318718798,0.170215083086525,
-0.333129957242076));
#82000=CARTESIAN_POINT('Ctrl Pts',(0.163099248543014,0.1722178535817,-0.332940954623932));
#82001=CARTESIAN_POINT('Ctrl Pts',(0.159744275359288,0.175318428889826,
-0.3326399943499));
#82002=CARTESIAN_POINT('Ctrl Pts',(0.158502445760494,0.176441943609541,
-0.332529132375849));
#82003=CARTESIAN_POINT('Ctrl Pts',(0.156142963260916,0.178531615989263,
-0.332319429764708));
#82004=CARTESIAN_POINT('Ctrl Pts',(0.155027973240739,0.179500669154759,
-0.332220716664099));
#82005=CARTESIAN_POINT('Ctrl Pts',(0.152487404560057,0.181667384353392,
-0.331996607533027));
#82006=CARTESIAN_POINT('Ctrl Pts',(0.151056643554464,0.182858790279001,
-0.331870964414313));
#82007=CARTESIAN_POINT('Ctrl Pts',(0.146640869377827,0.186448647871401,
-0.331484812161052));
#82008=CARTESIAN_POINT('Ctrl Pts',(0.143611800593303,0.188791659351642,
-0.331222136529913));
#82009=CARTESIAN_POINT('Ctrl Pts',(0.125397349609529,0.202188646110562,
-0.329654568159222));
#82010=CARTESIAN_POINT('Ctrl Pts',(0.109001148624927,0.211478722522018,
-0.328283626173752));
#82011=CARTESIAN_POINT('Ctrl Pts',(0.0823499098869818,0.222649799466091,
-0.32617672611718));
#82012=CARTESIAN_POINT('Ctrl Pts',(0.0727726864805359,0.225961537904021,
-0.325443107747218));
#82013=CARTESIAN_POINT('Ctrl Pts',(0.0607968002134912,0.229261882958715,
-0.324574569025959));
#82014=CARTESIAN_POINT('Ctrl Pts',(0.0585724281075908,0.229840234802622,
-0.324415282928699));
#82015=CARTESIAN_POINT('Ctrl Pts',(0.0552991464789388,0.230640701026333,
-0.324184197217415));
#82016=CARTESIAN_POINT('Ctrl Pts',(0.0542566538772727,0.230888163821148,
-0.324111089074754));
#82017=CARTESIAN_POINT('Ctrl Pts',(0.0524804574162301,0.231297095740523,
-0.323987399813118));
#82018=CARTESIAN_POINT('Ctrl Pts',(0.0517476178585353,0.2314621546013,-0.323936620189704));
#82019=CARTESIAN_POINT('Ctrl Pts',(0.0500706866346547,0.231831490350322,
-0.323821007403158));
#82020=CARTESIAN_POINT('Ctrl Pts',(0.04912611799872,0.232033485064156,-0.32375630336873));
#82021=CARTESIAN_POINT('Ctrl Pts',(0.0464973582687399,0.232578869581847,
-0.323577321928129));
#82022=CARTESIAN_POINT('Ctrl Pts',(0.0448105898301258,0.232909738657296,
-0.323463718725321));
#82023=CARTESIAN_POINT('Ctrl Pts',(0.032177102441422,0.2352455361084,-0.322621104706866));
#82024=CARTESIAN_POINT('Ctrl Pts',(0.021103542522077,0.236496371368418,
-0.321928350421202));
#82025=CARTESIAN_POINT('Ctrl Pts',(0.0010892911798639,0.237339442916482,
-0.320694626488137));
#82026=CARTESIAN_POINT('Ctrl Pts',(-0.00781722545426386,0.237213172340247,
-0.320152075868688));
#82027=CARTESIAN_POINT('Ctrl Pts',(-0.024473012866557,0.236037798100911,
-0.319121716253824));
#82028=CARTESIAN_POINT('Ctrl Pts',(-0.0322181478482891,0.235105822802945,
-0.318636142384706));
#82029=CARTESIAN_POINT('Ctrl Pts',(-0.0405811005292778,0.233678471844009,
-0.318096673108255));
#82030=CARTESIAN_POINT('Ctrl Pts',(-0.0412587354183974,0.233559779549431,
-0.318052853219164));
#82031=CARTESIAN_POINT('Ctrl Pts',(-0.0419358257618152,0.233438144146741,
-0.318008956663326));
#82032=CARTESIAN_POINT('Origin',(0.,0.,-1.7456589891905));
#82033=CARTESIAN_POINT('',(-0.0419358257146564,0.233438144155213,-0.198327653695922));
#82034=CARTESIAN_POINT('',(-0.0419358573824119,0.23343813846628,-0.21792431326882));
#82035=CARTESIAN_POINT('',(-0.0419358257166344,0.233438144154858,-1.7456589891905));
#82036=CARTESIAN_POINT('',(-0.237174957655792,0.000141724990824578,-0.276089073795202));
#82037=CARTESIAN_POINT('Ctrl Pts',(-0.0419358257146564,0.233438144155213,
-0.198327653695922));
#82038=CARTESIAN_POINT('Ctrl Pts',(-0.0409295018561971,0.233618924473252,
-0.198398144126953));
#82039=CARTESIAN_POINT('Ctrl Pts',(-0.0399219914476528,0.233793200733438,
-0.198468316308305));
#82040=CARTESIAN_POINT('Ctrl Pts',(-0.0379917462161784,0.23411424712948,
-0.198601948924105));
#82041=CARTESIAN_POINT('Ctrl Pts',(-0.0370692168767604,0.234262089816906,
-0.198665464692559));
#82042=CARTESIAN_POINT('Ctrl Pts',(-0.0353118932121755,0.234533073978755,
-0.19878575615995));
#82043=CARTESIAN_POINT('Ctrl Pts',(-0.034477289734947,0.234657216180683,
-0.198842582756937));
#82044=CARTESIAN_POINT('Ctrl Pts',(-0.0324705827651871,0.234944764444413,
-0.198978518044225));
#82045=CARTESIAN_POINT('Ctrl Pts',(-0.0312978674836229,0.235103859437134,
-0.199057389664625));
#82046=CARTESIAN_POINT('Ctrl Pts',(-0.0271889308576364,0.235630003235974,
-0.199331905422777));
#82047=CARTESIAN_POINT('Ctrl Pts',(-0.0242469412288661,0.235950893558866,
-0.199525188091554));
#82048=CARTESIAN_POINT('Ctrl Pts',(-0.0168220143442844,0.236620396099102,
-0.200006512303282));
#82049=CARTESIAN_POINT('Ctrl Pts',(-0.0123336234078155,0.236896767771464,
-0.200291556632799));
#82050=CARTESIAN_POINT('Ctrl Pts',(0.0113721108625147,0.23768079081269,
-0.201778359613328));
#82051=CARTESIAN_POINT('Ctrl Pts',(0.0305901720537581,0.235978359998802,
-0.20292502075045));
#82052=CARTESIAN_POINT('Ctrl Pts',(0.0560615728204603,0.230554918206611,
-0.20456330421721));
#82053=CARTESIAN_POINT('Ctrl Pts',(0.0626655378895886,0.22884817563284,
-0.2049985933393));
#82054=CARTESIAN_POINT('Ctrl Pts',(0.0714532723348395,0.226168139172614,
-0.205597320091774));
#82055=CARTESIAN_POINT('Ctrl Pts',(0.073709589115798,0.225442882151697,
-0.20575280414045));
#82056=CARTESIAN_POINT('Ctrl Pts',(0.0774361015453184,0.224183131596434,
-0.206012719189443));
#82057=CARTESIAN_POINT('Ctrl Pts',(0.0789125884266836,0.223667676485543,
-0.206116522411113));
#82058=CARTESIAN_POINT('Ctrl Pts',(0.0818097755059774,0.222623984373176,
-0.206321883865032));
#82059=CARTESIAN_POINT('Ctrl Pts',(0.0832307245350489,0.222096654851263,
-0.206423407875292));
#82060=CARTESIAN_POINT('Ctrl Pts',(0.0866307240737717,0.220797667863252,
-0.206668314559968));
#82061=CARTESIAN_POINT('Ctrl Pts',(0.0886046224538898,0.220012983383521,
-0.206812126083803));
#82062=CARTESIAN_POINT('Ctrl Pts',(0.0955806457836407,0.217130699638356,
-0.207326343025699));
#82063=CARTESIAN_POINT('Ctrl Pts',(0.100520721818551,0.214888289170165,
-0.207701546929794));
#82064=CARTESIAN_POINT('Ctrl Pts',(0.112847654321066,0.208774719773076,
-0.208666807060047));
#82065=CARTESIAN_POINT('Ctrl Pts',(0.120114872362343,0.204679922594302,
-0.209263525395607));
#82066=CARTESIAN_POINT('Ctrl Pts',(0.142733935714427,0.190314940920863,
-0.211204424988388));
#82067=CARTESIAN_POINT('Ctrl Pts',(0.157108495119061,0.178632917160131,
-0.212574485897301));
#82068=CARTESIAN_POINT('Ctrl Pts',(0.17150327087572,0.163839435516765,-0.214015687243499));
#82069=CARTESIAN_POINT('Ctrl Pts',(0.173001946396445,0.162256155304988,
-0.214166618343512));
#82070=CARTESIAN_POINT('Ctrl Pts',(0.175189386874293,0.15988045645427,-0.214387948933597));
#82071=CARTESIAN_POINT('Ctrl Pts',(0.175895016843176,0.159103817629245,
-0.214459510329381));
#82072=CARTESIAN_POINT('Ctrl Pts',(0.177149349376817,0.15770471479123,-0.214586973506717));
#82073=CARTESIAN_POINT('Ctrl Pts',(0.177699963334139,0.157084028926035,
-0.214643012607144));
#82074=CARTESIAN_POINT('Ctrl Pts',(0.178920151978048,0.155693930677102,
-0.214767393848887));
#82075=CARTESIAN_POINT('Ctrl Pts',(0.179588031563946,0.154923077198476,
-0.214835613669686));
#82076=CARTESIAN_POINT('Ctrl Pts',(0.181569456349057,0.152606123050205,
-0.215038507143711));
#82077=CARTESIAN_POINT('Ctrl Pts',(0.182868197495589,0.151047407424668,
-0.215172166210084));
#82078=CARTESIAN_POINT('Ctrl Pts',(0.191983046944001,0.139818087640798,
-0.21611666488759));
#82079=CARTESIAN_POINT('Ctrl Pts',(0.19904901951974,0.129561401520513,-0.21688396384605));
#82080=CARTESIAN_POINT('Ctrl Pts',(0.214123429576822,0.103513068382687,
-0.218731839225787));
#82081=CARTESIAN_POINT('Ctrl Pts',(0.221232787789981,0.087291327449634,
-0.219806414719049));
#82082=CARTESIAN_POINT('Ctrl Pts',(0.227371487580681,0.0675520607829406,
-0.22113993249783));
#82083=CARTESIAN_POINT('Ctrl Pts',(0.228211958917473,0.0646558178095527,
-0.2213360583988));
#82084=CARTESIAN_POINT('Ctrl Pts',(0.229485439364699,0.059932750458057,
-0.221657077139612));
#82085=CARTESIAN_POINT('Ctrl Pts',(0.229952396058286,0.0581153737704889,
-0.221780881259894));
#82086=CARTESIAN_POINT('Ctrl Pts',(0.230748790532733,0.054855847936956,
-0.222003520359543));
#82087=CARTESIAN_POINT('Ctrl Pts',(0.231086396188675,0.0534157814926653,
-0.222102087881052));
#82088=CARTESIAN_POINT('Ctrl Pts',(0.231775697230703,0.0503466400727279,
-0.222312639924505));
#82089=CARTESIAN_POINT('Ctrl Pts',(0.232123733810521,0.0487168343575298,
-0.222424735411401));
#82090=CARTESIAN_POINT('Ctrl Pts',(0.233021104798295,0.0442864535046422,
-0.222730290557363));
#82091=CARTESIAN_POINT('Ctrl Pts',(0.233537097698428,0.0414794890363676,
-0.222924791395834));
#82092=CARTESIAN_POINT('Ctrl Pts',(0.236644508588403,0.0226728140927505,
-0.224234542005628));
#82093=CARTESIAN_POINT('Ctrl Pts',(0.23764010807973,0.00645582023651468,
-0.225400098459223));
#82094=CARTESIAN_POINT('Ctrl Pts',(0.23638211304355,-0.0241735396929289,
-0.227635834337646));
#82095=CARTESIAN_POINT('Ctrl Pts',(0.234470267849405,-0.038530825471946,
-0.228696964040031));
#82096=CARTESIAN_POINT('Ctrl Pts',(0.2307718722995,-0.0547833980533723,
-0.229861202801916));
#82097=CARTESIAN_POINT('Ctrl Pts',(0.230250654967697,-0.0569342999416245,
-0.230014468222843));
#82098=CARTESIAN_POINT('Ctrl Pts',(0.2294364166732,-0.0601001321103912,
-0.230238542524708));
#82099=CARTESIAN_POINT('Ctrl Pts',(0.22916661759314,-0.0611208365723519,
-0.23031055314345));
#82100=CARTESIAN_POINT('Ctrl Pts',(0.22867254113044,-0.0629407537955865,
-0.230438488454017));
#82101=CARTESIAN_POINT('Ctrl Pts',(0.228450874581588,-0.0637406269324779,
-0.230494555054434));
#82102=CARTESIAN_POINT('Ctrl Pts',(0.227948962014029,-0.0655154972710364,
-0.23061860220317));
#82103=CARTESIAN_POINT('Ctrl Pts',(0.227666655946991,-0.0664898753987113,
-0.230686464540052));
#82104=CARTESIAN_POINT('Ctrl Pts',(0.226808868083418,-0.069380998084145,
-0.230887197120308));
#82105=CARTESIAN_POINT('Ctrl Pts',(0.226215352852066,-0.0712923580666077,
-0.231019084582089));
#82106=CARTESIAN_POINT('Ctrl Pts',(0.224778952662249,-0.0757194897754526,
-0.231323150652912));
#82107=CARTESIAN_POINT('Ctrl Pts',(0.223917895770443,-0.0782291242891998,
-0.231494445886704));
#82108=CARTESIAN_POINT('Ctrl Pts',(0.220717668370193,-0.0870703521247797,
-0.232095836284813));
#82109=CARTESIAN_POINT('Ctrl Pts',(0.218150436507448,-0.0933163167867047,
-0.232516944114112));
#82110=CARTESIAN_POINT('Ctrl Pts',(0.208700143588238,-0.11377833226479,
-0.233909753533043));
#82111=CARTESIAN_POINT('Ctrl Pts',(0.200665771464921,-0.127414675726643,
-0.234862761617255));
#82112=CARTESIAN_POINT('Ctrl Pts',(0.187341707435098,-0.145604802054904,
-0.236281685003211));
#82113=CARTESIAN_POINT('Ctrl Pts',(0.183116299598353,-0.150884332270434,
-0.236713344727211));
#82114=CARTESIAN_POINT('Ctrl Pts',(0.177116914925679,-0.157756670092081,
-0.237307901715248));
#82115=CARTESIAN_POINT('Ctrl Pts',(0.175535849385921,-0.159514054029838,
-0.237462996884774));
#82116=CARTESIAN_POINT('Ctrl Pts',(0.172866359926882,-0.162393486435211,
-0.237722448513469));
#82117=CARTESIAN_POINT('Ctrl Pts',(0.171792615037167,-0.163528957838641,
-0.237826182215525));
#82118=CARTESIAN_POINT('Ctrl Pts',(0.16965479235176,-0.165745384617747,
-0.238031549997146));
#82119=CARTESIAN_POINT('Ctrl Pts',(0.1685914099205,-0.16682690852156,-0.238133151193444));
#82120=CARTESIAN_POINT('Ctrl Pts',(0.166010401503156,-0.169402069418534,
-0.238378490683021));
#82121=CARTESIAN_POINT('Ctrl Pts',(0.164482914501138,-0.170885589954701,
-0.238522661425185));
#82122=CARTESIAN_POINT('Ctrl Pts',(0.158968707943325,-0.176098644612035,
-0.239039660542118));
#82123=CARTESIAN_POINT('Ctrl Pts',(0.1548737179677,-0.179710616909112,-0.239417355775723));
#82124=CARTESIAN_POINT('Ctrl Pts',(0.144157279857009,-0.188524550826298,
-0.240390960346584));
#82125=CARTESIAN_POINT('Ctrl Pts',(0.137377103152433,-0.193520890712681,
-0.240993682564937));
#82126=CARTESIAN_POINT('Ctrl Pts',(0.115081230103722,-0.20818778225116,
-0.242927398593638));
#82127=CARTESIAN_POINT('Ctrl Pts',(0.0987066923786381,-0.216432154076649,
-0.244282923447387));
#82128=CARTESIAN_POINT('Ctrl Pts',(0.0794644365894028,-0.223477751461063,
-0.245714329730063));
#82129=CARTESIAN_POINT('Ctrl Pts',(0.0773705599006154,-0.224211282997807,
-0.245867983877223));
#82130=CARTESIAN_POINT('Ctrl Pts',(0.0742645410349022,-0.22525069402127,
-0.246092507625092));
#82131=CARTESIAN_POINT('Ctrl Pts',(0.0732602205408174,-0.225579337275491,
-0.246164585931202));
#82132=CARTESIAN_POINT('Ctrl Pts',(0.0714631790824603,-0.226154114571549,
-0.246292587290453));
#82133=CARTESIAN_POINT('Ctrl Pts',(0.0706713268466481,-0.226402811660227,
-0.246348652998078));
#82134=CARTESIAN_POINT('Ctrl Pts',(0.0689097245733172,-0.226945935125436,
-0.246472632548486));
#82135=CARTESIAN_POINT('Ctrl Pts',(0.067939378164787,-0.227238307949446,
-0.246540428871454));
#82136=CARTESIAN_POINT('Ctrl Pts',(0.0650521016142871,-0.2280881186778,
-0.246740771526688));
#82137=CARTESIAN_POINT('Ctrl Pts',(0.0631299201846156,-0.228627600319104,
-0.246872340681428));
#82138=CARTESIAN_POINT('Ctrl Pts',(0.0586462310286548,-0.229825135888949,
-0.247175547936488));
#82139=CARTESIAN_POINT('Ctrl Pts',(0.0560800355443542,-0.230464757272304,
-0.247346309527518));
#82140=CARTESIAN_POINT('Ctrl Pts',(0.0469618253401709,-0.232576130648339,
-0.247945011676506));
#82141=CARTESIAN_POINT('Ctrl Pts',(0.0403582345617251,-0.233812520889941,
-0.248364049529611));
#82142=CARTESIAN_POINT('Ctrl Pts',(0.0182028173772347,-0.236993860421164,
-0.249747412432378));
#82143=CARTESIAN_POINT('Ctrl Pts',(0.00251303484284274,-0.237678587525126,
-0.250693120635765));
#82144=CARTESIAN_POINT('Ctrl Pts',(-0.0200199974816856,-0.236429277364393,
-0.252112193814768));
#82145=CARTESIAN_POINT('Ctrl Pts',(-0.0268898286998592,-0.23574674345327,
-0.252552598600587));
#82146=CARTESIAN_POINT('Ctrl Pts',(-0.0360743234931796,-0.234427563424361,
-0.253157222044048));
#82147=CARTESIAN_POINT('Ctrl Pts',(-0.0384236640166671,-0.234053969590932,
-0.253313273930226));
#82148=CARTESIAN_POINT('Ctrl Pts',(-0.0423094383433683,-0.233375971025366,
-0.253573888222162));
#82149=CARTESIAN_POINT('Ctrl Pts',(-0.0438492212495575,-0.233091565745727,
-0.253677815895445));
#82150=CARTESIAN_POINT('Ctrl Pts',(-0.0468727081328813,-0.232502094693021,
-0.253883232867947));
#82151=CARTESIAN_POINT('Ctrl Pts',(-0.048356530564873,-0.232198020173935,
-0.253984686155312));
#82152=CARTESIAN_POINT('Ctrl Pts',(-0.0519079600649834,-0.231434720732135,
-0.254229098546829));
#82153=CARTESIAN_POINT('Ctrl Pts',(-0.0539724958372374,-0.230961978399432,
-0.254372481922059));
#82154=CARTESIAN_POINT('Ctrl Pts',(-0.0612581645060652,-0.229190669965657,
-0.254883240960526));
#82155=CARTESIAN_POINT('Ctrl Pts',(-0.0664408052724592,-0.227742260616885,
-0.255255328663669));
#82156=CARTESIAN_POINT('Ctrl Pts',(-0.0794212189962251,-0.223633803746686,
-0.256210163212567));
#82157=CARTESIAN_POINT('Ctrl Pts',(-0.087137563490602,-0.220741546854758,
-0.256799383868919));
#82158=CARTESIAN_POINT('Ctrl Pts',(-0.110726080089186,-0.210470269257686,
-0.258662201734215));
#82159=CARTESIAN_POINT('Ctrl Pts',(-0.12594301130912,-0.201733443822673,
-0.259958703337694));
#82160=CARTESIAN_POINT('Ctrl Pts',(-0.142397655557306,-0.189692573614097,
-0.261393974947682));
#82161=CARTESIAN_POINT('Ctrl Pts',(-0.144703008694772,-0.187939899750234,
-0.261595776834146));
#82162=CARTESIAN_POINT('Ctrl Pts',(-0.147923341950101,-0.185397203533312,
-0.261878049370054));
#82163=CARTESIAN_POINT('Ctrl Pts',(-0.148865174718396,-0.184641810227938,
-0.261960650594842));
#82164=CARTESIAN_POINT('Ctrl Pts',(-0.150458507916976,-0.183343766660157,
-0.262100411187563));
#82165=CARTESIAN_POINT('Ctrl Pts',(-0.151112933831447,-0.182804761154152,
-0.262157820056457));
#82166=CARTESIAN_POINT('Ctrl Pts',(-0.152430692339048,-0.181707501843111,
-0.262273410618339));
#82167=CARTESIAN_POINT('Ctrl Pts',(-0.153093870381759,-0.181149107380981,
-0.262331582198368));
#82168=CARTESIAN_POINT('Ctrl Pts',(-0.154799170583816,-0.179697194516189,
-0.262481208074137));
#82169=CARTESIAN_POINT('Ctrl Pts',(-0.155836641508467,-0.178798227939612,
-0.26257227953416));
#82170=CARTESIAN_POINT('Ctrl Pts',(-0.158166006212268,-0.176744159684211,
-0.262777008956114));
#82171=CARTESIAN_POINT('Ctrl Pts',(-0.159453176054601,-0.175583793505985,
-0.262890318573197));
#82172=CARTESIAN_POINT('Ctrl Pts',(-0.163325162380227,-0.172015551546312,
-0.263232142502596));
#82173=CARTESIAN_POINT('Ctrl Pts',(-0.165869105982434,-0.169563855076502,
-0.263458070893069));
#82174=CARTESIAN_POINT('Ctrl Pts',(-0.176142383352577,-0.159210550523479,
-0.264380904150731));
#82175=CARTESIAN_POINT('Ctrl Pts',(-0.183369911272575,-0.150829862892916,
-0.265055985185981));
#82176=CARTESIAN_POINT('Ctrl Pts',(-0.198724041381375,-0.130283418644556,
-0.266629107176469));
#82177=CARTESIAN_POINT('Ctrl Pts',(-0.20636227527214,-0.117811541647545,
-0.267527285381611));
#82178=CARTESIAN_POINT('Ctrl Pts',(-0.21418755505127,-0.101909122793188,
-0.268669301252688));
#82179=CARTESIAN_POINT('Ctrl Pts',(-0.215513764223123,-0.0990736797484941,
-0.268872694215964));
#82180=CARTESIAN_POINT('Ctrl Pts',(-0.217557964764391,-0.0944677621900607,
-0.269203206296615));
#82181=CARTESIAN_POINT('Ctrl Pts',(-0.218311382219074,-0.0927133548378095,
-0.269329125099819));
#82182=CARTESIAN_POINT('Ctrl Pts',(-0.21961205622331,-0.0895808210678317,
-0.269554099520366));
#82183=CARTESIAN_POINT('Ctrl Pts',(-0.220167731420872,-0.088206284427222,
-0.26965286519967));
#82184=CARTESIAN_POINT('Ctrl Pts',(-0.221313563593816,-0.0852936170948401,
-0.269862298268792));
#82185=CARTESIAN_POINT('Ctrl Pts',(-0.221900652202324,-0.0837543722016801,
-0.269973062139128));
#82186=CARTESIAN_POINT('Ctrl Pts',(-0.22342971788904,-0.0796164668709136,
-0.270271117734031));
#82187=CARTESIAN_POINT('Ctrl Pts',(-0.224342356768258,-0.0770073144024099,
-0.270459365215664));
#82188=CARTESIAN_POINT('Ctrl Pts',(-0.229585288078088,-0.0611332879802501,
-0.271606971425387));
#82189=CARTESIAN_POINT('Ctrl Pts',(-0.232782897997094,-0.0475256227456584,
-0.272602837934513));
#82190=CARTESIAN_POINT('Ctrl Pts',(-0.236376712548598,-0.0225032534968295,
-0.274440149136895));
#82191=CARTESIAN_POINT('Ctrl Pts',(-0.237181727633546,-0.0111877461047197,
-0.275272490505346));
#82192=CARTESIAN_POINT('Ctrl Pts',(-0.237174957655792,0.000141724990824578,
-0.276089073795202));
#82193=CARTESIAN_POINT('Ctrl Pts',(-0.237174957457087,0.000142057132016532,
-0.276089097734616));
#82194=CARTESIAN_POINT('Ctrl Pts',(-0.237171123206076,0.00654362463918838,
-0.276550497106281));
#82195=CARTESIAN_POINT('Ctrl Pts',(-0.236908112528632,0.012943138279542,
-0.277006175155684));
#82196=CARTESIAN_POINT('Ctrl Pts',(-0.236286385740191,0.0205482695635013,
-0.277535497651701));
#82197=CARTESIAN_POINT('Ctrl Pts',(-0.236176867875511,0.021770960076209,
-0.27762021817767));
#82198=CARTESIAN_POINT('Ctrl Pts',(-0.235973345262132,0.0238604473347336,
-0.27776428851774));
#82199=CARTESIAN_POINT('Ctrl Pts',(-0.235884046417673,0.0247276631767218,
-0.277823873369331));
#82200=CARTESIAN_POINT('Ctrl Pts',(-0.235706331929214,0.0263648697496518,
-0.277935941863676));
#82201=CARTESIAN_POINT('Ctrl Pts',(-0.235618919917507,0.027134957061119,
-0.277988478882682));
#82202=CARTESIAN_POINT('Ctrl Pts',(-0.23543630164553,0.0286763387713665,
-0.278093263611178));
#82203=CARTESIAN_POINT('Ctrl Pts',(-0.235341076468838,0.029447619740959,
-0.278145509817826));
#82204=CARTESIAN_POINT('Ctrl Pts',(-0.235078125829394,0.0314946170376426,
-0.278283710842499));
#82205=CARTESIAN_POINT('Ctrl Pts',(-0.234903804536596,0.0327694819225507,
-0.278369305355628));
#82206=CARTESIAN_POINT('Ctrl Pts',(-0.234228363170439,0.0374265174654742,
-0.278680442328267));
#82207=CARTESIAN_POINT('Ctrl Pts',(-0.23366447574511,0.0407993380059595,
-0.278902811857691));
#82208=CARTESIAN_POINT('Ctrl Pts',(-0.23150980970564,0.0521695515704485,
-0.279645968361694));
#82209=CARTESIAN_POINT('Ctrl Pts',(-0.229579620685065,0.0600972033888468,
-0.280153297476245));
#82210=CARTESIAN_POINT('Ctrl Pts',(-0.222417162287063,0.0840645845238832,
-0.281695453450788));
#82211=CARTESIAN_POINT('Ctrl Pts',(-0.215881182356292,0.0996570917218917,
-0.282714097051292));
#82212=CARTESIAN_POINT('Ctrl Pts',(-0.205148301362771,0.119143517555824,
-0.284126770614526));
#82213=CARTESIAN_POINT('Ctrl Pts',(-0.202389371298119,0.123772124403427,
-0.284473340961328));
#82214=CARTESIAN_POINT('Ctrl Pts',(-0.198329116547582,0.130084712040769,
-0.284964076005512));
#82215=CARTESIAN_POINT('Ctrl Pts',(-0.197159019835836,0.131851398154596,
-0.285103460646346));
#82216=CARTESIAN_POINT('Ctrl Pts',(-0.195112106652395,0.134853777393515,
-0.285344007064877));
#82217=CARTESIAN_POINT('Ctrl Pts',(-0.194246819411867,0.136097202054448,
-0.285444732111356));
#82218=CARTESIAN_POINT('Ctrl Pts',(-0.192463183464042,0.138608638349725,
-0.285650481024354));
#82219=CARTESIAN_POINT('Ctrl Pts',(-0.191544073393037,0.139876014238715,
-0.285755530668955));
#82220=CARTESIAN_POINT('Ctrl Pts',(-0.189197759539961,0.143044890688382,
-0.286021339884536));
#82221=CARTESIAN_POINT('Ctrl Pts',(-0.187754413618233,0.144934165810404,
-0.286182720369332));
#82222=CARTESIAN_POINT('Ctrl Pts',(-0.182019556237,0.152211388141673,-0.286815998338447));
#82223=CARTESIAN_POINT('Ctrl Pts',(-0.177522917977595,0.157432597239822,
-0.287295909786507));
#82224=CARTESIAN_POINT('Ctrl Pts',(-0.162066449515711,0.173874349211572,
-0.288894211410407));
#82225=CARTESIAN_POINT('Ctrl Pts',(-0.150221505017259,0.184204298527142,
-0.290044704432539));
#82226=CARTESIAN_POINT('Ctrl Pts',(-0.131971006368453,0.197182064023182,
-0.291674537374458));
#82227=CARTESIAN_POINT('Ctrl Pts',(-0.126332738989519,0.200841139320602,
-0.292160449990694));
#82228=CARTESIAN_POINT('Ctrl Pts',(-0.118268344683921,0.205600526103471,
-0.292824831013015));
#82229=CARTESIAN_POINT('Ctrl Pts',(-0.11596785407051,0.206906828706353,
-0.293011025212574));
#82230=CARTESIAN_POINT('Ctrl Pts',(-0.111893289307474,0.209131201553266,
-0.293334420813143));
#82231=CARTESIAN_POINT('Ctrl Pts',(-0.110128601965627,0.210065845247152,
-0.293472428184499));
#82232=CARTESIAN_POINT('Ctrl Pts',(-0.107450690220867,0.211441143085923,
-0.29367854597882));
#82233=CARTESIAN_POINT('Ctrl Pts',(-0.106546150592695,0.211898385334806,
-0.293747606371846));
#82234=CARTESIAN_POINT('Ctrl Pts',(-0.104895559291557,0.212719512911488,
-0.293872571110933));
#82235=CARTESIAN_POINT('Ctrl Pts',(-0.104150509410119,0.213085290360015,
-0.293928586546284));
#82236=CARTESIAN_POINT('Ctrl Pts',(-0.102452612427634,0.213907828887981,
-0.294055361508047));
#82237=CARTESIAN_POINT('Ctrl Pts',(-0.101498617774442,0.214362141594273,
-0.294125972225777));
#82238=CARTESIAN_POINT('Ctrl Pts',(-0.0985327658483198,0.215750305011249,
-0.29434367445231));
#82239=CARTESIAN_POINT('Ctrl Pts',(-0.0965107564119194,0.216662352108946,
-0.294489519747987));
#82240=CARTESIAN_POINT('Ctrl Pts',(-0.0813113264516549,0.223263182334507,
-0.295568894712545));
#82241=CARTESIAN_POINT('Ctrl Pts',(-0.0676528558566008,0.22777441008224,
-0.296445644416075));
#82242=CARTESIAN_POINT('Ctrl Pts',(-0.0497766623182696,0.23192720841488,
-0.297571054174985));
#82243=CARTESIAN_POINT('Ctrl Pts',(-0.0458644337506357,0.232732392654763,
-0.297815947261534));
#82244=CARTESIAN_POINT('Ctrl Pts',(-0.041935800711444,0.233438148646895,
-0.298061760785893));
#82245=CARTESIAN_POINT('Ctrl Pts',(-0.0419358257618152,0.233438144146741,
-0.318008956663326));
#82246=CARTESIAN_POINT('Ctrl Pts',(-0.044737224506651,0.232934888905049,
-0.317827338718805));
#82247=CARTESIAN_POINT('Ctrl Pts',(-0.0475293014180542,0.232381253280233,
-0.31764440450371));
#82248=CARTESIAN_POINT('Ctrl Pts',(-0.0531300061965072,0.231165538094296,
-0.317273042601415));
#82249=CARTESIAN_POINT('Ctrl Pts',(-0.0559377967065655,0.230502202348022,
-0.317084609932621));
#82250=CARTESIAN_POINT('Ctrl Pts',(-0.0603533376871241,0.229373610792194,
-0.316784349244478));
#82251=CARTESIAN_POINT('Ctrl Pts',(-0.061969518210354,0.228942257501103,
-0.316673608092285));
#82252=CARTESIAN_POINT('Ctrl Pts',(-0.065004402940657,0.228097766931276,
-0.316464006431609));
#82253=CARTESIAN_POINT('Ctrl Pts',(-0.0664240784855643,0.227688395199332,
-0.316365272057344));
#82254=CARTESIAN_POINT('Ctrl Pts',(-0.0696266824510545,0.226732404246507,
-0.31614093994205));
#82255=CARTESIAN_POINT('Ctrl Pts',(-0.0714071569589592,0.226177973363719,
-0.316015093125072));
#82256=CARTESIAN_POINT('Ctrl Pts',(-0.0768381431734285,0.224416272751221,
-0.315627653325478));
#82257=CARTESIAN_POINT('Ctrl Pts',(-0.0804658345185623,0.223141233765613,
-0.315363872686392));
#82258=CARTESIAN_POINT('Ctrl Pts',(-0.101606714570959,0.215128206394684,
-0.313796252903389));
#82259=CARTESIAN_POINT('Ctrl Pts',(-0.118298783878005,0.206420020816826,
-0.312426568457534));
#82260=CARTESIAN_POINT('Ctrl Pts',(-0.142140668815194,0.190132472464896,
-0.310321402256422));
#82261=CARTESIAN_POINT('Ctrl Pts',(-0.150121291795257,0.183896612738681,
-0.309588208050902));
#82262=CARTESIAN_POINT('Ctrl Pts',(-0.159396122117666,0.17564206652246,
-0.308720108761738));
#82263=CARTESIAN_POINT('Ctrl Pts',(-0.161090171560196,0.174089680564432,
-0.308560862914296));
#82264=CARTESIAN_POINT('Ctrl Pts',(-0.163540709299311,0.171777660790436,
-0.308329824110731));
#82265=CARTESIAN_POINT('Ctrl Pts',(-0.164314976743271,0.171037179800256,
-0.308256723350301));
#82266=CARTESIAN_POINT('Ctrl Pts',(-0.1656235622732,0.16976860872937,-0.308133042336726));
#82267=CARTESIAN_POINT('Ctrl Pts',(-0.166160422846664,0.169243194331276,
-0.308082263650794));
#82268=CARTESIAN_POINT('Ctrl Pts',(-0.167381944514523,0.168036300736565,
-0.307966647150124));
#82269=CARTESIAN_POINT('Ctrl Pts',(-0.168064948531303,0.167353180048676,
-0.307901938518283));
#82270=CARTESIAN_POINT('Ctrl Pts',(-0.169951821676863,0.165442782567326,
-0.307722931605015));
#82271=CARTESIAN_POINT('Ctrl Pts',(-0.171146577587408,0.164206532743473,
-0.307609307835896));
#82272=CARTESIAN_POINT('Ctrl Pts',(-0.179999188518044,0.154844873753818,
-0.306764280778705));
#82273=CARTESIAN_POINT('Ctrl Pts',(-0.187089178391121,0.146199684170916,
-0.306069376668011));
#82274=CARTESIAN_POINT('Ctrl Pts',(-0.194093647528112,0.136310454038169,
-0.305323084695238));
#82275=CARTESIAN_POINT('Ctrl Pts',(-0.194638311143868,0.135531589448686,
-0.305264618339877));
#82276=CARTESIAN_POINT('Ctrl Pts',(-0.199832467761139,0.128008097442224,
-0.304702643742296));
#82277=CARTESIAN_POINT('Ctrl Pts',(-0.204134223151693,0.121030185759319,
-0.304202629271089));
#82278=CARTESIAN_POINT('Ctrl Pts',(-0.211726254429488,0.107154623293612,
-0.303225921147974));
#82279=CARTESIAN_POINT('Ctrl Pts',(-0.215061272561181,0.100293350834665,
-0.302750604068203));
#82280=CARTESIAN_POINT('Ctrl Pts',(-0.219430434859827,0.090080003930204,
-0.30204385172456));
#82281=CARTESIAN_POINT('Ctrl Pts',(-0.220730131667224,0.0868465887399211,
-0.301820244975571));
#82282=CARTESIAN_POINT('Ctrl Pts',(-0.222963637299589,0.080915624169825,
-0.301409453376225));
#82283=CARTESIAN_POINT('Ctrl Pts',(-0.223920891601717,0.078227584397045,
-0.301223043338473));
#82284=CARTESIAN_POINT('Ctrl Pts',(-0.225359900312026,0.0739437058484087,
-0.300925265407773));
#82285=CARTESIAN_POINT('Ctrl Pts',(-0.225873744756608,0.0723588798611643,
-0.300814953344303));
#82286=CARTESIAN_POINT('Ctrl Pts',(-0.22681201159711,0.0693576104274131,
-0.300605705159269));
#82287=CARTESIAN_POINT('Ctrl Pts',(-0.227239969496744,0.0679423492532866,
-0.300506890159107));
#82288=CARTESIAN_POINT('Ctrl Pts',(-0.228180704954914,0.0647229793272365,
-0.300281741536621));
#82289=CARTESIAN_POINT('Ctrl Pts',(-0.228685365605001,0.0629166223994482,
-0.300155151586595));
#82290=CARTESIAN_POINT('Ctrl Pts',(-0.229944988481716,0.0581924880857962,
-0.299823321492983));
#82291=CARTESIAN_POINT('Ctrl Pts',(-0.230665831395072,0.0552660490577273,
-0.299617008753984));
#82292=CARTESIAN_POINT('Ctrl Pts',(-0.235230687917048,0.0350853430291806,
-0.298188580713162));
#82293=CARTESIAN_POINT('Ctrl Pts',(-0.237190255440108,0.017464876297323,
-0.296906754664287));
#82294=CARTESIAN_POINT('Ctrl Pts',(-0.237164491901432,-0.0122038927658462,
-0.294741033499129));
#82295=CARTESIAN_POINT('Ctrl Pts',(-0.236243679131832,-0.02418489130466,
-0.293866282665382));
#82296=CARTESIAN_POINT('Ctrl Pts',(-0.234070332528061,-0.0383190626295442,
-0.292866418383835));
#82297=CARTESIAN_POINT('Ctrl Pts',(-0.233687694842236,-0.040587355012341,
-0.292706990211092));
#82298=CARTESIAN_POINT('Ctrl Pts',(-0.233078462852458,-0.0439039807099018,
-0.292475739015903));
#82299=CARTESIAN_POINT('Ctrl Pts',(-0.232877676313772,-0.0449568387911039,
-0.2924026049039));
#82300=CARTESIAN_POINT('Ctrl Pts',(-0.232508644788786,-0.0468230765778575,
-0.292273505401584));
#82301=CARTESIAN_POINT('Ctrl Pts',(-0.232343256747318,-0.0476369763435173,
-0.29221738637369));
#82302=CARTESIAN_POINT('Ctrl Pts',(-0.231969239368831,-0.0494292756284665,
-0.292094214046769));
#82303=CARTESIAN_POINT('Ctrl Pts',(-0.231758692633005,-0.0504072393866343,
-0.292027268710623));
#82304=CARTESIAN_POINT('Ctrl Pts',(-0.231123292757905,-0.0532704287460914,
-0.291831966983464));
#82305=CARTESIAN_POINT('Ctrl Pts',(-0.230681567704826,-0.055151880680277,
-0.291704515881314));
#82306=CARTESIAN_POINT('Ctrl Pts',(-0.229607414813284,-0.0594881542306176,
-0.29141237831822));
#82307=CARTESIAN_POINT('Ctrl Pts',(-0.228958522904757,-0.061938690007187,
-0.291248481805874));
#82308=CARTESIAN_POINT('Ctrl Pts',(-0.226566109956297,-0.070421608189004,
-0.290683806939825));
#82309=CARTESIAN_POINT('Ctrl Pts',(-0.224622351775801,-0.0763951232515684,
-0.290290886308136));
#82310=CARTESIAN_POINT('Ctrl Pts',(-0.214932176059995,-0.102590943123617,
-0.288560987456185));
#82311=CARTESIAN_POINT('Ctrl Pts',(-0.204676490544675,-0.121771291991963,
-0.287265233888708));
#82312=CARTESIAN_POINT('Ctrl Pts',(-0.190255229946048,-0.141645209744189,
-0.285679416188456));
#82313=CARTESIAN_POINT('Ctrl Pts',(-0.188506295092459,-0.14396455639597,
-0.285490333663751));
#82314=CARTESIAN_POINT('Ctrl Pts',(-0.185578386823007,-0.147702546010807,
-0.285178563053428));
#82315=CARTESIAN_POINT('Ctrl Pts',(-0.184424650583428,-0.149140630585426,
-0.285056860638317));
#82316=CARTESIAN_POINT('Ctrl Pts',(-0.18231747702811,-0.151705292892896,
-0.284836536656718));
#82317=CARTESIAN_POINT('Ctrl Pts',(-0.181370059009402,-0.152836709753627,
-0.284738160605091));
#82318=CARTESIAN_POINT('Ctrl Pts',(-0.179317206485874,-0.155242279451977,
-0.284526407489484));
#82319=CARTESIAN_POINT('Ctrl Pts',(-0.178208618999928,-0.156513621550609,
-0.284412904149812));
#82320=CARTESIAN_POINT('Ctrl Pts',(-0.175123201405693,-0.159976736714004,
-0.28409923632388));
#82321=CARTESIAN_POINT('Ctrl Pts',(-0.173118929309267,-0.162143537988935,
-0.283897933977972));
#82322=CARTESIAN_POINT('Ctrl Pts',(-0.160083332301166,-0.175718940144487,
-0.282603459960778));
#82323=CARTESIAN_POINT('Ctrl Pts',(-0.14797273206907,-0.186031502910855,
-0.281462496582422));
#82324=CARTESIAN_POINT('Ctrl Pts',(-0.122878564582116,-0.203389830309261,
-0.279237459876383));
#82325=CARTESIAN_POINT('Ctrl Pts',(-0.110084202406319,-0.210589889922625,
-0.278161402006479));
#82326=CARTESIAN_POINT('Ctrl Pts',(-0.0947049310682703,-0.217457493067885,
-0.276985231664967));
#82327=CARTESIAN_POINT('Ctrl Pts',(-0.0926910865022384,-0.218323495290598,
-0.276833449300373));
#82328=CARTESIAN_POINT('Ctrl Pts',(-0.089693808526222,-0.219563446341538,
-0.276611127888372));
#82329=CARTESIAN_POINT('Ctrl Pts',(-0.0887194933516494,-0.219958945856709,
-0.276539412422915));
#82330=CARTESIAN_POINT('Ctrl Pts',(-0.0869718292039139,-0.220654865709612,
-0.276411802896522));
#82331=CARTESIAN_POINT('Ctrl Pts',(-0.086199501251897,-0.220957721933588,
-0.276355769800023));
#82332=CARTESIAN_POINT('Ctrl Pts',(-0.0844764353274816,-0.221622985324765,
-0.276231559155315));
#82333=CARTESIAN_POINT('Ctrl Pts',(-0.0835249399719161,-0.221983333266375,
-0.276163502216342));
#82334=CARTESIAN_POINT('Ctrl Pts',(-0.0806801648442189,-0.223039818330449,
-0.275961529198533));
#82335=CARTESIAN_POINT('Ctrl Pts',(-0.0787802369266001,-0.223717957466329,
-0.275828614448493));
#82336=CARTESIAN_POINT('Ctrl Pts',(-0.065550073507352,-0.228250731312771,
-0.274915176004379));
#82337=CARTESIAN_POINT('Ctrl Pts',(-0.0539494389249483,-0.231267681349453,
-0.27417497891087));
#82338=CARTESIAN_POINT('Ctrl Pts',(-0.0242180253288097,-0.236639463413832,
-0.272318726146063));
#82339=CARTESIAN_POINT('Ctrl Pts',(-0.00595455369689349,-0.23780078972795,
-0.271210896862154));
#82340=CARTESIAN_POINT('Ctrl Pts',(0.0152194618640961,-0.236704721490966,
-0.269842414849665));
#82341=CARTESIAN_POINT('Ctrl Pts',(0.018174788174134,-0.236496158582522,
-0.269649658192206));
#82342=CARTESIAN_POINT('Ctrl Pts',(0.0229785367224207,-0.236066578130393,
-0.269333073140798));
#82343=CARTESIAN_POINT('Ctrl Pts',(0.024829682379341,-0.235879055884054,
-0.269210283762994));
#82344=CARTESIAN_POINT('Ctrl Pts',(0.028146143825838,-0.235503624450238,
-0.268988785116284));
#82345=CARTESIAN_POINT('Ctrl Pts',(0.0296122870441792,-0.235323765966861,
-0.268890332864579));
#82346=CARTESIAN_POINT('Ctrl Pts',(0.0327376114709803,-0.234910698954546,
-0.26867928436136));
#82347=CARTESIAN_POINT('Ctrl Pts',(0.0343961853875026,-0.234673581532916,
-0.268566570155466));
#82348=CARTESIAN_POINT('Ctrl Pts',(0.0389160629527017,-0.233978454397253,
-0.268257389180577));
#82349=CARTESIAN_POINT('Ctrl Pts',(0.0417716257831052,-0.233485560724004,
-0.268059838120755));
#82350=CARTESIAN_POINT('Ctrl Pts',(0.0598124875004766,-0.23003002077837,
-0.266797127522385));
#82351=CARTESIAN_POINT('Ctrl Pts',(0.0746836961509353,-0.225640268093727,
-0.265686620470406));
#82352=CARTESIAN_POINT('Ctrl Pts',(0.10309832759062,-0.214134163914343,
-0.263452353107394));
#82353=CARTESIAN_POINT('Ctrl Pts',(0.116598202778023,-0.20709329908703,
-0.26233492838413));
#82354=CARTESIAN_POINT('Ctrl Pts',(0.131145348479145,-0.197629842440134,
-0.261123466124225));
#82355=CARTESIAN_POINT('Ctrl Pts',(0.132941909799233,-0.19642582948905,
-0.260973763481388));
#82356=CARTESIAN_POINT('Ctrl Pts',(0.135582579598143,-0.194603285051045,
-0.260753879875164));
#82357=CARTESIAN_POINT('Ctrl Pts',(0.136439412404792,-0.194003508447241,
-0.260682558006626));
#82358=CARTESIAN_POINT('Ctrl Pts',(0.137968610652286,-0.192917938673726,
-0.26055535453712));
#82359=CARTESIAN_POINT('Ctrl Pts',(0.138642422930922,-0.192434267246748,
-0.260499337976279));
#82360=CARTESIAN_POINT('Ctrl Pts',(0.14014125784733,-0.191346424169191,
-0.260374806708731));
#82361=CARTESIAN_POINT('Ctrl Pts',(0.140964923683091,-0.190740442961656,
-0.260306416362147));
#82362=CARTESIAN_POINT('Ctrl Pts',(0.143422351635631,-0.188907869606034,
-0.260102419339643));
#82363=CARTESIAN_POINT('Ctrl Pts',(0.145044259696085,-0.187665440516178,
-0.259967844062063));
#82364=CARTESIAN_POINT('Ctrl Pts',(0.157534261770296,-0.177839060107151,
-0.258930226621931));
#82365=CARTESIAN_POINT('Ctrl Pts',(0.167649169349661,-0.168337861946153,
-0.258081321272123));
#82366=CARTESIAN_POINT('Ctrl Pts',(0.187580879846075,-0.146025671495544,
-0.256246405739105));
#82367=CARTESIAN_POINT('Ctrl Pts',(0.197037607658726,-0.132989440744198,
-0.255263098502526));
#82368=CARTESIAN_POINT('Ctrl Pts',(0.206660021572981,-0.1164182971209,-0.254027992627695));
#82369=CARTESIAN_POINT('Ctrl Pts',(0.208163459012305,-0.113708211380189,
-0.253826571581315));
#82370=CARTESIAN_POINT('Ctrl Pts',(0.210502338947981,-0.109290239056547,
-0.253498653809637));
#82371=CARTESIAN_POINT('Ctrl Pts',(0.211371129998348,-0.10760035366967,
-0.253373326877886));
#82372=CARTESIAN_POINT('Ctrl Pts',(0.212880850105106,-0.104574940189114,
-0.253149037770916));
#82373=CARTESIAN_POINT('Ctrl Pts',(0.213529755160749,-0.103243488647643,
-0.253050359481818));
#82374=CARTESIAN_POINT('Ctrl Pts',(0.214875783557254,-0.100414670961389,
-0.252840722074069));
#82375=CARTESIAN_POINT('Ctrl Pts',(0.215569818697656,-0.0989159316360683,
-0.252729662886937));
#82376=CARTESIAN_POINT('Ctrl Pts',(0.217392135345646,-0.0948704314916453,
-0.252429843993907));
#82377=CARTESIAN_POINT('Ctrl Pts',(0.218491268708121,-0.0923109074411124,
-0.252240108221553));
#82378=CARTESIAN_POINT('Ctrl Pts',(0.225184781710279,-0.0759341871235249,
-0.251025340990785));
#82379=CARTESIAN_POINT('Ctrl Pts',(0.229510133731044,-0.061637165720413,
-0.249958226679802));
#82380=CARTESIAN_POINT('Ctrl Pts',(0.235656506295156,-0.0312570795072213,
-0.247701568476758));
#82381=CARTESIAN_POINT('Ctrl Pts',(0.23723424670619,-0.0151979632950478,
-0.246514887085686));
#82382=CARTESIAN_POINT('Ctrl Pts',(0.237165430903666,0.00297621288797808,
-0.245247490743187));
#82383=CARTESIAN_POINT('Ctrl Pts',(0.237130247962653,0.00505427478992429,
-0.245103740710931));
#82384=CARTESIAN_POINT('Ctrl Pts',(0.237036797149612,0.00816071496787572,
-0.244890854639971));
#82385=CARTESIAN_POINT('Ctrl Pts',(0.236999140809376,0.00918954987237131,
-0.244820676720547));
#82386=CARTESIAN_POINT('Ctrl Pts',(0.236919055571126,0.0110466977904574,
-0.244694631186582));
#82387=CARTESIAN_POINT('Ctrl Pts',(0.236878980505837,0.0118750609268024,
-0.244638640548759));
#82388=CARTESIAN_POINT('Ctrl Pts',(0.236778933743643,0.0137402962778775,
-0.244513080280148));
#82389=CARTESIAN_POINT('Ctrl Pts',(0.236716496140876,0.0147770011340075,
-0.244443646627491));
#82390=CARTESIAN_POINT('Ctrl Pts',(0.236505596892895,0.0179331272526227,
-0.244233248820455));
#82391=CARTESIAN_POINT('Ctrl Pts',(0.23633546116401,0.0200510592879945,
-0.244093413980158));
#82392=CARTESIAN_POINT('Ctrl Pts',(0.235341043720841,0.0306444569417719,
-0.243399493207613));
#82393=CARTESIAN_POINT('Ctrl Pts',(0.23408912166504,0.0390743318283394,
-0.242864849516497));
#82394=CARTESIAN_POINT('Ctrl Pts',(0.228060541885727,0.068618348108636,
-0.24099737152617));
#82395=CARTESIAN_POINT('Ctrl Pts',(0.220855101704296,0.089123979595825,
-0.239702457676735));
#82396=CARTESIAN_POINT('Ctrl Pts',(0.209641029013294,0.110955286301882,
-0.238117460143258));
#82397=CARTESIAN_POINT('Ctrl Pts',(0.208264951189478,0.113517159623033,
-0.237928173712019));
#82398=CARTESIAN_POINT('Ctrl Pts',(0.205939567314313,0.117661709463617,
-0.237616135206286));
#82399=CARTESIAN_POINT('Ctrl Pts',(0.205018252915175,0.119259795870082,
-0.237494371711622));
#82400=CARTESIAN_POINT('Ctrl Pts',(0.203326458989841,0.12211678694886,-0.237273981226376));
#82401=CARTESIAN_POINT('Ctrl Pts',(0.202562684228262,0.123379566258158,
-0.237175600386978));
#82402=CARTESIAN_POINT('Ctrl Pts',(0.200901116304354,0.126069683966955,
-0.236963885770057));
#82403=CARTESIAN_POINT('Ctrl Pts',(0.199999791057501,0.127494733501093,
-0.23685042618563));
#82404=CARTESIAN_POINT('Ctrl Pts',(0.197480812258102,0.131384941425137,
-0.236537010710989));
#82405=CARTESIAN_POINT('Ctrl Pts',(0.195832311531961,0.133829662049031,
-0.236335920028601));
#82406=CARTESIAN_POINT('Ctrl Pts',(0.1850717872156,0.149162821672237,-0.235047572658002));
#82407=CARTESIAN_POINT('Ctrl Pts',(0.17473940732281,0.161143060871856,-0.233913077632657));
#82408=CARTESIAN_POINT('Ctrl Pts',(0.15259804829544,0.182163169599489,-0.231686982579052));
#82409=CARTESIAN_POINT('Ctrl Pts',(0.140974861054286,0.191300136693265,
-0.23060308542215));
#82410=CARTESIAN_POINT('Ctrl Pts',(0.12674175486475,0.200482616674133,-0.229420379300678));
#82411=CARTESIAN_POINT('Ctrl Pts',(0.124889887881046,0.201641436129321,
-0.229269133627125));
#82412=CARTESIAN_POINT('Ctrl Pts',(0.122124451376495,0.203319211082609,
-0.229047440720122));
#82413=CARTESIAN_POINT('Ctrl Pts',(0.12122307888493,0.203857912454156,-0.228975826285862));
#82414=CARTESIAN_POINT('Ctrl Pts',(0.11960326456342,0.204811444662896,-0.228848321537439));
#82415=CARTESIAN_POINT('Ctrl Pts',(0.11888619397236,0.205228510941119,-0.228792293228712));
#82416=CARTESIAN_POINT('Ctrl Pts',(0.11728365425391,0.206149370156308,-0.2286680026274));
#82417=CARTESIAN_POINT('Ctrl Pts',(0.116397114079517,0.206651228645653,
-0.228599861891554));
#82418=CARTESIAN_POINT('Ctrl Pts',(0.113739891180856,0.208132921448531,
-0.228397378344447));
#82419=CARTESIAN_POINT('Ctrl Pts',(0.111959821231756,0.209095851071455,
-0.228264044434999));
#82420=CARTESIAN_POINT('Ctrl Pts',(0.0995565237143344,0.215601601108312,
-0.227349329052414));
#82421=CARTESIAN_POINT('Ctrl Pts',(0.0885375182843082,0.22035592507667,
-0.226608334829467));
#82422=CARTESIAN_POINT('Ctrl Pts',(0.0599853404440585,0.230185583827689,
-0.224753132956455));
#82423=CARTESIAN_POINT('Ctrl Pts',(0.0421420985265483,0.234110254978682,
-0.223647029432988));
#82424=CARTESIAN_POINT('Ctrl Pts',(0.0210759898834814,0.236255322603898,
-0.222280354114845));
#82425=CARTESIAN_POINT('Ctrl Pts',(0.0181204824398082,0.23650036294834,
-0.222087408859593));
#82426=CARTESIAN_POINT('Ctrl Pts',(0.0133036130396962,0.236808909277324,
-0.221770577768577));
#82427=CARTESIAN_POINT('Ctrl Pts',(0.0114446761111455,0.236906025024711,
-0.221647733749127));
#82428=CARTESIAN_POINT('Ctrl Pts',(0.00810885019312719,0.237040944266894,
-0.221426177069523));
#82429=CARTESIAN_POINT('Ctrl Pts',(0.0066323724036509,0.23708684944135,
-0.221327722020929));
#82430=CARTESIAN_POINT('Ctrl Pts',(0.00348115318510966,0.237155365240182,
-0.221116711741436));
#82431=CARTESIAN_POINT('Ctrl Pts',(0.00180641587100689,0.2371740337858,
-0.221004038979407));
#82432=CARTESIAN_POINT('Ctrl Pts',(-0.00276325770148828,0.237176570449328,
-0.220695088179958));
#82433=CARTESIAN_POINT('Ctrl Pts',(-0.00565784294585478,0.237125175148811,
-0.220497728528713));
#82434=CARTESIAN_POINT('Ctrl Pts',(-0.0197582379176476,0.236616495735213,
-0.219527834492675));
#82435=CARTESIAN_POINT('Ctrl Pts',(-0.0309145038583286,0.235418063051798,
-0.218733292196062));
#82436=CARTESIAN_POINT('Ctrl Pts',(-0.0419358573824117,0.23343813846628,
-0.21792431326882));
#82437=CARTESIAN_POINT('Origin',(0.,0.,-1.7456589891905));
#82438=CARTESIAN_POINT('',(-0.0419357865133591,0.233438151197498,-0.0979694843087456));
#82439=CARTESIAN_POINT('',(-0.0419358257166351,0.233438144154857,-0.117607078812657));
#82440=CARTESIAN_POINT('',(-0.0419358257166344,0.233438144154858,-1.7456589891905));
#82441=CARTESIAN_POINT('Ctrl Pts',(-0.0419357865133626,0.233438151197497,
-0.0979694843087454));
#82442=CARTESIAN_POINT('Ctrl Pts',(-0.0296502970070915,0.235645166899533,
-0.0988623235472579));
#82443=CARTESIAN_POINT('Ctrl Pts',(-0.0172022719087811,0.236880230763759,
-0.0997773423278653));
#82444=CARTESIAN_POINT('Ctrl Pts',(0.00526639588502789,0.237326279997791,
-0.101416241531675));
#82445=CARTESIAN_POINT('Ctrl Pts',(0.0152438555841809,0.23689483305609,
-0.102139040137741));
#82446=CARTESIAN_POINT('Ctrl Pts',(0.0274385970011549,0.235593570823695,
-0.102996550783393));
#82447=CARTESIAN_POINT('Ctrl Pts',(0.0297083461511621,0.235318130091136,
-0.103155020639958));
#82448=CARTESIAN_POINT('Ctrl Pts',(0.0330342406462287,0.234865631355384,
-0.103385226295336));
#82449=CARTESIAN_POINT('Ctrl Pts',(0.0340936593597889,0.234714184381017,
-0.103458255688368));
#82450=CARTESIAN_POINT('Ctrl Pts',(0.0358939585432025,0.234444379689392,
-0.103581805818235));
#82451=CARTESIAN_POINT('Ctrl Pts',(0.0366353544226617,0.234329670118397,
-0.10363252559559));
#82452=CARTESIAN_POINT('Ctrl Pts',(0.0383259100939763,0.234059885739427,
-0.103747802115136));
#82453=CARTESIAN_POINT('Ctrl Pts',(0.0392746864652687,0.233902553602965,
-0.103812231261498));
#82454=CARTESIAN_POINT('Ctrl Pts',(0.041912373716246,0.233448653431822,
-0.103990674570355));
#82455=CARTESIAN_POINT('Ctrl Pts',(0.0435991041550788,0.233139527744794,
-0.104104011653244));
#82456=CARTESIAN_POINT('Ctrl Pts',(0.0563400609601184,0.23066138783625,
-0.104955287501612));
#82457=CARTESIAN_POINT('Ctrl Pts',(0.0672320017415795,0.227725281444977,
-0.105655775882896));
#82458=CARTESIAN_POINT('Ctrl Pts',(0.0790729838427031,0.223609150026908,
-0.106427197102565));
#82459=CARTESIAN_POINT('Ctrl Pts',(0.0802674417935084,0.223183168194255,
-0.106505123941752));
#82460=CARTESIAN_POINT('Ctrl Pts',(0.0935508502138204,0.218325448147053,
-0.107373494122607));
#82461=CARTESIAN_POINT('Ctrl Pts',(0.105262485500107,0.212926167066963,
-0.108156791943747));
#82462=CARTESIAN_POINT('Ctrl Pts',(0.122629804939815,0.203134901026933,
-0.109409586985152));
#82463=CARTESIAN_POINT('Ctrl Pts',(0.128623298879774,0.199393804944908,
-0.109860150855383));
#82464=CARTESIAN_POINT('Ctrl Pts',(0.136351794999779,0.19407614654249,-0.110471684636701));
#82465=CARTESIAN_POINT('Ctrl Pts',(0.13824355289158,0.192733188924514,-0.110623915464666));
#82466=CARTESIAN_POINT('Ctrl Pts',(0.141362616754455,0.190449419196269,
-0.110879365283801));
#82467=CARTESIAN_POINT('Ctrl Pts',(0.142600994878233,0.189523947707758,
-0.11098198798307));
#82468=CARTESIAN_POINT('Ctrl Pts',(0.145016645453251,0.187681590911978,
-0.111184596387472));
#82469=CARTESIAN_POINT('Ctrl Pts',(0.146194488975136,0.186765570281374,
-0.111284544872751));
#82470=CARTESIAN_POINT('Ctrl Pts',(0.149025636432859,0.184520567151784,
-0.111527662042611));
#82471=CARTESIAN_POINT('Ctrl Pts',(0.150669880487639,0.183180420948124,
-0.111671274290903));
#82472=CARTESIAN_POINT('Ctrl Pts',(0.156208400688382,0.178541211467236,
-0.112163487267368));
#82473=CARTESIAN_POINT('Ctrl Pts',(0.160013833270068,0.175138787437171,
-0.112516267672541));
#82474=CARTESIAN_POINT('Ctrl Pts',(0.17919013169737,0.156846364889147,-0.114372903367958));
#82475=CARTESIAN_POINT('Ctrl Pts',(0.192602417110062,0.140049669047372,
-0.115959227321972));
#82476=CARTESIAN_POINT('Ctrl Pts',(0.205961363579348,0.117700783204675,
-0.117838972832013));
#82477=CARTESIAN_POINT('Ctrl Pts',(0.208227142396897,0.113644269778579,
-0.118171408062634));
#82478=CARTESIAN_POINT('Ctrl Pts',(0.21176934589466,0.10684042088923,-0.118711904040006));
#82479=CARTESIAN_POINT('Ctrl Pts',(0.213114874962106,0.104130608332205,
-0.118922846291999));
#82480=CARTESIAN_POINT('Ctrl Pts',(0.214916077539252,0.100321837949637,
-0.119212636339154));
#82481=CARTESIAN_POINT('Ctrl Pts',(0.215415829334444,0.0992442047540888,
-0.119293892916657));
#82482=CARTESIAN_POINT('Ctrl Pts',(0.216255501052316,0.0973973611503321,
-0.11943184250332));
#82483=CARTESIAN_POINT('Ctrl Pts',(0.216599458075126,0.0966300292158377,
-0.119488774312477));
#82484=CARTESIAN_POINT('Ctrl Pts',(0.217314403298719,0.095012061626186,
-0.119607998972777));
#82485=CARTESIAN_POINT('Ctrl Pts',(0.217684487627134,0.0941610623125813,
-0.119670238888293));
#82486=CARTESIAN_POINT('Ctrl Pts',(0.21867442692235,0.0918476906086514,
-0.119838223970688));
#82487=CARTESIAN_POINT('Ctrl Pts',(0.219284615626328,0.0903811979696927,
-0.119943410308313));
#82488=CARTESIAN_POINT('Ctrl Pts',(0.222252324054333,0.0830417550943661,
-0.120463910861526));
#82489=CARTESIAN_POINT('Ctrl Pts',(0.224389071118317,0.0770817012009295,
-0.120867797357706));
#82490=CARTESIAN_POINT('Ctrl Pts',(0.230055927068213,0.0590316652519871,
-0.122055535693422));
#82491=CARTESIAN_POINT('Ctrl Pts',(0.232864730298824,0.0467388204712098,
-0.122819020413789));
#82492=CARTESIAN_POINT('Ctrl Pts',(0.23594012342884,0.0256847102230647,
-0.12412812249881));
#82493=CARTESIAN_POINT('Ctrl Pts',(0.23672244495599,0.0170268520257548,
-0.124666668127815));
#82494=CARTESIAN_POINT('Ctrl Pts',(0.237224436192984,0.00277035666120866,
-0.12557144375578));
#82495=CARTESIAN_POINT('Ctrl Pts',(0.237223951580282,-0.00281018967891917,
-0.125930037078752));
#82496=CARTESIAN_POINT('Ctrl Pts',(0.236950725223211,-0.0105335445401973,
-0.126435150991745));
#82497=CARTESIAN_POINT('Ctrl Pts',(0.236845522297355,-0.0126806866194454,
-0.126576515422812));
#82498=CARTESIAN_POINT('Ctrl Pts',(0.236615915622534,-0.0163465636875743,
-0.126819617219337));
#82499=CARTESIAN_POINT('Ctrl Pts',(0.236506033809207,-0.017866098022569,
-0.126920898222681));
#82500=CARTESIAN_POINT('Ctrl Pts',(0.23626870837976,-0.0207601382877996,
-0.127114818793256));
#82501=CARTESIAN_POINT('Ctrl Pts',(0.2361438890667,-0.0221348010830024,
-0.127207372442139));
#82502=CARTESIAN_POINT('Ctrl Pts',(0.235788703276618,-0.0257006251974836,
-0.12744863959502));
#82503=CARTESIAN_POINT('Ctrl Pts',(0.235539795532364,-0.0278897630292103,
-0.127597925128941));
#82504=CARTESIAN_POINT('Ctrl Pts',(0.234557521020033,-0.0355735508544045,
-0.128126176961274));
#82505=CARTESIAN_POINT('Ctrl Pts',(0.233662114391534,-0.0410452892270384,
-0.128510099895484));
#82506=CARTESIAN_POINT('Ctrl Pts',(0.228956189674062,-0.064592586781429,
-0.130196829830423));
#82507=CARTESIAN_POINT('Ctrl Pts',(0.223233293707215,-0.0822183391911368,
-0.13155519211993));
#82508=CARTESIAN_POINT('Ctrl Pts',(0.213052851899309,-0.104381792501776,
-0.133324915147205));
#82509=CARTESIAN_POINT('Ctrl Pts',(0.210379075050698,-0.109671007246825,
-0.133751626709029));
#82510=CARTESIAN_POINT('Ctrl Pts',(0.205773711537953,-0.11799158313073,
-0.134424555871511));
#82511=CARTESIAN_POINT('Ctrl Pts',(0.203966535122649,-0.121088768858699,
-0.134675413868254));
#82512=CARTESIAN_POINT('Ctrl Pts',(0.201421854732821,-0.125231166540058,
-0.135010272661717));
#82513=CARTESIAN_POINT('Ctrl Pts',(0.200745213416078,-0.126312976807091,
-0.135097660143353));
#82514=CARTESIAN_POINT('Ctrl Pts',(0.199596312420747,-0.128117280316379,
-0.135243236113761));
#82515=CARTESIAN_POINT('Ctrl Pts',(0.199128786446996,-0.128842741121642,
-0.135301720381014));
#82516=CARTESIAN_POINT('Ctrl Pts',(0.198163444429932,-0.130322857406912,
-0.135420919112081));
#82517=CARTESIAN_POINT('Ctrl Pts',(0.197665256220833,-0.131077246014573,
-0.135481608294959));
#82518=CARTESIAN_POINT('Ctrl Pts',(0.196342369979463,-0.133055750942652,
-0.135640657651683));
#82519=CARTESIAN_POINT('Ctrl Pts',(0.195510522389097,-0.134275072208138,
-0.135738557599815));
#82520=CARTESIAN_POINT('Ctrl Pts',(0.191822389533644,-0.139574186748402,
-0.136163876183264));
#82521=CARTESIAN_POINT('Ctrl Pts',(0.188849182762526,-0.143571504638587,
-0.136484323789983));
#82522=CARTESIAN_POINT('Ctrl Pts',(0.176295664600405,-0.159383547039957,
-0.13776353729087));
#82523=CARTESIAN_POINT('Ctrl Pts',(0.165714901945666,-0.170358201862381,
-0.138680749379591));
#82524=CARTESIAN_POINT('Ctrl Pts',(0.145037245659004,-0.188042895364414,
-0.140358765807748));
#82525=CARTESIAN_POINT('Ctrl Pts',(0.135341716696507,-0.19513712982678,
-0.141108930978769));
#82526=CARTESIAN_POINT('Ctrl Pts',(0.122863008083415,-0.202888942367795,
-0.142062787531925));
#82527=CARTESIAN_POINT('Ctrl Pts',(0.120550077429619,-0.204271680758161,
-0.142239068440764));
#82528=CARTESIAN_POINT('Ctrl Pts',(0.116798390582325,-0.206428640332843,
-0.142524466897245));
#82529=CARTESIAN_POINT('Ctrl Pts',(0.115374277767884,-0.207227950328199,
-0.1426326794694));
#82530=CARTESIAN_POINT('Ctrl Pts',(0.112637969237295,-0.208726805699705,
-0.14284042856344));
#82531=CARTESIAN_POINT('Ctrl Pts',(0.11132722252084,-0.209428844441946,
-0.142939870303248));
#82532=CARTESIAN_POINT('Ctrl Pts',(0.108320533248837,-0.211003031619845,
-0.143167854295474));
#82533=CARTESIAN_POINT('Ctrl Pts',(0.106620517609702,-0.211867133203949,
-0.143296671171745));
#82534=CARTESIAN_POINT('Ctrl Pts',(0.101155608140235,-0.21456246333258,
-0.143710594915352));
#82535=CARTESIAN_POINT('Ctrl Pts',(0.097352754746615,-0.216314458661817,
-0.143998386545142));
#82536=CARTESIAN_POINT('Ctrl Pts',(0.076587470532443,-0.225222653805274,
-0.145569461166284));
#82537=CARTESIAN_POINT('Ctrl Pts',(0.0588841223995243,-0.230484972980918,
-0.14691448185796));
#82538=CARTESIAN_POINT('Ctrl Pts',(0.0308961087109997,-0.235366855482296,
-0.148985768307353));
#82539=CARTESIAN_POINT('Ctrl Pts',(0.0209377253252353,-0.23646094135097,
-0.149710785513475));
#82540=CARTESIAN_POINT('Ctrl Pts',(0.00865477628305593,-0.237028067937734,
-0.150570420715818));
#82541=CARTESIAN_POINT('Ctrl Pts',(0.00636888330677741,-0.237100502804236,
-0.15072891438379));
#82542=CARTESIAN_POINT('Ctrl Pts',(0.0030129791589171,-0.237158272360684,
-0.150959080476967));
#82543=CARTESIAN_POINT('Ctrl Pts',(0.00194362205948525,-0.237169447097857,
-0.151032047743092));
#82544=CARTESIAN_POINT('Ctrl Pts',(0.000123397125888366,-0.237176156287328,
-0.151155570988071));
#82545=CARTESIAN_POINT('Ctrl Pts',(-0.000627420688090736,-0.237175358626607,
-0.151206324337761));
#82546=CARTESIAN_POINT('Ctrl Pts',(-0.00234487118603359,-0.237165378127367,
-0.151321959629161));
#82547=CARTESIAN_POINT('Ctrl Pts',(-0.00331146528490936,-0.237153851504941,
-0.151386711623283));
#82548=CARTESIAN_POINT('Ctrl Pts',(-0.00600141592165971,-0.237105324315642,
-0.15156606430459));
#82549=CARTESIAN_POINT('Ctrl Pts',(-0.00772452011704736,-0.237055445044221,
-0.151679985054861));
#82550=CARTESIAN_POINT('Ctrl Pts',(-0.0209506145951181,-0.23652821412298,
-0.152548034431701));
#82551=CARTESIAN_POINT('Ctrl Pts',(-0.0324072025590242,-0.235232583416807,
-0.153263286616282));
#82552=CARTESIAN_POINT('Ctrl Pts',(-0.0442734976490555,-0.233006756850052,
-0.154006167339822));
#82553=CARTESIAN_POINT('Ctrl Pts',(-0.0448209908590255,-0.232902061203127,
-0.154040446250534));
#82554=CARTESIAN_POINT('Ctrl Pts',(-0.0546570822746849,-0.230985164146947,
-0.154656425495733));
#82555=CARTESIAN_POINT('Ctrl Pts',(-0.0638292257565803,-0.228620579608439,
-0.155233379005194));
#82556=CARTESIAN_POINT('Ctrl Pts',(-0.0793861270860631,-0.223600542396664,
-0.156246223577628));
#82557=CARTESIAN_POINT('Ctrl Pts',(-0.0858412260355698,-0.221202697185943,
-0.156677095946507));
#82558=CARTESIAN_POINT('Ctrl Pts',(-0.0965617681928096,-0.216680398596723,
-0.157419157318497));
#82559=CARTESIAN_POINT('Ctrl Pts',(-0.100884160695088,-0.214702006151476,
-0.157725917847034));
#82560=CARTESIAN_POINT('Ctrl Pts',(-0.106955765509068,-0.211699150489251,
-0.158169391279693));
#82561=CARTESIAN_POINT('Ctrl Pts',(-0.108755968918634,-0.210779991697385,
-0.158302493265481));
#82562=CARTESIAN_POINT('Ctrl Pts',(-0.111868656451764,-0.209140205320798,
-0.158535580709895));
#82563=CARTESIAN_POINT('Ctrl Pts',(-0.113186490573348,-0.208429940158595,
-0.158635197973423));
#82564=CARTESIAN_POINT('Ctrl Pts',(-0.115725062858082,-0.20703056612243,
-0.158828953862965));
#82565=CARTESIAN_POINT('Ctrl Pts',(-0.116946592074119,-0.20634301524124,
-0.158923033795038));
#82566=CARTESIAN_POINT('Ctrl Pts',(-0.120193190949362,-0.204477543302115,
-0.159175395607942));
#82567=CARTESIAN_POINT('Ctrl Pts',(-0.122206978977638,-0.203280403556447,
-0.159334363762111));
#82568=CARTESIAN_POINT('Ctrl Pts',(-0.129809096186403,-0.198607372570047,
-0.159944025178804));
#82569=CARTESIAN_POINT('Ctrl Pts',(-0.135269166933451,-0.194929546079957,
-0.160401980760352));
#82570=CARTESIAN_POINT('Ctrl Pts',(-0.156276049181342,-0.179471677087928,
-0.162246144590844));
#82571=CARTESIAN_POINT('Ctrl Pts',(-0.170496885396524,-0.166020864733996,
-0.163690208444125));
#82572=CARTESIAN_POINT('Ctrl Pts',(-0.185783894244829,-0.147501610085427,
-0.165421610853591));
#82573=CARTESIAN_POINT('Ctrl Pts',(-0.188559241875037,-0.143936782942163,
-0.165744446181988));
#82574=CARTESIAN_POINT('Ctrl Pts',(-0.192987113327554,-0.137901291045558,
-0.166271461189346));
#82575=CARTESIAN_POINT('Ctrl Pts',(-0.19469800369272,-0.135475021090899,
-0.166478325900128));
#82576=CARTESIAN_POINT('Ctrl Pts',(-0.19702713335062,-0.132036705832587,
-0.166763888942078));
#82577=CARTESIAN_POINT('Ctrl Pts',(-0.197683947227924,-0.131051288128644,
-0.166844878600389));
#82578=CARTESIAN_POINT('Ctrl Pts',(-0.198795915797674,-0.129355618169833,
-0.166982734377129));
#82579=CARTESIAN_POINT('Ctrl Pts',(-0.199254706253551,-0.128647791348568,
-0.167039834035365));
#82580=CARTESIAN_POINT('Ctrl Pts',(-0.200213320589415,-0.127151399690861,
-0.167159593043341));
#82581=CARTESIAN_POINT('Ctrl Pts',(-0.200712276150341,-0.12636231424909,
-0.167222197294596));
#82582=CARTESIAN_POINT('Ctrl Pts',(-0.202061497451522,-0.124200400006544,
-0.167392288613574));
#82583=CARTESIAN_POINT('Ctrl Pts',(-0.202902441524335,-0.122821772055035,
-0.167499192470464));
#82584=CARTESIAN_POINT('Ctrl Pts',(-0.207170059161103,-0.115662045762974,
-0.168046956485997));
#82585=CARTESIAN_POINT('Ctrl Pts',(-0.210364301721418,-0.109745253559405,
-0.168474892278541));
#82586=CARTESIAN_POINT('Ctrl Pts',(-0.219580861595622,-0.090787515397533,
-0.169795237678399));
#82587=CARTESIAN_POINT('Ctrl Pts',(-0.224673269829578,-0.0773310182121016,
-0.170661704553817));
#82588=CARTESIAN_POINT('Ctrl Pts',(-0.231347718129668,-0.0533101887918559,
-0.172203453400025));
#82589=CARTESIAN_POINT('Ctrl Pts',(-0.233493482912646,-0.0429476118216739,
-0.172866752055428));
#82590=CARTESIAN_POINT('Ctrl Pts',(-0.235331768237854,-0.029649432772079,
-0.173736915432756));
#82591=CARTESIAN_POINT('Ctrl Pts',(-0.23567157363426,-0.0268148885641986,
-0.173923419753141));
#82592=CARTESIAN_POINT('Ctrl Pts',(-0.236128644959213,-0.0223164269138676,
-0.17422136407572));
#82593=CARTESIAN_POINT('Ctrl Pts',(-0.236279670300917,-0.0206561623852188,
-0.174331747677524));
#82594=CARTESIAN_POINT('Ctrl Pts',(-0.236531678892094,-0.0175195586972447,
-0.174541143305403));
#82595=CARTESIAN_POINT('Ctrl Pts',(-0.236636373061018,-0.0160435915765055,
-0.174640034194312));
#82596=CARTESIAN_POINT('Ctrl Pts',(-0.236842542188051,-0.0126930992496076,
-0.174865374608882));
#82597=CARTESIAN_POINT('Ctrl Pts',(-0.236935584727386,-0.0108181743880108,
-0.174992080937197));
#82598=CARTESIAN_POINT('Ctrl Pts',(-0.237120120327206,-0.00592729861421873,
-0.175324266635088));
#82599=CARTESIAN_POINT('Ctrl Pts',(-0.237176331506308,-0.00291043915855068,
-0.175530820825717));
#82600=CARTESIAN_POINT('Ctrl Pts',(-0.237169629823592,0.0120064184497657,
-0.176560669106382));
#82601=CARTESIAN_POINT('Ctrl Pts',(-0.236268727446282,0.0238872698427732,
-0.177409033635695));
#82602=CARTESIAN_POINT('Ctrl Pts',(-0.232595665367843,0.0480468528614814,
-0.179181181641774));
#82603=CARTESIAN_POINT('Ctrl Pts',(-0.22973046826708,0.0602756598030736,
-0.180103840466648));
#82604=CARTESIAN_POINT('Ctrl Pts',(-0.223972964181899,0.0782856049083706,
-0.181465462863492));
#82605=CARTESIAN_POINT('Ctrl Pts',(-0.221790416919298,0.0842707001371504,
-0.181918159224013));
#82606=CARTESIAN_POINT('Ctrl Pts',(-0.218764640787951,0.0916326550916187,
-0.182469493903072));
#82607=CARTESIAN_POINT('Ctrl Pts',(-0.218145061551391,0.093098034363224,
-0.182578952955352));
#82608=CARTESIAN_POINT('Ctrl Pts',(-0.217140509370585,0.0954088166548229,
-0.182750987278822));
#82609=CARTESIAN_POINT('Ctrl Pts',(-0.21676524798063,0.0962583526113689,
-0.182814109999193));
#82610=CARTESIAN_POINT('Ctrl Pts',(-0.216038396768121,0.0978780281791985,
-0.182934188207076));
#82611=CARTESIAN_POINT('Ctrl Pts',(-0.215687663061853,0.0986485139394347,
-0.182991189472202));
#82612=CARTESIAN_POINT('Ctrl Pts',(-0.214830378888533,0.100505351189763,
-0.183128300551818));
#82613=CARTESIAN_POINT('Ctrl Pts',(-0.214319696103869,0.101589789470971,
-0.183208162754854));
#82614=CARTESIAN_POINT('Ctrl Pts',(-0.212477328474379,0.105426337412689,
-0.183490102194614));
#82615=CARTESIAN_POINT('Ctrl Pts',(-0.211100614825139,0.108156646974326,
-0.183689646358448));
#82616=CARTESIAN_POINT('Ctrl Pts',(-0.20747130783064,0.115020834465941,
-0.184190429503946));
#82617=CARTESIAN_POINT('Ctrl Pts',(-0.205147679212546,0.11911578843044,
-0.184488354641332));
#82618=CARTESIAN_POINT('Ctrl Pts',(-0.190996797101151,0.142410049123834,
-0.186193920512833));
#82619=CARTESIAN_POINT('Ctrl Pts',(-0.176602377519959,0.159912672971394,
-0.187531056512033));
#82620=CARTESIAN_POINT('Ctrl Pts',(-0.156885554463896,0.177921778831899,
-0.189241229014651));
#82621=CARTESIAN_POINT('Ctrl Pts',(-0.153745479005323,0.180642079648262,
-0.189510140310479));
#82622=CARTESIAN_POINT('Ctrl Pts',(-0.149044783077938,0.184502996840263,
-0.189908856633506));
#82623=CARTESIAN_POINT('Ctrl Pts',(-0.147538978764656,0.18570932283121,
-0.190036022723369));
#82624=CARTESIAN_POINT('Ctrl Pts',(-0.144844910826985,0.187814139659975,
-0.190262662666932));
#82625=CARTESIAN_POINT('Ctrl Pts',(-0.143662571948544,0.188720069142855,
-0.190361835606296));
#82626=CARTESIAN_POINT('Ctrl Pts',(-0.141175845133713,0.190588533401589,
-0.190569859540911));
#82627=CARTESIAN_POINT('Ctrl Pts',(-0.139869969087599,0.191548948927301,
-0.190678786045187));
#82628=CARTESIAN_POINT('Ctrl Pts',(-0.136411550309813,0.194038244058697,
-0.190966501124822));
#82629=CARTESIAN_POINT('Ctrl Pts',(-0.134243196607195,0.195544660889043,
-0.191146132365549));
#82630=CARTESIAN_POINT('Ctrl Pts',(-0.12297638748398,0.203096310757125,
-0.192075994484177));
#82631=CARTESIAN_POINT('Ctrl Pts',(-0.113494563711403,0.208543103336196,
-0.192847885563617));
#82632=CARTESIAN_POINT('Ctrl Pts',(-0.0907806086982198,0.219582141372441,
-0.194668225909773));
#82633=CARTESIAN_POINT('Ctrl Pts',(-0.077348037838596,0.224665734697365,
-0.195724955588978));
#82634=CARTESIAN_POINT('Ctrl Pts',(-0.0569941024071704,0.230325426267022,
-0.197249209986626));
#82635=CARTESIAN_POINT('Ctrl Pts',(-0.0503732679658347,0.231863497808429,
-0.197733162821848));
#82636=CARTESIAN_POINT('Ctrl Pts',(-0.0431089756126745,0.233225110688087,
-0.19824534105726));
#82637=CARTESIAN_POINT('Ctrl Pts',(-0.0425226023732719,0.233332733088914,
-0.198286551480927));
#82638=CARTESIAN_POINT('Ctrl Pts',(-0.0419358257146564,0.233438144155213,
-0.198327653695922));
#82639=CARTESIAN_POINT('',(-0.237174999736212,0.000149622570500169,-0.195497187201803));
#82640=CARTESIAN_POINT('Ctrl Pts',(-0.0419358573824119,0.23343813846628,
-0.21792431326882));
#82641=CARTESIAN_POINT('Ctrl Pts',(-0.0475813473021413,0.232423957742928,
-0.217509928377795));
#82642=CARTESIAN_POINT('Ctrl Pts',(-0.0531914539463961,0.231204729662501,
-0.217091959100834));
#82643=CARTESIAN_POINT('Ctrl Pts',(-0.0718995017673666,0.226421103070235,
-0.21568278922388));
#82644=CARTESIAN_POINT('Ctrl Pts',(-0.08473246436092,0.221938116056266,
-0.214689093391387));
#82645=CARTESIAN_POINT('Ctrl Pts',(-0.0989682866032168,0.215549057935862,
-0.213598669945546));
#82646=CARTESIAN_POINT('Ctrl Pts',(-0.100813330008522,0.214692317737573,
-0.21345762059194));
#82647=CARTESIAN_POINT('Ctrl Pts',(-0.103578434075613,0.21336484175236,
-0.213246895731129));
#82648=CARTESIAN_POINT('Ctrl Pts',(-0.104506763191787,0.212911681800699,
-0.213176262852819));
#82649=CARTESIAN_POINT('Ctrl Pts',(-0.106187000873629,0.212077843371299,
-0.213048666863625));
#82650=CARTESIAN_POINT('Ctrl Pts',(-0.10693989715422,0.211699195298644,
-0.212991583686003));
#82651=CARTESIAN_POINT('Ctrl Pts',(-0.10850471271827,0.210901736530197,
-0.212873154268009));
#82652=CARTESIAN_POINT('Ctrl Pts',(-0.109316253104794,0.210482236854643,
-0.212811851042991));
#82653=CARTESIAN_POINT('Ctrl Pts',(-0.111475115727062,0.209350428110302,
-0.21264902875134));
#82654=CARTESIAN_POINT('Ctrl Pts',(-0.112818056847528,0.208629790598616,
-0.21254801217778));
#82655=CARTESIAN_POINT('Ctrl Pts',(-0.119562607976484,0.20492641666531,
-0.212041568395363));
#82656=CARTESIAN_POINT('Ctrl Pts',(-0.124853786587566,0.201746375086211,
-0.211647122413952));
#82657=CARTESIAN_POINT('Ctrl Pts',(-0.139575678231878,0.192097048014007,
-0.210540364956864));
#82658=CARTESIAN_POINT('Ctrl Pts',(-0.148670991652626,0.185147538116201,
-0.209844614970619));
#82659=CARTESIAN_POINT('Ctrl Pts',(-0.167970311510928,0.168058769231198,
-0.208261922196304));
#82660=CARTESIAN_POINT('Ctrl Pts',(-0.177824246589785,0.157595170912801,
-0.207373553800128));
#82661=CARTESIAN_POINT('Ctrl Pts',(-0.1883891081727,0.14411548477092,-0.206262633302431));
#82662=CARTESIAN_POINT('Ctrl Pts',(-0.190067462902371,0.141894635264199,
-0.206080674187128));
#82663=CARTESIAN_POINT('Ctrl Pts',(-0.192678509028361,0.13831015640968,
-0.205788360392234));
#82664=CARTESIAN_POINT('Ctrl Pts',(-0.193636744596031,0.136965390218447,
-0.205678994601114));
#82665=CARTESIAN_POINT('Ctrl Pts',(-0.195427773767813,0.134395535352883,
-0.205470497454414));
#82666=CARTESIAN_POINT('Ctrl Pts',(-0.196263287427143,0.133172431531167,
-0.205371475979964));
#82667=CARTESIAN_POINT('Ctrl Pts',(-0.198144701979407,0.130362075661904,
-0.205144385638657));
#82668=CARTESIAN_POINT('Ctrl Pts',(-0.199183076085089,0.128769932552469,
-0.205016043318625));
#82669=CARTESIAN_POINT('Ctrl Pts',(-0.202368897983294,0.123754355414727,
-0.204612599241643));
#82670=CARTESIAN_POINT('Ctrl Pts',(-0.20444796145925,0.120288565313191,
-0.204335038133216));
#82671=CARTESIAN_POINT('Ctrl Pts',(-0.217230163614773,0.0976912409873149,
-0.202532016808482));
#82672=CARTESIAN_POINT('Ctrl Pts',(-0.225324127245524,0.0772088528636334,
-0.200913870670797));
#82673=CARTESIAN_POINT('Ctrl Pts',(-0.232174844739072,0.0489682894189661,
-0.198810257691918));
#82674=CARTESIAN_POINT('Ctrl Pts',(-0.233544999494523,0.0419500199357592,
-0.198298686662149));
#82675=CARTESIAN_POINT('Ctrl Pts',(-0.23488572077168,0.0329325829767082,
-0.197663620432129));
#82676=CARTESIAN_POINT('Ctrl Pts',(-0.235151015032261,0.030981568729426,
-0.197527537215044));
#82677=CARTESIAN_POINT('Ctrl Pts',(-0.235516870281126,0.028014737500568,
-0.19732282445107));
#82678=CARTESIAN_POINT('Ctrl Pts',(-0.23563521377347,0.0270012561039096,
-0.197253286522257));
#82679=CARTESIAN_POINT('Ctrl Pts',(-0.235830586734086,0.0252288869015158,
-0.197132401553093));
#82680=CARTESIAN_POINT('Ctrl Pts',(-0.235910499416103,0.0244703633485507,
-0.197080899613214));
#82681=CARTESIAN_POINT('Ctrl Pts',(-0.236066270194763,0.0229200630103421,
-0.196976111803439));
#82682=CARTESIAN_POINT('Ctrl Pts',(-0.236141805411595,0.0221282849541749,
-0.196922843244826));
#82683=CARTESIAN_POINT('Ctrl Pts',(-0.236304116651473,0.0203313289297527,
-0.196802483779544));
#82684=CARTESIAN_POINT('Ctrl Pts',(-0.236388465503058,0.0193259397540431,
-0.196735522155818));
#82685=CARTESIAN_POINT('Ctrl Pts',(-0.236643307830565,0.0160365523661593,
-0.196517588783739));
#82686=CARTESIAN_POINT('Ctrl Pts',(-0.236787139955247,0.0137505420066819,
-0.196367941629022));
#82687=CARTESIAN_POINT('Ctrl Pts',(-0.237080167909662,0.0076945842123848,
-0.195975440832477));
#82688=CARTESIAN_POINT('Ctrl Pts',(-0.237172572604718,0.00392248085024846,
-0.195734988776373));
#82689=CARTESIAN_POINT('Ctrl Pts',(-0.237174952801866,0.000149627646716525,
-0.195497106204122));
#82690=CARTESIAN_POINT('Ctrl Pts',(-0.0419358257166351,0.233438144154857,
-0.117607078812657));
#82691=CARTESIAN_POINT('Ctrl Pts',(-0.0419265777945186,0.233439805491104,
-0.117607705924788));
#82692=CARTESIAN_POINT('Ctrl Pts',(-0.0419173297741229,0.233441466277719,
-0.1176083330665));
#82693=CARTESIAN_POINT('Ctrl Pts',(-0.0409907050910767,0.233607815415776,
-0.117671173135956));
#82694=CARTESIAN_POINT('Ctrl Pts',(-0.0400723854496901,0.233767091732025,
-0.117733675692303));
#82695=CARTESIAN_POINT('Ctrl Pts',(-0.0383210922081365,0.234060219319985,
-0.117853342829096));
#82696=CARTESIAN_POINT('Ctrl Pts',(-0.0374883115568983,0.234195044310303,
-0.117910453369518));
#82697=CARTESIAN_POINT('Ctrl Pts',(-0.0354829573920695,0.234508736072031,
-0.118048451574336));
#82698=CARTESIAN_POINT('Ctrl Pts',(-0.0343097379480292,0.234683253114481,
-0.118129574214464));
#82699=CARTESIAN_POINT('Ctrl Pts',(-0.0301829751756676,0.23526550599523,
-0.118416165989855));
#82700=CARTESIAN_POINT('Ctrl Pts',(-0.0272232321177378,0.235626322622069,
-0.118623946951721));
#82701=CARTESIAN_POINT('Ctrl Pts',(-0.0197365438543336,0.236396078507233,
-0.119153890339818));
#82702=CARTESIAN_POINT('Ctrl Pts',(-0.0152032701702621,0.236730844555789,
-0.119478771799242));
#82703=CARTESIAN_POINT('Ctrl Pts',(0.00920816932607272,0.237829501948512,
-0.121240927099465));
#82704=CARTESIAN_POINT('Ctrl Pts',(0.029117201024944,0.236220327226059,
-0.122714309179163));
#82705=CARTESIAN_POINT('Ctrl Pts',(0.0546850039237533,0.230868546420666,
-0.12455747527582));
#82706=CARTESIAN_POINT('Ctrl Pts',(0.0607261396610016,0.229353621366613,
-0.124990094419032));
#82707=CARTESIAN_POINT('Ctrl Pts',(0.0689058507610582,0.226956477003981,
-0.125572115740927));
#82708=CARTESIAN_POINT('Ctrl Pts',(0.0711010985469295,0.226278353260724,
-0.125727952190311));
#82709=CARTESIAN_POINT('Ctrl Pts',(0.0746111610970285,0.225137948932055,
-0.125976616958903));
#82710=CARTESIAN_POINT('Ctrl Pts',(0.0759323120642836,0.224695806675034,
-0.126070095440765));
#82711=CARTESIAN_POINT('Ctrl Pts',(0.0786694219798809,0.223752895107317,
-0.126263549669242));
#82712=CARTESIAN_POINT('Ctrl Pts',(0.0800846776646495,0.223250264509662,
-0.126363459171373));
#82713=CARTESIAN_POINT('Ctrl Pts',(0.0834227956687519,0.222028897449522,
-0.126598885737254));
#82714=CARTESIAN_POINT('Ctrl Pts',(0.0853413098005264,0.221298566237656,
-0.126734012150409));
#82715=CARTESIAN_POINT('Ctrl Pts',(0.0918571664609958,0.218720799321267,
-0.127192565796493));
#82716=CARTESIAN_POINT('Ctrl Pts',(0.0964061735817152,0.216754197831421,
-0.127512024565827));
#82717=CARTESIAN_POINT('Ctrl Pts',(0.107500114491197,0.211539699948246,
-0.128292681016182));
#82718=CARTESIAN_POINT('Ctrl Pts',(0.113963004897077,0.20812920176753,-0.128748775612309));
#82719=CARTESIAN_POINT('Ctrl Pts',(0.132637893181025,0.197143225015587,
-0.130088438292451));
#82720=CARTESIAN_POINT('Ctrl Pts',(0.14432942615202,0.188751799029415,-0.130954950075696));
#82721=CARTESIAN_POINT('Ctrl Pts',(0.160275312239641,0.17495437793864,-0.132275617936893));
#82722=CARTESIAN_POINT('Ctrl Pts',(0.165171099072202,0.170339954697062,
-0.132703770185722));
#82723=CARTESIAN_POINT('Ctrl Pts',(0.17098777834711,0.164370783049533,-0.133251513148062));
#82724=CARTESIAN_POINT('Ctrl Pts',(0.172099999711381,0.163205895766076,
-0.13335813626804));
#82725=CARTESIAN_POINT('Ctrl Pts',(0.173836818389356,0.161349339878685,
-0.133527824433443));
#82726=CARTESIAN_POINT('Ctrl Pts',(0.174469374019223,0.160665137356043,
-0.133590308920945));
#82727=CARTESIAN_POINT('Ctrl Pts',(0.175667159942027,0.159354139858835,
-0.133709979431747));
#82728=CARTESIAN_POINT('Ctrl Pts',(0.176233098705831,0.15872803091911,-0.133767111668537));
#82729=CARTESIAN_POINT('Ctrl Pts',(0.177586372071624,0.157214719786741,
-0.133905130840699));
#82730=CARTESIAN_POINT('Ctrl Pts',(0.178370409101057,0.15632461313397,-0.133986252581333));
#82731=CARTESIAN_POINT('Ctrl Pts',(0.181098680804904,0.15317999643998,-0.134272523215124));
#82732=CARTESIAN_POINT('Ctrl Pts',(0.183007025887036,0.150894897072971,
-0.134479973806765));
#82733=CARTESIAN_POINT('Ctrl Pts',(0.187712012965702,0.145040470726881,
-0.135008779438561));
#82734=CARTESIAN_POINT('Ctrl Pts',(0.190450190727485,0.141425803641111,
-0.135332836228307));
#82735=CARTESIAN_POINT('Ctrl Pts',(0.204538553060434,0.12167614015856,-0.137082022024091));
#82736=CARTESIAN_POINT('Ctrl Pts',(0.213947939084654,0.104247613409395,
-0.138542944563336));
#82737=CARTESIAN_POINT('Ctrl Pts',(0.223395288667307,0.0799191575166064,
-0.140385964958119));
#82738=CARTESIAN_POINT('Ctrl Pts',(0.225460482240546,0.0738925624869005,
-0.140828739120122));
#82739=CARTESIAN_POINT('Ctrl Pts',(0.227943403377497,0.0655679821931603,
-0.141422053878623));
#82740=CARTESIAN_POINT('Ctrl Pts',(0.228573449965457,0.0633366723610477,
-0.14157934297761));
#82741=CARTESIAN_POINT('Ctrl Pts',(0.229530911741545,0.0597452637186364,
-0.141829808941046));
#82742=CARTESIAN_POINT('Ctrl Pts',(0.229879175347535,0.0583909313838091,
-0.141923650985323));
#82743=CARTESIAN_POINT('Ctrl Pts',(0.230576592878991,0.055575812476405,
-0.14211748185522));
#82744=CARTESIAN_POINT('Ctrl Pts',(0.230923890977936,0.0541146271189418,
-0.142217407357086));
#82745=CARTESIAN_POINT('Ctrl Pts',(0.231710764031525,0.0506584182208344,
-0.14245221316225));
#82746=CARTESIAN_POINT('Ctrl Pts',(0.232138494345643,0.0486607991953727,
-0.142586711381885));
#82747=CARTESIAN_POINT('Ctrl Pts',(0.233500400352394,0.0418731283491117,
-0.143039850555427));
#82748=CARTESIAN_POINT('Ctrl Pts',(0.23431257204386,0.0370596773168619,
-0.143354663842213));
#82749=CARTESIAN_POINT('Ctrl Pts',(0.235946557497328,0.0251448581549002,
-0.144121031418296));
#82750=CARTESIAN_POINT('Ctrl Pts',(0.236597039528159,0.0180248174690313,
-0.144567751118608));
#82751=CARTESIAN_POINT('Ctrl Pts',(0.237570878337871,-0.00317030612551152,
-0.145880865478057));
#82752=CARTESIAN_POINT('Ctrl Pts',(0.23696454687095,-0.0172553458568963,
-0.146730525182806));
#82753=CARTESIAN_POINT('Ctrl Pts',(0.234167407682442,-0.0383317056288286,
-0.148058975761636));
#82754=CARTESIAN_POINT('Ctrl Pts',(0.232897686118451,-0.0454130042510966,
-0.148515652040689));
#82755=CARTESIAN_POINT('Ctrl Pts',(0.230946169735583,-0.0540234569482967,
-0.149095638372124));
#82756=CARTESIAN_POINT('Ctrl Pts',(0.230567319856711,-0.0556181432819762,
-0.149204111617994));
#82757=CARTESIAN_POINT('Ctrl Pts',(0.229945489618602,-0.0581199979109375,
-0.14937614491087));
#82758=CARTESIAN_POINT('Ctrl Pts',(0.229713588661616,-0.0590299031092129,
-0.149439099770317));
#82759=CARTESIAN_POINT('Ctrl Pts',(0.229263384083825,-0.0607535277025079,
-0.149559133198301));
#82760=CARTESIAN_POINT('Ctrl Pts',(0.229046139894657,-0.0615674923705631,
-0.149616152561482));
#82761=CARTESIAN_POINT('Ctrl Pts',(0.2285157073984,-0.0635132357561912,
-0.149753238110809));
#82762=CARTESIAN_POINT('Ctrl Pts',(0.22819844397826,-0.0646438679636609,
-0.149833530292068));
#82763=CARTESIAN_POINT('Ctrl Pts',(0.22706846509421,-0.0685587739201833,
-0.150113644419974));
#82764=CARTESIAN_POINT('Ctrl Pts',(0.226213116631161,-0.071330339370902,
-0.150315643008835));
#82765=CARTESIAN_POINT('Ctrl Pts',(0.223941650125932,-0.0782382865753364,
-0.150827255781619));
#82766=CARTESIAN_POINT('Ctrl Pts',(0.222461605151747,-0.0823524250290794,
-0.151139370333243));
#82767=CARTESIAN_POINT('Ctrl Pts',(0.214411683574856,-0.102925367467154,
-0.152730596968696));
#82768=CARTESIAN_POINT('Ctrl Pts',(0.206124467374483,-0.118654114988966,
-0.154041890305366));
#82769=CARTESIAN_POINT('Ctrl Pts',(0.191566349298557,-0.140075608869588,
-0.155888979932513));
#82770=CARTESIAN_POINT('Ctrl Pts',(0.186623159193027,-0.146596949990851,
-0.156461833166066));
#82771=CARTESIAN_POINT('Ctrl Pts',(0.179719788495819,-0.154787582462731,
-0.157195319250065));
#82772=CARTESIAN_POINT('Ctrl Pts',(0.178056210160813,-0.156698388469869,
-0.157367530699892));
#82773=CARTESIAN_POINT('Ctrl Pts',(0.175293853077611,-0.159770457507143,
-0.157646313907743));
#82774=CARTESIAN_POINT('Ctrl Pts',(0.174213424026886,-0.16094787082695,
-0.157753635465204));
#82775=CARTESIAN_POINT('Ctrl Pts',(0.172097823575316,-0.163207111328723,
-0.157960535940788));
#82776=CARTESIAN_POINT('Ctrl Pts',(0.171064148464539,-0.164290229024031,
-0.15806017129055));
#82777=CARTESIAN_POINT('Ctrl Pts',(0.168614193105888,-0.166809176932296,
-0.158292991796427));
#82778=CARTESIAN_POINT('Ctrl Pts',(0.167189704132289,-0.168236889155858,
-0.158425812702684));
#82779=CARTESIAN_POINT('Ctrl Pts',(0.162371625139891,-0.172944229295513,
-0.15886687300084));
#82780=CARTESIAN_POINT('Ctrl Pts',(0.158898266649461,-0.176140843480554,
-0.159171561999456));
#82781=CARTESIAN_POINT('Ctrl Pts',(0.150182941314529,-0.183693996772097,
-0.159907308336116));
#82782=CARTESIAN_POINT('Ctrl Pts',(0.144844125561484,-0.187932407448559,
-0.160334047367573));
#82783=CARTESIAN_POINT('Ctrl Pts',(0.131589775265627,-0.197554020956514,
-0.161349293366636));
#82784=CARTESIAN_POINT('Ctrl Pts',(0.123516850480698,-0.2026994111859,-0.161932412291567));
#82785=CARTESIAN_POINT('Ctrl Pts',(0.114501104060991,-0.207706614298023,
-0.162566348917039));
#82786=CARTESIAN_POINT('Ctrl Pts',(0.113845283084768,-0.20806679688921,
-0.162612370318857));
#82787=CARTESIAN_POINT('Ctrl Pts',(0.103213836423129,-0.213840366633772,
-0.163357087997546));
#82788=CARTESIAN_POINT('Ctrl Pts',(0.092865228265687,-0.218533245999777,
-0.164062655014361));
#82789=CARTESIAN_POINT('Ctrl Pts',(0.080607470294182,-0.223063622081155,
-0.164919701229648));
#82790=CARTESIAN_POINT('Ctrl Pts',(0.0789864511814116,-0.223642759486695,
-0.165033463254584));
#82791=CARTESIAN_POINT('Ctrl Pts',(0.0764457488195572,-0.224519402520991,
-0.165212638335533));
#82792=CARTESIAN_POINT('Ctrl Pts',(0.0755302693831734,-0.224829030476986,
-0.16527737471599));
#82793=CARTESIAN_POINT('Ctrl Pts',(0.0739000429001116,-0.225369315422509,
-0.165393006492608));
#82794=CARTESIAN_POINT('Ctrl Pts',(0.0731860555935161,-0.22560218501491,
-0.165443772311477));
#82795=CARTESIAN_POINT('Ctrl Pts',(0.0714517422664168,-0.226158738451587,
-0.165567376111735));
#82796=CARTESIAN_POINT('Ctrl Pts',(0.070430327076123,-0.226478907114379,
-0.16564041194777));
#82797=CARTESIAN_POINT('Ctrl Pts',(0.0672140418516335,-0.227463209645694,
-0.165871067604539));
#82798=CARTESIAN_POINT('Ctrl Pts',(0.0650117612637484,-0.228102409222718,
-0.166029989598631));
#82799=CARTESIAN_POINT('Ctrl Pts',(0.0530858793934686,-0.231377101078858,
-0.166894636839782));
#82800=CARTESIAN_POINT('Ctrl Pts',(0.0432119074080155,-0.233422717921159,
-0.167624510497337));
#82801=CARTESIAN_POINT('Ctrl Pts',(0.0148055467333385,-0.237443408314525,
-0.169716111386987));
#82802=CARTESIAN_POINT('Ctrl Pts',(-0.00387450207890598,-0.237873493384784,
-0.171075953190418));
#82803=CARTESIAN_POINT('Ctrl Pts',(-0.0259760064417461,-0.235775372336707,
-0.172616887618995));
#82804=CARTESIAN_POINT('Ctrl Pts',(-0.0295295429081284,-0.235356724164988,
-0.172862799016053));
#82805=CARTESIAN_POINT('Ctrl Pts',(-0.0348849999033451,-0.234602574580965,
-0.173230770590165));
#82806=CARTESIAN_POINT('Ctrl Pts',(-0.036694606063742,-0.234326348135469,
-0.173354652287345));
#82807=CARTESIAN_POINT('Ctrl Pts',(-0.0399902925233111,-0.233784164398225,
-0.173579484750334));
#82808=CARTESIAN_POINT('Ctrl Pts',(-0.0414773628497172,-0.233524918525139,
-0.173680640838416));
#82809=CARTESIAN_POINT('Ctrl Pts',(-0.0444835890997039,-0.23297121079324,
-0.173884583261272));
#82810=CARTESIAN_POINT('Ctrl Pts',(-0.0460025416331815,-0.232676043273171,
-0.173987341925818));
#82811=CARTESIAN_POINT('Ctrl Pts',(-0.0497625273489416,-0.231907131444321,
-0.174241059670093));
#82812=CARTESIAN_POINT('Ctrl Pts',(-0.0519998231382932,-0.231415742199298,
-0.174391453281907));
#82813=CARTESIAN_POINT('Ctrl Pts',(-0.0607685582511844,-0.229356225207998,
-0.174979029842838));
#82814=CARTESIAN_POINT('Ctrl Pts',(-0.0672396073726376,-0.227543278559063,
-0.17540843185929));
#82815=CARTESIAN_POINT('Ctrl Pts',(-0.0847875059113642,-0.221812843167166,
-0.17657111944796));
#82816=CARTESIAN_POINT('Ctrl Pts',(-0.0956639400839108,-0.217343716207261,
-0.177289149619266));
#82817=CARTESIAN_POINT('Ctrl Pts',(-0.118000538669546,-0.206162648559552,
-0.178821277424981));
#82818=CARTESIAN_POINT('Ctrl Pts',(-0.129318028224345,-0.199258430833094,
-0.179633441489538));
#82819=CARTESIAN_POINT('Ctrl Pts',(-0.141829310345399,-0.190109357917505,
-0.18064238423881));
#82820=CARTESIAN_POINT('Ctrl Pts',(-0.143640102587277,-0.188744910521885,
-0.180791386041895));
#82821=CARTESIAN_POINT('Ctrl Pts',(-0.14627275780133,-0.186701356468941,
-0.181012892041752));
#82822=CARTESIAN_POINT('Ctrl Pts',(-0.147110107769845,-0.186042286229062,
-0.181084086028159));
#82823=CARTESIAN_POINT('Ctrl Pts',(-0.148557252977984,-0.184887373533538,
-0.181208477415839));
#82824=CARTESIAN_POINT('Ctrl Pts',(-0.149169068496573,-0.184394108573547,
-0.181261494207584));
#82825=CARTESIAN_POINT('Ctrl Pts',(-0.150532094357359,-0.183283970887871,
-0.181380578017171));
#82826=CARTESIAN_POINT('Ctrl Pts',(-0.151281957126289,-0.182665527069756,
-0.181446753165607));
#82827=CARTESIAN_POINT('Ctrl Pts',(-0.153315314723421,-0.18096742228859,
-0.181627959386198));
#82828=CARTESIAN_POINT('Ctrl Pts',(-0.154591164189701,-0.179878751433083,
-0.181743594837502));
#82829=CARTESIAN_POINT('Ctrl Pts',(-0.157528416585325,-0.177318090858562,
-0.182014135621691));
#82830=CARTESIAN_POINT('Ctrl Pts',(-0.159180894756273,-0.175836143431599,
-0.182169630790074));
#82831=CARTESIAN_POINT('Ctrl Pts',(-0.164570582929584,-0.170864414105881,
-0.182687122092148));
#82832=CARTESIAN_POINT('Ctrl Pts',(-0.16821558618414,-0.167277120099077,
-0.183053885108616));
#82833=CARTESIAN_POINT('Ctrl Pts',(-0.178810446120136,-0.15615331099749,
-0.18416513338657));
#82834=CARTESIAN_POINT('Ctrl Pts',(-0.185390717457096,-0.148281196006734,
-0.184917292934201));
#82835=CARTESIAN_POINT('Ctrl Pts',(-0.199681143153089,-0.128741083458007,
-0.186676919771659));
#82836=CARTESIAN_POINT('Ctrl Pts',(-0.206911612059503,-0.116766995786366,
-0.187673666215287));
#82837=CARTESIAN_POINT('Ctrl Pts',(-0.214270990595344,-0.101723520058102,
-0.18882355529731));
#82838=CARTESIAN_POINT('Ctrl Pts',(-0.215450359037064,-0.0992011889059501,
-0.189013213581285));
#82839=CARTESIAN_POINT('Ctrl Pts',(-0.217258097298813,-0.0951505485358067,
-0.189312944690432));
#82840=CARTESIAN_POINT('Ctrl Pts',(-0.217915354369932,-0.0936354969931824,
-0.189423992418324));
#82841=CARTESIAN_POINT('Ctrl Pts',(-0.219132039914642,-0.090748685131472,
-0.189633629024345));
#82842=CARTESIAN_POINT('Ctrl Pts',(-0.219694542086868,-0.0893783145813873,
-0.189732317761885));
#82843=CARTESIAN_POINT('Ctrl Pts',(-0.220949413534856,-0.0862377516615316,
-0.189956659415953));
#82844=CARTESIAN_POINT('Ctrl Pts',(-0.221633421666249,-0.0844643114152518,
-0.190082028081883));
#82845=CARTESIAN_POINT('Ctrl Pts',(-0.223704465682497,-0.0788962255196485,
-0.190471729477082));
#82846=CARTESIAN_POINT('Ctrl Pts',(-0.22501595872422,-0.0750741218466543,
-0.190733579167669));
#82847=CARTESIAN_POINT('Ctrl Pts',(-0.232809958768127,-0.050316666738961,
-0.192398034470159));
#82848=CARTESIAN_POINT('Ctrl Pts',(-0.236461512232343,-0.0286036546426776,
-0.193702262630212));
#82849=CARTESIAN_POINT('Ctrl Pts',(-0.237144870573307,-0.00441616317524204,
-0.195210186855258));
#82850=CARTESIAN_POINT('Ctrl Pts',(-0.237176389888194,-0.00213345270163669,
-0.195353155554687));
#82851=CARTESIAN_POINT('Ctrl Pts',(-0.237174953014705,0.000149289894911542,
-0.195497084908503));
#82852=CARTESIAN_POINT('Origin',(0.,0.,-0.7775));
#82853=CARTESIAN_POINT('',(-0.294199934127337,0.000196874250640231,-1.52858238829104));
#82854=CARTESIAN_POINT('',(0.129149509984275,0.264863564072709,-1.56079685779694));
#82855=CARTESIAN_POINT('Ctrl Pts',(-0.294538311519035,0.00019710068779305,
-1.52858238829104));
#82856=CARTESIAN_POINT('Ctrl Pts',(-0.294613795190814,0.0107826090470038,
-1.52915696469556));
#82857=CARTESIAN_POINT('Ctrl Pts',(-0.289298612898278,0.118649030238792,
-1.53501631456641));
#82858=CARTESIAN_POINT('Ctrl Pts',(-0.161137893181224,0.303346279680123,
-1.54575447106838));
#82859=CARTESIAN_POINT('Ctrl Pts',(0.0481708578874521,0.303785786120914,
-1.55591805116582));
#82860=CARTESIAN_POINT('Ctrl Pts',(0.129149509984275,0.264863564072709,
-1.56079685779694));
#82861=CARTESIAN_POINT('',(-0.128892185405329,0.264462557919714,-1.5608));
#82862=CARTESIAN_POINT('Origin',(0.,0.,-1.5608));
#82863=CARTESIAN_POINT('',(-0.294219088584387,0.0003134260107802,-1.54301761170896));
#82864=CARTESIAN_POINT('Ctrl Pts',(-0.128892185405329,0.264462557919714,
-1.5608));
#82865=CARTESIAN_POINT('Ctrl Pts',(-0.216707535766418,0.221663635799285,
-1.55551522653367));
#82866=CARTESIAN_POINT('Ctrl Pts',(-0.288573197476053,0.121171389152581,
-1.54958776376999));
#82867=CARTESIAN_POINT('Ctrl Pts',(-0.294558913961987,0.012149256643495,
-1.54366030100631));
#82868=CARTESIAN_POINT('Ctrl Pts',(-0.294466535937668,0.000313689611749063,
-1.54301761170896));
#82869=CARTESIAN_POINT('',(-0.29419997848679,0.000112509433066526,-1.44301761171429));
#82870=CARTESIAN_POINT('Ctrl Pts',(-0.294199833067583,0.000313405498243621,
-1.54301761170896));
#82871=CARTESIAN_POINT('Ctrl Pts',(-0.294217023327698,-0.0158234258104146,
-1.54214055457276));
#82872=CARTESIAN_POINT('Ctrl Pts',(-0.292902300314846,-0.0320212444901405,
-1.54126349743655));
#82873=CARTESIAN_POINT('Ctrl Pts',(-0.290252026430234,-0.0480354156133036,
-1.54038644030035));
#82874=CARTESIAN_POINT('Ctrl Pts',(-0.287606426933038,-0.0640213419424432,
-1.5395109300627));
#82875=CARTESIAN_POINT('Ctrl Pts',(-0.283630014961905,-0.0798234427950474,
-1.53863541982506));
#82876=CARTESIAN_POINT('Ctrl Pts',(-0.278370984510483,-0.0952010240631088,
-1.53775990958741));
#82877=CARTESIAN_POINT('Ctrl Pts',(-0.273111814349831,-0.110579013845637,
-1.53688437609132));
#82878=CARTESIAN_POINT('Ctrl Pts',(-0.266570184910628,-0.125531664434472,
-1.53600884259523));
#82879=CARTESIAN_POINT('Ctrl Pts',(-0.258844231073643,-0.139833129264471,
-1.53513330909914));
#82880=CARTESIAN_POINT('Ctrl Pts',(-0.251117939135543,-0.154135219951332,
-1.53425773728819));
#82881=CARTESIAN_POINT('Ctrl Pts',(-0.242207642809512,-0.167785355035112,
-1.53338216547723));
#82882=CARTESIAN_POINT('Ctrl Pts',(-0.232256525314706,-0.180583904179579,
-1.53250659366628));
#82883=CARTESIAN_POINT('Ctrl Pts',(-0.22228391538919,-0.193410095639677,
-1.5316291307947));
#82884=CARTESIAN_POINT('Ctrl Pts',(-0.211266563528022,-0.205380423780031,
-1.53075166792313));
#82885=CARTESIAN_POINT('Ctrl Pts',(-0.199386261618759,-0.216330207501624,
-1.52987420505155));
#82886=CARTESIAN_POINT('Ctrl Pts',(-0.195853179539396,-0.219586562848073,
-1.52961325643504));
#82887=CARTESIAN_POINT('Ctrl Pts',(-0.192243996622234,-0.222752935046479,
-1.52935230781854));
#82888=CARTESIAN_POINT('Ctrl Pts',(-0.188564008153101,-0.225825717820706,
-1.52909135920203));
#82889=CARTESIAN_POINT('Ctrl Pts',(-0.175876360259589,-0.236419877617578,
-1.52819167590349));
#82890=CARTESIAN_POINT('Ctrl Pts',(-0.162253493509079,-0.245974552757455,
-1.52729199260495));
#82891=CARTESIAN_POINT('Ctrl Pts',(-0.147890921192098,-0.254326395462509,
-1.5263923093064));
#82892=CARTESIAN_POINT('Ctrl Pts',(-0.133556120734875,-0.262662088817767,
-1.52549436565991));
#82893=CARTESIAN_POINT('Ctrl Pts',(-0.118485095219775,-0.269799118991503,
-1.52459642201342));
#82894=CARTESIAN_POINT('Ctrl Pts',(-0.102903127863606,-0.275616738018369,
-1.52369847836693));
#82895=CARTESIAN_POINT('Ctrl Pts',(-0.0873242018146189,-0.281433221555337,
-1.52280070998216));
#82896=CARTESIAN_POINT('Ctrl Pts',(-0.0712352500269611,-0.285930481905613,
-1.52190294159739));
#82897=CARTESIAN_POINT('Ctrl Pts',(-0.0548822808447564,-0.289035595125025,
-1.52100517321262));
#82898=CARTESIAN_POINT('Ctrl Pts',(-0.0385337861512818,-0.292139858725389,
-1.52010765047465));
#82899=CARTESIAN_POINT('Ctrl Pts',(-0.0219221940289531,-0.293852594565548,
-1.51921012773668));
#82900=CARTESIAN_POINT('Ctrl Pts',(-0.00530292333947626,-0.294152203806219,
-1.51831260499871));
#82901=CARTESIAN_POINT('Ctrl Pts',(0.0113551230825498,-0.294452512088865,
-1.51741298817958));
#82902=CARTESIAN_POINT('Ctrl Pts',(0.0280200919670017,-0.293333120120612,
-1.51651337136045));
#82903=CARTESIAN_POINT('Ctrl Pts',(0.0444369333245589,-0.290824687667173,
-1.51561375454132));
#82904=CARTESIAN_POINT('Ctrl Pts',(0.0588942609324966,-0.288615661644938,
-1.51482151596189));
#82905=CARTESIAN_POINT('Ctrl Pts',(0.0731588662054835,-0.285330278632224,
-1.51402927738247));
#82906=CARTESIAN_POINT('Ctrl Pts',(0.0870651703785879,-0.281021878342145,
-1.51323703880304));
#82907=CARTESIAN_POINT('Ctrl Pts',(0.102861402450364,-0.276127947503798,
-1.51233713151631));
#82908=CARTESIAN_POINT('Ctrl Pts',(0.118291944426169,-0.269883086688625,
-1.51143722422959));
#82909=CARTESIAN_POINT('Ctrl Pts',(0.133113420325067,-0.262363216418312,
-1.51053731694286));
#82910=CARTESIAN_POINT('Ctrl Pts',(0.147907029704503,-0.254857484592285,
-1.50963910161205));
#82911=CARTESIAN_POINT('Ctrl Pts',(0.162093122993974,-0.246081798862244,
-1.50874088628125));
#82912=CARTESIAN_POINT('Ctrl Pts',(0.175448032739809,-0.236160174050857,
-1.50784267095044));
#82913=CARTESIAN_POINT('Ctrl Pts',(0.188801379043309,-0.226239710751495,
-1.50694456077257));
#82914=CARTESIAN_POINT('Ctrl Pts',(0.201323074164483,-0.215174002594547,
-1.50604645059469));
#82915=CARTESIAN_POINT('Ctrl Pts',(0.212818425931049,-0.203130395520293,
-1.50514834041681));
#82916=CARTESIAN_POINT('Ctrl Pts',(0.224311133852135,-0.191089558386165,
-1.50425043679761));
#82917=CARTESIAN_POINT('Ctrl Pts',(0.234777431857193,-0.178071847420231,
-1.5033525331784));
#82918=CARTESIAN_POINT('Ctrl Pts',(0.244060688518756,-0.164280310201043,
-1.50245462955919));
#82919=CARTESIAN_POINT('Ctrl Pts',(0.253366195528285,-0.150455717071274,
-1.50155457382152));
#82920=CARTESIAN_POINT('Ctrl Pts',(0.261482578973351,-0.135854264949523,
-1.50065451808386));
#82921=CARTESIAN_POINT('Ctrl Pts',(0.268297333756601,-0.120707003521333,
-1.4997544623462));
#82922=CARTESIAN_POINT('Ctrl Pts',(0.274283205037668,-0.107402114342831,
-1.49896388103215));
#82923=CARTESIAN_POINT('Ctrl Pts',(0.279265420715235,-0.0936768370847798,
-1.49817329971811));
#82924=CARTESIAN_POINT('Ctrl Pts',(0.283199357402271,-0.0796979545969695,
-1.49738271840406));
#82925=CARTESIAN_POINT('Ctrl Pts',(0.287663489115224,-0.0638350728095948,
-1.49648558675288));
#82926=CARTESIAN_POINT('Ctrl Pts',(0.290805227469212,-0.0475442036619822,
-1.49558845510169));
#82927=CARTESIAN_POINT('Ctrl Pts',(0.292554872675635,-0.0310690597498993,
-1.49469132345051));
#82928=CARTESIAN_POINT('Ctrl Pts',(0.294301078016627,-0.014626306563552,
-1.49379595559243));
#82929=CARTESIAN_POINT('Ctrl Pts',(0.294660472434726,0.00199922976480145,
-1.49290058773435));
#82930=CARTESIAN_POINT('Ctrl Pts',(0.293614361666323,0.0185538843177906,
-1.49200521987627));
#82931=CARTESIAN_POINT('Ctrl Pts',(0.292568453553665,0.0351053318529641,
-1.49111002547157));
#82932=CARTESIAN_POINT('Ctrl Pts',(0.290117576849656,0.0515851321130972,
-1.49021483106686));
#82933=CARTESIAN_POINT('Ctrl Pts',(0.28629515761753,0.0677401116381822,
-1.48931963666216));
#82934=CARTESIAN_POINT('Ctrl Pts',(0.282473802126637,0.0838905953932358,
-1.48842469138114));
#82935=CARTESIAN_POINT('Ctrl Pts',(0.27728185476015,0.099715667866776,-1.48752974610013));
#82936=CARTESIAN_POINT('Ctrl Pts',(0.270803446863671,0.114974489199799,
-1.48663480081912));
#82937=CARTESIAN_POINT('Ctrl Pts',(0.264309524078873,0.130269853293429,
-1.4857377122683));
#82938=CARTESIAN_POINT('Ctrl Pts',(0.256523323413169,0.144995534646025,
-1.48484062371747));
#82939=CARTESIAN_POINT('Ctrl Pts',(0.247576534598606,0.158932374034195,
-1.48394353516664));
#82940=CARTESIAN_POINT('Ctrl Pts',(0.239547701724778,0.1714392696988,-1.48313848944612));
#82941=CARTESIAN_POINT('Ctrl Pts',(0.230585110038212,0.183310912449293,
-1.4823334437256));
#82942=CARTESIAN_POINT('Ctrl Pts',(0.220811679822929,0.194411527574309,
-1.48152839800507));
#82943=CARTESIAN_POINT('Ctrl Pts',(0.209902410249452,0.206802223590211,
-1.48062979223507));
#82944=CARTESIAN_POINT('Ctrl Pts',(0.197912414603261,0.218311041742577,
-1.47973118646507));
#82945=CARTESIAN_POINT('Ctrl Pts',(0.185009421737734,0.228746921002818,
-1.47883258069506));
#82946=CARTESIAN_POINT('Ctrl Pts',(0.172131383146893,0.23916261736438,-1.47793571282072));
#82947=CARTESIAN_POINT('Ctrl Pts',(0.158344418734345,0.248508951470909,
-1.47703884494637));
#82948=CARTESIAN_POINT('Ctrl Pts',(0.143852220535281,0.256632380355771,
-1.47614197707202));
#82949=CARTESIAN_POINT('Ctrl Pts',(0.129362538240474,0.264754398980502,
-1.47524526489756));
#82950=CARTESIAN_POINT('Ctrl Pts',(0.114168527049344,0.271653502815025,
-1.47434855272311));
#82951=CARTESIAN_POINT('Ctrl Pts',(0.0985016927601044,0.277220231086034,
-1.47345184054865));
#82952=CARTESIAN_POINT('Ctrl Pts',(0.0828389927852362,0.282785490355439,
-1.4725553650072));
#82953=CARTESIAN_POINT('Ctrl Pts',(0.0667044661733018,0.287018817653418,
-1.47165888946574));
#82954=CARTESIAN_POINT('Ctrl Pts',(0.0503467484441305,0.289860043678158,
-1.47076241392429));
#82955=CARTESIAN_POINT('Ctrl Pts',(0.0339501292217874,0.292708026631745,
-1.46986380640833));
#82956=CARTESIAN_POINT('Ctrl Pts',(0.0173300454633171,0.294157186473883,
-1.46896519889237));
#82957=CARTESIAN_POINT('Ctrl Pts',(0.000742728730556185,0.294199062462872,
-1.46806659137641));
#82958=CARTESIAN_POINT('Ctrl Pts',(-0.0139783380277216,0.294236226956648,
-1.4672690867863));
#82959=CARTESIAN_POINT('Ctrl Pts',(-0.0286731558972058,0.293165762192075,
-1.4664715821962));
#82960=CARTESIAN_POINT('Ctrl Pts',(-0.0431663430276392,0.291015990676836,
-1.46567407760609));
#82961=CARTESIAN_POINT('Ctrl Pts',(-0.0594954107105255,0.288593903370631,
-1.46477555153918));
#82962=CARTESIAN_POINT('Ctrl Pts',(-0.0756716406703319,0.284785528261025,
-1.46387702547228));
#82963=CARTESIAN_POINT('Ctrl Pts',(-0.0914435276617728,0.279627826313424,
-1.46297849940537));
#82964=CARTESIAN_POINT('Ctrl Pts',(-0.107184988715157,0.274480074216469,
-1.46208170670737));
#82965=CARTESIAN_POINT('Ctrl Pts',(-0.122522891907933,0.267988343099318,
-1.46118491400936));
#82966=CARTESIAN_POINT('Ctrl Pts',(-0.137217684288146,0.260240171992333,
-1.46028812131136));
#82967=CARTESIAN_POINT('Ctrl Pts',(-0.151910059462569,0.252493275413328,
-1.45939147613041));
#82968=CARTESIAN_POINT('Ctrl Pts',(-0.165958812148944,0.243490670498873,
-1.45849483094946));
#82969=CARTESIAN_POINT('Ctrl Pts',(-0.179146280018388,0.233367200685044,
-1.45759818576851));
#82970=CARTESIAN_POINT('Ctrl Pts',(-0.192330331990485,0.223246353113332,
-1.45670177284199));
#82971=CARTESIAN_POINT('Ctrl Pts',(-0.204652921497238,0.212005707492377,
-1.45580535991548));
#82972=CARTESIAN_POINT('Ctrl Pts',(-0.215928460295286,0.199821270225437,
-1.45490894698896));
#82973=CARTESIAN_POINT('Ctrl Pts',(-0.227230926056984,0.187607735466548,
-1.45401039335071));
#82974=CARTESIAN_POINT('Ctrl Pts',(-0.237480827513171,0.174446508563989,
-1.45311183971245));
#82975=CARTESIAN_POINT('Ctrl Pts',(-0.246531858943066,0.16054806920694,
-1.4522132860742));
#82976=CARTESIAN_POINT('Ctrl Pts',(-0.254568442804848,0.148207379164488,
-1.4514154431185));
#82977=CARTESIAN_POINT('Ctrl Pts',(-0.261660267585032,0.135286274905178,
-1.4506176001628));
#82978=CARTESIAN_POINT('Ctrl Pts',(-0.267735737189512,0.12194759133164,
-1.4498197572071));
#82979=CARTESIAN_POINT('Ctrl Pts',(-0.275189887420251,0.105582016699494,
-1.44884086312327));
#82980=CARTESIAN_POINT('Ctrl Pts',(-0.281154975269878,0.0884973724728511,
-1.44786196903944));
#82981=CARTESIAN_POINT('Ctrl Pts',(-0.285512149944728,0.0709679662519578,
-1.44688307495561));
#82982=CARTESIAN_POINT('Ctrl Pts',(-0.289842117365214,0.0535480178906884,
-1.44591029332362));
#82983=CARTESIAN_POINT('Ctrl Pts',(-0.292583943111203,0.0356893481811567,
-1.44493751169162));
#82984=CARTESIAN_POINT('Ctrl Pts',(-0.29366817978795,0.0176816339751797,
-1.44396473005963));
#82985=CARTESIAN_POINT('Ctrl Pts',(-0.294020057473362,0.0118374184729343,
-1.44364902394452));
#82986=CARTESIAN_POINT('Ctrl Pts',(-0.294197735516373,0.00597763407621125,
-1.4433333178294));
#82987=CARTESIAN_POINT('Ctrl Pts',(-0.29419997848679,0.000112509433066627,
-1.44301761171429));
#82988=CARTESIAN_POINT('',(-0.294199881040649,-0.000264566943933203,-1.34301761170622));
#82989=CARTESIAN_POINT('Ctrl Pts',(-0.294199978486827,0.000112509333972839,
-1.44301761170896));
#82990=CARTESIAN_POINT('Ctrl Pts',(-0.294206483659082,-0.0168978263402081,
-1.44210198462188));
#82991=CARTESIAN_POINT('Ctrl Pts',(-0.292733371950329,-0.0338987372162774,
-1.44118635753479));
#82992=CARTESIAN_POINT('Ctrl Pts',(-0.289811541802209,-0.050625193710509,
-1.44027073044771));
#82993=CARTESIAN_POINT('Ctrl Pts',(-0.286887052022081,-0.0673668756685116,
-1.43935426989975));
#82994=CARTESIAN_POINT('Ctrl Pts',(-0.282511400153008,-0.0838328853838791,
-1.4384378093518));
#82995=CARTESIAN_POINT('Ctrl Pts',(-0.276766242696575,-0.0997701704098992,
-1.43752134880384));
#82996=CARTESIAN_POINT('Ctrl Pts',(-0.27100445262236,-0.115753594949471,
-1.43660223504087));
#82997=CARTESIAN_POINT('Ctrl Pts',(-0.263865555093411,-0.131204564891129,
-1.4356831212779));
#82998=CARTESIAN_POINT('Ctrl Pts',(-0.255478857719724,-0.145891032137774,
-1.43476400751493));
#82999=CARTESIAN_POINT('Ctrl Pts',(-0.253049934293915,-0.150144470976485,
-1.43449781727933));
#83000=CARTESIAN_POINT('Ctrl Pts',(-0.250516628906551,-0.154333967966321,
-1.43423162704372));
#83001=CARTESIAN_POINT('Ctrl Pts',(-0.247882742893601,-0.158454364962109,
-1.43396543680811));
#83002=CARTESIAN_POINT('Ctrl Pts',(-0.238993368333329,-0.172360719319312,
-1.43306704382643));
#83003=CARTESIAN_POINT('Ctrl Pts',(-0.22890188787328,-0.185560863680223,
-1.43216865084475));
#83004=CARTESIAN_POINT('Ctrl Pts',(-0.21774480709357,-0.197840438191447,
-1.43127025786306));
#83005=CARTESIAN_POINT('Ctrl Pts',(-0.206609320701942,-0.210096245742237,
-1.43037360370958));
#83006=CARTESIAN_POINT('Ctrl Pts',(-0.194412805089058,-0.221434397337263,
-1.4294769495561));
#83007=CARTESIAN_POINT('Ctrl Pts',(-0.181333039984309,-0.231672114442047,
-1.42858029540262));
#83008=CARTESIAN_POINT('Ctrl Pts',(-0.168255519859482,-0.2419080743693,
-1.42768379514873));
#83009=CARTESIAN_POINT('Ctrl Pts',(-0.154295639738224,-0.251043447384909,
-1.42678729489485));
#83010=CARTESIAN_POINT('Ctrl Pts',(-0.139665399961993,-0.258934771812239,
-1.42589079464096));
#83011=CARTESIAN_POINT('Ctrl Pts',(-0.125039011724739,-0.266824018779181,
-1.42499453039863));
#83012=CARTESIAN_POINT('Ctrl Pts',(-0.109743315736894,-0.273469501436223,
-1.4240982661563));
#83013=CARTESIAN_POINT('Ctrl Pts',(-0.0940147633797387,-0.278773858650075,
-1.42320200191398));
#83014=CARTESIAN_POINT('Ctrl Pts',(-0.0782486995485523,-0.284090866377042,
-1.42230360014544));
#83015=CARTESIAN_POINT('Ctrl Pts',(-0.0620484787177007,-0.288060131993999,
-1.42140519837691));
#83016=CARTESIAN_POINT('Ctrl Pts',(-0.0456659476067264,-0.290634239602253,
-1.42050679660837));
#83017=CARTESIAN_POINT('Ctrl Pts',(-0.0311040493667709,-0.292922280003103,
-1.41970823654196));
#83018=CARTESIAN_POINT('Ctrl Pts',(-0.0163986702893981,-0.294108744107576,
-1.41890967647555));
#83019=CARTESIAN_POINT('Ctrl Pts',(-0.00172821287218314,-0.294194923953947,
-1.41811111640913));
#83020=CARTESIAN_POINT('Ctrl Pts',(0.0147757332526237,-0.294291874410302,
-1.41721275366974));
#83021=CARTESIAN_POINT('Ctrl Pts',(0.0313402951844906,-0.292996035529911,
-1.41631439093035));
#83022=CARTESIAN_POINT('Ctrl Pts',(0.047711361023731,-0.290305470202101,
-1.41541602819095));
#83023=CARTESIAN_POINT('Ctrl Pts',(0.0640507438107881,-0.287620111946484,
-1.41451940406001));
#83024=CARTESIAN_POINT('Ctrl Pts',(0.0801965916035031,-0.283545447123526,
-1.41362277992908));
#83025=CARTESIAN_POINT('Ctrl Pts',(0.0958988663854379,-0.278131349232674,
-1.41272615579814));
#83026=CARTESIAN_POINT('Ctrl Pts',(0.111598459935975,-0.272718175822477,
-1.41182968476966));
#83027=CARTESIAN_POINT('Ctrl Pts',(0.126853868205815,-0.265966230750605,
-1.41093321374117));
#83028=CARTESIAN_POINT('Ctrl Pts',(0.141429454492969,-0.257975482171894,
-1.41003674271269));
#83029=CARTESIAN_POINT('Ctrl Pts',(0.156001209790034,-0.249986833850284,
-1.40914050730914));
#83030=CARTESIAN_POINT('Ctrl Pts',(0.169892809329383,-0.240760418453787,
-1.4082442719056));
#83031=CARTESIAN_POINT('Ctrl Pts',(0.182894023142827,-0.230441785053473,
-1.40734803650205));
#83032=CARTESIAN_POINT('Ctrl Pts',(0.195926263307315,-0.220098527064504,
-1.4064496623048));
#83033=CARTESIAN_POINT('Ctrl Pts',(0.208063268358004,-0.20865836005635,
-1.40555128810755));
#83034=CARTESIAN_POINT('Ctrl Pts',(0.219128364473481,-0.196306902281039,
-1.4046529139103));
#83035=CARTESIAN_POINT('Ctrl Pts',(0.228965866838071,-0.185325750937871,
-1.40385420794358));
#83036=CARTESIAN_POINT('Ctrl Pts',(0.237956405352934,-0.173625154600472,
-1.40305550197687));
#83037=CARTESIAN_POINT('Ctrl Pts',(0.24600404911102,-0.161355656303034,
-1.40225679601015));
#83038=CARTESIAN_POINT('Ctrl Pts',(0.25505536946571,-0.147555945105597,
-1.40135847796933));
#83039=CARTESIAN_POINT('Ctrl Pts',(0.26297071114369,-0.132948365572465,
-1.40046015992852));
#83040=CARTESIAN_POINT('Ctrl Pts',(0.269610320154723,-0.117745128417561,
-1.3995618418877));
#83041=CARTESIAN_POINT('Ctrl Pts',(0.276237069189704,-0.102571337765516,
-1.39866526376085));
#83042=CARTESIAN_POINT('Ctrl Pts',(0.28159261699149,-0.086804869870417,
-1.39776868563401));
#83043=CARTESIAN_POINT('Ctrl Pts',(0.285582909949582,-0.0706826820708495,
-1.39687210750716));
#83044=CARTESIAN_POINT('Ctrl Pts',(0.289572515582222,-0.0545632713079921,
-1.39597568381534));
#83045=CARTESIAN_POINT('Ctrl Pts',(0.292197092671192,-0.0380890151960811,
-1.39507926012351));
#83046=CARTESIAN_POINT('Ctrl Pts',(0.293412462568779,-0.0215120154640292,
-1.39418283643168));
#83047=CARTESIAN_POINT('Ctrl Pts',(0.294627511901832,-0.00493938806193824,
-1.39328664917952));
#83048=CARTESIAN_POINT('Ctrl Pts',(0.294434045039363,0.0117351391589708,
-1.39239046192735));
#83049=CARTESIAN_POINT('Ctrl Pts',(0.292839952512838,0.0282560119669929,
-1.39149427467518));
#83050=CARTESIAN_POINT('Ctrl Pts',(0.291242056236625,0.0448163061158407,
-1.39059594898254));
#83051=CARTESIAN_POINT('Ctrl Pts',(0.288236962203357,0.0612214253628249,
-1.3896976232899));
#83052=CARTESIAN_POINT('Ctrl Pts',(0.283884433831552,0.0772222003580513,
-1.38879929759725));
#83053=CARTESIAN_POINT('Ctrl Pts',(0.280013441465023,0.0914527515627984,
-1.38800035693522));
#83054=CARTESIAN_POINT('Ctrl Pts',(0.275077547695713,0.10536325850791,-1.38720141627319));
#83055=CARTESIAN_POINT('Ctrl Pts',(0.269151047893426,0.118791217764071,
-1.38640247561116));
#83056=CARTESIAN_POINT('Ctrl Pts',(0.262487121855226,0.133889999559775,
-1.38550412385915));
#83057=CARTESIAN_POINT('Ctrl Pts',(0.254527548677776,0.148474275772685,
-1.38460577210714));
#83058=CARTESIAN_POINT('Ctrl Pts',(0.245374517644184,0.162311386202213,
-1.38370742035513));
#83059=CARTESIAN_POINT('Ctrl Pts',(0.236239207109633,0.176121707636796,
-1.38281080783477));
#83060=CARTESIAN_POINT('Ctrl Pts',(0.225915401710059,0.189187046186855,
-1.38191419531442));
#83061=CARTESIAN_POINT('Ctrl Pts',(0.214550900598436,0.201299654874021,
-1.38101758279407));
#83062=CARTESIAN_POINT('Ctrl Pts',(0.203188350100266,0.21341018454186,-1.38012112416912));
#83063=CARTESIAN_POINT('Ctrl Pts',(0.190785959733452,0.224567697913147,
-1.37922466554417));
#83064=CARTESIAN_POINT('Ctrl Pts',(0.177531347443001,0.234598083272376,
-1.37832820691922));
#83065=CARTESIAN_POINT('Ctrl Pts',(0.164280225750256,0.24462582713298,-1.37743198437634));
#83066=CARTESIAN_POINT('Ctrl Pts',(0.150177965276877,0.253526563565899,
-1.37653576183347));
#83067=CARTESIAN_POINT('Ctrl Pts',(0.135443381568157,0.26116801180348,-1.3756395392906));
#83068=CARTESIAN_POINT('Ctrl Pts',(0.120673642665631,0.268827691746758,
-1.37474117845337));
#83069=CARTESIAN_POINT('Ctrl Pts',(0.105269284870452,0.275221740729953,
-1.37384281761614));
#83070=CARTESIAN_POINT('Ctrl Pts',(0.089471957604124,0.280264890420627,
-1.37294445677891));
#83071=CARTESIAN_POINT('Ctrl Pts',(0.0754259460574661,0.284748948868774,
-1.37214568959));
#83072=CARTESIAN_POINT('Ctrl Pts',(0.0610699287857648,0.288165653089362,
-1.37134692240109));
#83073=CARTESIAN_POINT('Ctrl Pts',(0.046580566216322,0.290489054614743,
-1.37054815521218));
#83074=CARTESIAN_POINT('Ctrl Pts',(0.0302848996917963,0.293102100998165,
-1.36964981039689));
#83075=CARTESIAN_POINT('Ctrl Pts',(0.0137168745443692,0.294347968966909,
-1.36875146558159));
#83076=CARTESIAN_POINT('Ctrl Pts',(-0.00287267759169578,0.294185974722545,
-1.3678531207663));
#83077=CARTESIAN_POINT('Ctrl Pts',(-0.0194301111209985,0.294024294111087,
-1.36695651521338));
#83078=CARTESIAN_POINT('Ctrl Pts',(-0.0360082063535757,0.292460103685732,
-1.36605990966046));
#83079=CARTESIAN_POINT('Ctrl Pts',(-0.0523522525572313,0.289504545132169,
-1.36516330410754));
#83080=CARTESIAN_POINT('Ctrl Pts',(-0.0686934944870301,0.286549493686544,
-1.36426685239214));
#83081=CARTESIAN_POINT('Ctrl Pts',(-0.0847999817327795,0.282203636625161,
-1.36337040067673));
#83082=CARTESIAN_POINT('Ctrl Pts',(-0.100423593422299,0.276529820967202,
-1.36247394896133));
#83083=CARTESIAN_POINT('Ctrl Pts',(-0.116043090950082,0.270857499393694,
-1.36157773330834));
#83084=CARTESIAN_POINT('Ctrl Pts',(-0.131179225375831,0.263858193884227,
-1.36068151765534));
#83085=CARTESIAN_POINT('Ctrl Pts',(-0.145602031196717,0.255643674890247,
-1.35978530200234));
#83086=CARTESIAN_POINT('Ctrl Pts',(-0.160059251500703,0.247409555103702,
-1.35888694787513));
#83087=CARTESIAN_POINT('Ctrl Pts',(-0.173799066667942,0.237954846934015,
-1.35798859374791));
#83088=CARTESIAN_POINT('Ctrl Pts',(-0.186618561891959,0.227436040146185,
-1.35709023962069));
#83089=CARTESIAN_POINT('Ctrl Pts',(-0.19801744460195,0.218082891466906,
-1.35629143801819));
#83090=CARTESIAN_POINT('Ctrl Pts',(-0.208688840866842,0.207889311073367,
-1.35549263641569));
#83091=CARTESIAN_POINT('Ctrl Pts',(-0.218514934030968,0.196989501256899,
-1.35469383481319));
#83092=CARTESIAN_POINT('Ctrl Pts',(-0.22945360436519,0.184855540760436,
-1.35380458745453));
#83093=CARTESIAN_POINT('Ctrl Pts',(-0.239416908998826,0.171764825371417,
-1.35291534009586));
#83094=CARTESIAN_POINT('Ctrl Pts',(-0.248235545782208,0.157901088692287,
-1.3520260927372));
#83095=CARTESIAN_POINT('Ctrl Pts',(-0.257037908143505,0.144062936954223,
-1.35113848644701));
#83096=CARTESIAN_POINT('Ctrl Pts',(-0.264699303159667,0.129455229767417,
-1.35025088015683));
#83097=CARTESIAN_POINT('Ctrl Pts',(-0.271091546655065,0.11429354020313,
-1.34936327386664));
#83098=CARTESIAN_POINT('Ctrl Pts',(-0.277477009665882,0.0991479331930178,
-1.34847660909265));
#83099=CARTESIAN_POINT('Ctrl Pts',(-0.28259565539752,0.0834502416635364,
-1.34758994431865));
#83100=CARTESIAN_POINT('Ctrl Pts',(-0.286366446301408,0.067438108163728,
-1.34670327954466));
#83101=CARTESIAN_POINT('Ctrl Pts',(-0.290139385992626,0.051416850140588,
-1.34581610950425));
#83102=CARTESIAN_POINT('Ctrl Pts',(-0.292562755010656,0.0350815797868516,
-1.34492893946383));
#83103=CARTESIAN_POINT('Ctrl Pts',(-0.293606252845568,0.0186817635672989,
-1.34404176942342));
#83104=CARTESIAN_POINT('Ctrl Pts',(-0.294007794192005,0.0123710611721357,
-1.3437003835186));
#83105=CARTESIAN_POINT('Ctrl Pts',(-0.294205560350854,0.00605085811264825,
-1.34335899761378));
#83106=CARTESIAN_POINT('Ctrl Pts',(-0.294199881040695,-0.000264566893242766,
-1.34301761170896));
#83107=CARTESIAN_POINT('',(-0.29419998971568,7.7790063860881E-5,-1.24301761170439));
#83108=CARTESIAN_POINT('Ctrl Pts',(-0.294199881040649,-0.000264566943932752,
-1.34301761170622));
#83109=CARTESIAN_POINT('Ctrl Pts',(-0.294180940205162,-0.0213268790539207,
-1.34187906972835));
#83110=CARTESIAN_POINT('Ctrl Pts',(-0.291896264550366,-0.0422876901627163,
-1.34074052775048));
#83111=CARTESIAN_POINT('Ctrl Pts',(-0.287433256096504,-0.0627356620253717,
-1.33960198577262));
#83112=CARTESIAN_POINT('Ctrl Pts',(-0.286436977175878,-0.0673002698559217,
-1.33934782865315));
#83113=CARTESIAN_POINT('Ctrl Pts',(-0.285332333255084,-0.0718394125108084,
-1.33909367153368));
#83114=CARTESIAN_POINT('Ctrl Pts',(-0.2841206116624,-0.0763486609482029,
-1.33883951441421));
#83115=CARTESIAN_POINT('Ctrl Pts',(-0.279837657272212,-0.0922870625645441,
-1.33794116997833));
#83116=CARTESIAN_POINT('Ctrl Pts',(-0.2741957617379,-0.107914611675097,
-1.33704282554245));
#83117=CARTESIAN_POINT('Ctrl Pts',(-0.267260427871627,-0.122985786552246,
-1.33614448110656));
#83118=CARTESIAN_POINT('Ctrl Pts',(-0.260338521832277,-0.138027781417061,
-1.3352478759977));
#83119=CARTESIAN_POINT('Ctrl Pts',(-0.252128415570261,-0.152514802477171,
-1.33435127088884));
#83120=CARTESIAN_POINT('Ctrl Pts',(-0.242744488248793,-0.166218992371003,
-1.33345466577998));
#83121=CARTESIAN_POINT('Ctrl Pts',(-0.233362171982384,-0.179920829496778,
-1.33255821460243));
#83122=CARTESIAN_POINT('Ctrl Pts',(-0.222806836889673,-0.192839421876937,
-1.33166176342487));
#83123=CARTESIAN_POINT('Ctrl Pts',(-0.211237345551264,-0.204774080011255,
-1.33076531224732));
#83124=CARTESIAN_POINT('Ctrl Pts',(-0.199670901482741,-0.216705594694987,
-1.32986909718461));
#83125=CARTESIAN_POINT('Ctrl Pts',(-0.187091390110108,-0.227653129150242,
-1.32897288212191));
#83126=CARTESIAN_POINT('Ctrl Pts',(-0.173694887112703,-0.237452576719869,
-1.3280766670592));
#83127=CARTESIAN_POINT('Ctrl Pts',(-0.160266419626245,-0.247275406088062,
-1.32717831359839));
#83128=CARTESIAN_POINT('Ctrl Pts',(-0.146017724105643,-0.255944229945598,
-1.32627996013759));
#83129=CARTESIAN_POINT('Ctrl Pts',(-0.131174613722805,-0.263337921148233,
-1.32538160667678));
#83130=CARTESIAN_POINT('Ctrl Pts',(-0.117976312901667,-0.269912295262152,
-1.32458280245626));
#83131=CARTESIAN_POINT('Ctrl Pts',(-0.104308786152013,-0.27547899508879,
-1.32378399823574));
#83132=CARTESIAN_POINT('Ctrl Pts',(-0.0903426948984102,-0.279985423689328,
-1.32298519401522));
#83133=CARTESIAN_POINT('Ctrl Pts',(-0.0746362911582433,-0.285053397665801,
-1.32208685092344));
#83134=CARTESIAN_POINT('Ctrl Pts',(-0.0584521846111506,-0.288811738808585,
-1.32118850783167));
#83135=CARTESIAN_POINT('Ctrl Pts',(-0.0420320653633554,-0.291181980007848,
-1.32029016473989));
#83136=CARTESIAN_POINT('Ctrl Pts',(-0.0256437381718955,-0.293547632029614,
-1.31939356098835));
#83137=CARTESIAN_POINT('Ctrl Pts',(-0.00902106987274824,-0.294530342122439,
-1.31849695723682));
#83138=CARTESIAN_POINT('Ctrl Pts',(0.00758251067853928,-0.294102270531545,
-1.31760035348528));
#83139=CARTESIAN_POINT('Ctrl Pts',(0.0241832406835549,-0.293674272433104,
-1.31670390366503));
#83140=CARTESIAN_POINT('Ctrl Pts',(0.0407640997441511,-0.291835941239725,
-1.31580745384478));
#83141=CARTESIAN_POINT('Ctrl Pts',(0.0570702851055986,-0.288611542662392,
-1.31491100402452));
#83142=CARTESIAN_POINT('Ctrl Pts',(0.0733721755573099,-0.285387993364062,
-1.31401479032149));
#83143=CARTESIAN_POINT('Ctrl Pts',(0.0893987618351136,-0.280779265739622,
-1.31311857661845));
#83144=CARTESIAN_POINT('Ctrl Pts',(0.104905721807555,-0.274860745709597,
-1.31222236291541));
#83145=CARTESIAN_POINT('Ctrl Pts',(0.120449682375012,-0.268928103713493,
-1.31132401078935));
#83146=CARTESIAN_POINT('Ctrl Pts',(0.135470807684591,-0.261679735676709,
-1.31042565866328));
#83147=CARTESIAN_POINT('Ctrl Pts',(0.149744688774196,-0.253239349596225,
-1.30952730653722));
#83148=CARTESIAN_POINT('Ctrl Pts',(0.162436964464623,-0.24573419340257,
-1.30872849556356));
#83149=CARTESIAN_POINT('Ctrl Pts',(0.174538440607036,-0.237287454248982,
-1.3079296845899));
#83150=CARTESIAN_POINT('Ctrl Pts',(0.185912204337808,-0.22801379843829,
-1.30713087361624));
#83151=CARTESIAN_POINT('Ctrl Pts',(0.198703134631412,-0.217584648699535,
-1.30623253110415));
#83152=CARTESIAN_POINT('Ctrl Pts',(0.210654423871686,-0.206042693857774,
-1.30533418859206));
#83153=CARTESIAN_POINT('Ctrl Pts',(0.221568841233891,-0.193548155750116,
-1.30443584607996));
#83154=CARTESIAN_POINT('Ctrl Pts',(0.23246212621466,-0.181077809437253,
-1.30353924292931));
#83155=CARTESIAN_POINT('Ctrl Pts',(0.242321960369317,-0.167659086567259,
-1.30264263977865));
#83156=CARTESIAN_POINT('Ctrl Pts',(0.250987228407161,-0.153489580025784,
-1.30174603662799));
#83157=CARTESIAN_POINT('Ctrl Pts',(0.259651008537639,-0.139322506520779,
-1.30084958743245));
#83158=CARTESIAN_POINT('Ctrl Pts',(0.267120173459694,-0.124405550612861,
-1.29995313823692));
#83159=CARTESIAN_POINT('Ctrl Pts',(0.273276597785878,-0.108965779502444,
-1.29905668904139));
#83160=CARTESIAN_POINT('Ctrl Pts',(0.279431400464002,-0.093530075342835,
-1.29816047597725));
#83161=CARTESIAN_POINT('Ctrl Pts',(0.284273866166556,-0.0775725684430892,
-1.29726426291312));
#83162=CARTESIAN_POINT('Ctrl Pts',(0.2877344757355,-0.0613393142545369,
-1.29636804984899));
#83163=CARTESIAN_POINT('Ctrl Pts',(0.291203342505222,-0.0450673266473652,
-1.29546969837222));
#83164=CARTESIAN_POINT('Ctrl Pts',(0.293283628383432,-0.0285190601876433,
-1.29457134689546));
#83165=CARTESIAN_POINT('Ctrl Pts',(0.293957198634491,-0.0119501201233388,
-1.2936729954187));
#83166=CARTESIAN_POINT('Ctrl Pts',(0.294556137252256,0.00278298016478098,
-1.29287418135155));
#83167=CARTESIAN_POINT('Ctrl Pts',(0.294043594649531,0.0175319521840072,
-1.2920753672844));
#83168=CARTESIAN_POINT('Ctrl Pts',(0.292441404009112,0.0321195457810242,
-1.29127655321725));
#83169=CARTESIAN_POINT('Ctrl Pts',(0.290639586612288,0.0485246971143476,
-1.29037821000721));
#83170=CARTESIAN_POINT('Ctrl Pts',(0.287447319294331,0.0648299086200134,
-1.28947986679716));
#83171=CARTESIAN_POINT('Ctrl Pts',(0.28289188937104,0.0807825409855569,
-1.28858152358712));
#83172=CARTESIAN_POINT('Ctrl Pts',(0.278345279537461,0.0967042863325372,
-1.28768491972283));
#83173=CARTESIAN_POINT('Ctrl Pts',(0.272440897570094,0.112274037639596,
-1.28678831585854));
#83174=CARTESIAN_POINT('Ctrl Pts',(0.265257029552737,0.127249158240274,
-1.28589171199425));
#83175=CARTESIAN_POINT('Ctrl Pts',(0.258074394962931,0.142221707701522,
-1.28499526207153));
#83176=CARTESIAN_POINT('Ctrl Pts',(0.24961300411642,0.156599095364782,-1.28409881214881));
#83177=CARTESIAN_POINT('Ctrl Pts',(0.239999249875403,0.170158749581806,
-1.28320236222609));
#83178=CARTESIAN_POINT('Ctrl Pts',(0.230388027873357,0.183714832219614,
-1.28230614842605));
#83179=CARTESIAN_POINT('Ctrl Pts',(0.219625511684055,0.1964529698853,-1.28140993462602));
#83180=CARTESIAN_POINT('Ctrl Pts',(0.20788045172467,0.208181069722362,-1.28051372082598));
#83181=CARTESIAN_POINT('Ctrl Pts',(0.196107367454748,0.219937153402248,
-1.27961536861422));
#83182=CARTESIAN_POINT('Ctrl Pts',(0.18334763810206,0.230677843492465,-1.27871701640246));
#83183=CARTESIAN_POINT('Ctrl Pts',(0.169805959154214,0.240248988001443,
-1.27781866419071));
#83184=CARTESIAN_POINT('Ctrl Pts',(0.157764763491979,0.248759603574887,
-1.27701985373323));
#83185=CARTESIAN_POINT('Ctrl Pts',(0.14510612512367,0.256345890152774,-1.27622104327575));
#83186=CARTESIAN_POINT('Ctrl Pts',(0.131990690368428,0.262929834092797,
-1.27542223281827));
#83187=CARTESIAN_POINT('Ctrl Pts',(0.117241060436347,0.270334143474923,
-1.27452388984653));
#83188=CARTESIAN_POINT('Ctrl Pts',(0.101819564026194,0.276517006092301,
-1.27362554687479));
#83189=CARTESIAN_POINT('Ctrl Pts',(0.0859530949446297,0.281364008838088,
-1.27272720390305));
#83190=CARTESIAN_POINT('Ctrl Pts',(0.0701173461179693,0.286201626940126,
-1.27183060028018));
#83191=CARTESIAN_POINT('Ctrl Pts',(0.0538390633948679,0.289708227895976,
-1.27093399665731));
#83192=CARTESIAN_POINT('Ctrl Pts',(0.0373644639970419,0.291817643109894,
-1.27003739303444));
#83193=CARTESIAN_POINT('Ctrl Pts',(0.0208926932127655,0.293926696146845,
-1.26914094335432));
#83194=CARTESIAN_POINT('Ctrl Pts',(0.00422544821317553,0.294638887359161,
-1.2682444936742));
#83195=CARTESIAN_POINT('Ctrl Pts',(-0.0123817484947549,0.293939334394383,
-1.26734804399409));
#83196=CARTESIAN_POINT('Ctrl Pts',(-0.0289845708872543,0.293239965691005,
-1.26645183043772));
#83197=CARTESIAN_POINT('Ctrl Pts',(-0.045526586286276,0.291129635322151,
-1.26555561688136));
#83198=CARTESIAN_POINT('Ctrl Pts',(-0.06175483299394,0.287645581578947,
-1.264659403325));
#83199=CARTESIAN_POINT('Ctrl Pts',(-0.0780218011952776,0.284153214690928,
-1.26376105135355));
#83200=CARTESIAN_POINT('Ctrl Pts',(-0.0939727343393061,0.279280770795784,
-1.26286269938211));
#83201=CARTESIAN_POINT('Ctrl Pts',(-0.109366980510989,0.2731162821472,-1.26196434741066));
#83202=CARTESIAN_POINT('Ctrl Pts',(-0.123055494354213,0.267634838803923,
-1.26116553574687));
#83203=CARTESIAN_POINT('Ctrl Pts',(-0.136303736560469,0.261132715282318,
-1.26036672408307));
#83204=CARTESIAN_POINT('Ctrl Pts',(-0.148958906168924,0.253702353700075,
-1.25956791241928));
#83205=CARTESIAN_POINT('Ctrl Pts',(-0.163190899122558,0.245346175398775,
-1.25866956950314));
#83206=CARTESIAN_POINT('Ctrl Pts',(-0.17676280583108,0.235762144364244,
-1.25777122658699));
#83207=CARTESIAN_POINT('Ctrl Pts',(-0.189455265116077,0.22507852523019,
-1.25687288367085));
#83208=CARTESIAN_POINT('Ctrl Pts',(-0.202123149546261,0.214415591479732,
-1.25597628010609));
#83209=CARTESIAN_POINT('Ctrl Pts',(-0.213914325929049,0.202657748893602,
-1.25507967654134));
#83210=CARTESIAN_POINT('Ctrl Pts',(-0.2246394260358,0.189975704421135,-1.25418307297659));
#83211=CARTESIAN_POINT('Ctrl Pts',(-0.235362684655307,0.177295837440989,
-1.25328662335763));
#83212=CARTESIAN_POINT('Ctrl Pts',(-0.245019680993877,0.16369265179071,
-1.25239017373867));
#83213=CARTESIAN_POINT('Ctrl Pts',(-0.253459038149679,0.149372540917799,
-1.25149372411971));
#83214=CARTESIAN_POINT('Ctrl Pts',(-0.261896172372185,0.135056201973327,
-1.25059751062628));
#83215=CARTESIAN_POINT('Ctrl Pts',(-0.269115911868186,0.12002399997494,
-1.24970129713285));
#83216=CARTESIAN_POINT('Ctrl Pts',(-0.275012021059745,0.104508508135148,
-1.24880508363943));
#83217=CARTESIAN_POINT('Ctrl Pts',(-0.280922198683778,0.0889559955004315,
-1.24790673173258));
#83218=CARTESIAN_POINT('Ctrl Pts',(-0.285502181001382,0.0729186419795194,
-1.24700837982573));
#83219=CARTESIAN_POINT('Ctrl Pts',(-0.288695059045791,0.0566462962826991,
-1.24611002791888));
#83220=CARTESIAN_POINT('Ctrl Pts',(-0.291534157142027,0.0421769726672756,
-1.24531121595269));
#83221=CARTESIAN_POINT('Ctrl Pts',(-0.29327720565083,0.0275224345870245,
-1.24451240398649));
#83222=CARTESIAN_POINT('Ctrl Pts',(-0.293918747058194,0.0128611868714064,
-1.2437135920203));
#83223=CARTESIAN_POINT('Ctrl Pts',(-0.294105065494125,0.00860322205134901,
-1.24348159858318));
#83224=CARTESIAN_POINT('Ctrl Pts',(-0.294198862422386,0.00434117925284497,
-1.24324960514607));
#83225=CARTESIAN_POINT('Ctrl Pts',(-0.294199989715657,7.77901478423249E-5,
-1.24301761170896));
#83226=CARTESIAN_POINT('',(-0.294199926066577,0.000208572338548644,-1.14301761549734));
#83227=CARTESIAN_POINT('Ctrl Pts',(-0.29419998971568,7.7790063860881E-5,
-1.24301761170439));
#83228=CARTESIAN_POINT('Ctrl Pts',(-0.294204324649468,-0.0163168162983833,
-1.24212549489629));
#83229=CARTESIAN_POINT('Ctrl Pts',(-0.292833941317543,-0.0327664949589083,
-1.24123337808819));
#83230=CARTESIAN_POINT('Ctrl Pts',(-0.290087364073985,-0.049020008206928,
-1.2403412612801));
#83231=CARTESIAN_POINT('Ctrl Pts',(-0.287345972973171,-0.0652428312422471,
-1.23945082898501));
#83232=CARTESIAN_POINT('Ctrl Pts',(-0.283233611214606,-0.0812694299995112,
-1.23856039668993));
#83233=CARTESIAN_POINT('Ctrl Pts',(-0.277800605409854,-0.0968527936299139,
-1.23766996439484));
#83234=CARTESIAN_POINT('Ctrl Pts',(-0.272368270947906,-0.112434231663436,
-1.23677964212823));
#83235=CARTESIAN_POINT('Ctrl Pts',(-0.265615832979466,-0.127571770699677,
-1.23588931986161));
#83236=CARTESIAN_POINT('Ctrl Pts',(-0.257643608018651,-0.142033134328338,
-1.234998997595));
#83237=CARTESIAN_POINT('Ctrl Pts',(-0.249672686289359,-0.156492133936285,
-1.23410882087069));
#83238=CARTESIAN_POINT('Ctrl Pts',(-0.240482776121732,-0.170274482609805,
-1.23321864414639));
#83239=CARTESIAN_POINT('Ctrl Pts',(-0.230219515778441,-0.183173727796156,
-1.23232846742209));
#83240=CARTESIAN_POINT('Ctrl Pts',(-0.21993289399697,-0.196102334502035,
-1.23143626445974));
#83241=CARTESIAN_POINT('Ctrl Pts',(-0.208568576975701,-0.208143220205496,
-1.2305440614974));
#83242=CARTESIAN_POINT('Ctrl Pts',(-0.196311668216858,-0.219124094799988,
-1.22965185853506));
#83243=CARTESIAN_POINT('Ctrl Pts',(-0.188102932771615,-0.226478240635376,
-1.22905432956381));
#83244=CARTESIAN_POINT('Ctrl Pts',(-0.179494641423396,-0.233357703304351,
-1.22845680059256));
#83245=CARTESIAN_POINT('Ctrl Pts',(-0.170549960397698,-0.239721402899999,
-1.22785927162131));
#83246=CARTESIAN_POINT('Ctrl Pts',(-0.157102258724431,-0.249288779696857,
-1.22696092864817));
#83247=CARTESIAN_POINT('Ctrl Pts',(-0.14280424939101,-0.257751478428811,
-1.22606258567502));
#83248=CARTESIAN_POINT('Ctrl Pts',(-0.12786272044659,-0.264961817475645,
-1.22516424270188));
#83249=CARTESIAN_POINT('Ctrl Pts',(-0.112950120925454,-0.272158196040184,
-1.22426763907845));
#83250=CARTESIAN_POINT('Ctrl Pts',(-0.0973971506760092,-0.278106629008214,
-1.22337103545502));
#83251=CARTESIAN_POINT('Ctrl Pts',(-0.0814370536116031,-0.282704167459662,
-1.22247443183159));
#83252=CARTESIAN_POINT('Ctrl Pts',(-0.0654796968465792,-0.287300916527955,
-1.22157798215223));
#83253=CARTESIAN_POINT('Ctrl Pts',(-0.0491160952757681,-0.290546962713943,
-1.22068153247288));
#83254=CARTESIAN_POINT('Ctrl Pts',(-0.0325965117074827,-0.292388623965612,
-1.21978508279352));
#83255=CARTESIAN_POINT('Ctrl Pts',(-0.0160812793908451,-0.29422980012445,
-1.21888886923865));
#83256=CARTESIAN_POINT('Ctrl Pts',(0.000589065745059934,-0.294667248985264,
-1.21799265568378));
#83257=CARTESIAN_POINT('Ctrl Pts',(0.0171588419832219,-0.293699189889579,
-1.21709644212891));
#83258=CARTESIAN_POINT('Ctrl Pts',(0.0337681546013056,-0.292728820952672,
-1.21619809016015));
#83259=CARTESIAN_POINT('Ctrl Pts',(0.0502756275678593,-0.29034631909139,
-1.21529973819139));
#83260=CARTESIAN_POINT('Ctrl Pts',(0.0664299975163362,-0.286601980854947,
-1.21440138622263));
#83261=CARTESIAN_POINT('Ctrl Pts',(0.0807944110567974,-0.28327252739838,
-1.21360257455587));
#83262=CARTESIAN_POINT('Ctrl Pts',(0.0948793846356908,-0.278867183381866,
-1.2128037628891));
#83263=CARTESIAN_POINT('Ctrl Pts',(0.108519805313765,-0.273454003179077,
-1.21200495122233));
#83264=CARTESIAN_POINT('Ctrl Pts',(0.123859811631003,-0.267366344999985,
-1.21110660825303));
#83265=CARTESIAN_POINT('Ctrl Pts',(0.138734734387574,-0.259964520171745,
-1.21020826528372));
#83266=CARTESIAN_POINT('Ctrl Pts',(0.152908215344758,-0.25134183432147,
-1.20930992231442));
#83267=CARTESIAN_POINT('Ctrl Pts',(0.167054253949881,-0.242735843507617,
-1.20841331869511));
#83268=CARTESIAN_POINT('Ctrl Pts',(0.180500844368606,-0.232914034008152,
-1.2075167150758));
#83269=CARTESIAN_POINT('Ctrl Pts',(0.193034796828567,-0.222016231869099,
-1.20662011145649));
#83270=CARTESIAN_POINT('Ctrl Pts',(0.205566597242393,-0.211120300853545,
-1.20572366178162));
#83271=CARTESIAN_POINT('Ctrl Pts',(0.217185441152932,-0.199149221706712,
-1.20482721210676));
#83272=CARTESIAN_POINT('Ctrl Pts',(0.22771024248155,-0.186283884082853,
-1.20393076243189));
#83273=CARTESIAN_POINT('Ctrl Pts',(0.238232271579244,-0.173421935186789,
-1.20303454888172));
#83274=CARTESIAN_POINT('Ctrl Pts',(0.247660337680816,-0.159666814838694,
-1.20213833533156));
#83275=CARTESIAN_POINT('Ctrl Pts',(0.255853974761835,-0.145232171362169,
-1.20124212178139));
#83276=CARTESIAN_POINT('Ctrl Pts',(0.264067162300656,-0.130763086051645,
-1.20034376981759));
#83277=CARTESIAN_POINT('Ctrl Pts',(0.271039669204752,-0.115611943382271,
-1.19944541785379));
#83278=CARTESIAN_POINT('Ctrl Pts',(0.276677143951878,-0.10001698863009,
-1.19854706589));
#83279=CARTESIAN_POINT('Ctrl Pts',(0.281689968440806,-0.0861500048133908,
-1.19774825420111));
#83280=CARTESIAN_POINT('Ctrl Pts',(0.285647818470339,-0.0719327978885206,
-1.19694944251223));
#83281=CARTESIAN_POINT('Ctrl Pts',(0.288518073790726,-0.0575409514701437,
-1.19615063082334));
#83282=CARTESIAN_POINT('Ctrl Pts',(0.291745960613989,-0.0413558925709045,
-1.19525228784092));
#83283=CARTESIAN_POINT('Ctrl Pts',(0.293617963536819,-0.0248469267792773,
-1.1943539448585));
#83284=CARTESIAN_POINT('Ctrl Pts',(0.29408393377337,-0.00826316503406248,
-1.19345560187609));
#83285=CARTESIAN_POINT('Ctrl Pts',(0.294549001809768,0.00828848763804503,
-1.19255899824334));
#83286=CARTESIAN_POINT('Ctrl Pts',(0.293613353229563,0.024913869004309,
-1.19166239461059));
#83287=CARTESIAN_POINT('Ctrl Pts',(0.291278480747702,0.04135803009466,-1.19076579097784));
#83288=CARTESIAN_POINT('Ctrl Pts',(0.288944009156409,0.0577993677721069,
-1.18986934128923));
#83289=CARTESIAN_POINT('Ctrl Pts',(0.285210849393363,0.0740587587732578,
-1.18897289160062));
#83290=CARTESIAN_POINT('Ctrl Pts',(0.280132411880159,0.0898858821740374,
-1.18807644191201));
#83291=CARTESIAN_POINT('Ctrl Pts',(0.275055312025453,0.105708836716569,
-1.18718022834791));
#83292=CARTESIAN_POINT('Ctrl Pts',(0.268633890113283,0.121098999628384,
-1.18628401478381));
#83293=CARTESIAN_POINT('Ctrl Pts',(0.260971132125323,0.135822340567474,
-1.1853878012197));
#83294=CARTESIAN_POINT('Ctrl Pts',(0.253290090385631,0.15058081218808,-1.18448944924195));
#83295=CARTESIAN_POINT('Ctrl Pts',(0.244362187410983,0.164668591742709,
-1.18359109726419));
#83296=CARTESIAN_POINT('Ctrl Pts',(0.234336120307431,0.177876987604527,
-1.18269274528643));
#83297=CARTESIAN_POINT('Ctrl Pts',(0.225420974450966,0.189621849714649,
-1.18189393366574));
#83298=CARTESIAN_POINT('Ctrl Pts',(0.215638442611246,0.200671536696332,
-1.18109512204505));
#83299=CARTESIAN_POINT('Ctrl Pts',(0.205118177365467,0.210903232109584,
-1.18029631042436));
#83300=CARTESIAN_POINT('Ctrl Pts',(0.193287094611401,0.222409789436847,
-1.17939796744835));
#83301=CARTESIAN_POINT('Ctrl Pts',(0.180447161138358,0.232954288037526,
-1.17849962447234));
#83302=CARTESIAN_POINT('Ctrl Pts',(0.166780220179905,0.242359233693999,
-1.17760128149633));
#83303=CARTESIAN_POINT('Ctrl Pts',(0.153139740819474,0.25174596972389,-1.1767046778701));
#83304=CARTESIAN_POINT('Ctrl Pts',(0.138676039276032,0.259997034964698,
-1.17580807424387));
#83305=CARTESIAN_POINT('Ctrl Pts',(0.123603927998681,0.266975109295411,
-1.17491147061763));
#83306=CARTESIAN_POINT('Ctrl Pts',(0.108534404558633,0.273951985511228,
-1.17401502093561));
#83307=CARTESIAN_POINT('Ctrl Pts',(0.0928573723032582,0.27965592568008,
-1.1731185712536));
#83308=CARTESIAN_POINT('Ctrl Pts',(0.0768119779240554,0.283995704276305,
-1.17222212157158));
#83309=CARTESIAN_POINT('Ctrl Pts',(0.0607708098965294,0.288334339776255,
-1.17132590801411));
#83310=CARTESIAN_POINT('Ctrl Pts',(0.044362239060206,0.291309331073124,
-1.17042969445665));
#83311=CARTESIAN_POINT('Ctrl Pts',(0.0278386839225503,0.292879920236025,
-1.16953348089918));
#83312=CARTESIAN_POINT('Ctrl Pts',(0.0112757026943745,0.294454256909071,
-1.16863512892801));
#83313=CARTESIAN_POINT('Ctrl Pts',(-0.0054020174295768,0.294617450173523,
-1.16773677695684));
#83314=CARTESIAN_POINT('Ctrl Pts',(-0.0219384814675519,0.293380883887989,
-1.16683842498566));
#83315=CARTESIAN_POINT('Ctrl Pts',(-0.0366426515522562,0.292281333165311,
-1.16603961333223));
#83316=CARTESIAN_POINT('Ctrl Pts',(-0.0512347525468744,0.290075858562765,
-1.1652408016788));
#83317=CARTESIAN_POINT('Ctrl Pts',(-0.0655412233709042,0.28680653416379,
-1.16444199002537));
#83318=CARTESIAN_POINT('Ctrl Pts',(-0.0816302695457364,0.283129854438748,
-1.16354364704931));
#83319=CARTESIAN_POINT('Ctrl Pts',(-0.0974601184399902,0.278083447173002,
-1.16264530407324));
#83320=CARTESIAN_POINT('Ctrl Pts',(-0.112782945798443,0.271723475498576,
-1.16174696109718));
#83321=CARTESIAN_POINT('Ctrl Pts',(-0.128076105471513,0.265375817846509,
-1.16085035747092));
#83322=CARTESIAN_POINT('Ctrl Pts',(-0.142863444807933,0.257719883201405,
-1.15995375384466));
#83323=CARTESIAN_POINT('Ctrl Pts',(-0.156912941363351,0.248861344593132,
-1.1590571502184));
#83324=CARTESIAN_POINT('Ctrl Pts',(-0.17096002566075,0.240004326970377,
-1.1581607005364));
#83325=CARTESIAN_POINT('Ctrl Pts',(-0.184268823550014,0.229945491424742,
-1.1572642508544));
#83326=CARTESIAN_POINT('Ctrl Pts',(-0.196632777383233,0.218835990775182,
-1.1563678011724));
#83327=CARTESIAN_POINT('Ctrl Pts',(-0.208993474554697,0.207729416364784,
-1.15547158761497));
#83328=CARTESIAN_POINT('Ctrl Pts',(-0.220409240524934,0.195573263295305,
-1.15457537405755));
#83329=CARTESIAN_POINT('Ctrl Pts',(-0.230708665875729,0.18255725537442,
-1.15367916050012));
#83330=CARTESIAN_POINT('Ctrl Pts',(-0.241032666208446,0.169510190559731,
-1.15278080852903));
#83331=CARTESIAN_POINT('Ctrl Pts',(-0.250234533990658,0.155599812781374,
-1.15188245655793));
#83332=CARTESIAN_POINT('Ctrl Pts',(-0.25818468306756,0.141047188661468,
-1.15098410458684));
#83333=CARTESIAN_POINT('Ctrl Pts',(-0.26525392979255,0.128107042583133,
-1.15018529293336));
#83334=CARTESIAN_POINT('Ctrl Pts',(-0.271333964041315,0.114659860226817,
-1.14938648127987));
#83335=CARTESIAN_POINT('Ctrl Pts',(-0.276365766182724,0.100874195323859,
-1.14858766962639));
#83336=CARTESIAN_POINT('Ctrl Pts',(-0.282866466672747,0.0830641789377884,
-1.14755566654652));
#83337=CARTESIAN_POINT('Ctrl Pts',(-0.287651798522018,0.0645963176383724,
-1.14652366346665));
#83338=CARTESIAN_POINT('Ctrl Pts',(-0.290615313155387,0.0457862398499426,
-1.14549166038678));
#83339=CARTESIAN_POINT('Ctrl Pts',(-0.292983480581905,0.030754961445827,
-1.14466697875697));
#83340=CARTESIAN_POINT('Ctrl Pts',(-0.294189081238035,0.015505652370611,
-1.14384229712716));
#83341=CARTESIAN_POINT('Ctrl Pts',(-0.294199926066577,0.000208572338548644,
-1.14301761549734));
#83342=CARTESIAN_POINT('',(-0.293910006811105,-0.000218120950975208,-1.04301761170896));
#83343=CARTESIAN_POINT('Ctrl Pts',(-0.293887912717633,0.000208280940901665,
-1.14301761170896));
#83344=CARTESIAN_POINT('Ctrl Pts',(-0.29347111625565,-0.0633124552653269,
-1.13958952421511));
#83345=CARTESIAN_POINT('Ctrl Pts',(-0.242085158539587,-0.225371926112401,
-1.13087666325494));
#83346=CARTESIAN_POINT('Ctrl Pts',(0.0248432358882371,-0.346674479333956,
-1.11687902882842));
#83347=CARTESIAN_POINT('Ctrl Pts',(0.3044975180128,-0.167575781385358,-1.10102470842943));
#83348=CARTESIAN_POINT('Ctrl Pts',(0.306165446002828,0.164508664378986,
-1.08517038803045));
#83349=CARTESIAN_POINT('Ctrl Pts',(0.0283243105090556,0.346407439901074,
-1.06931606763146));
#83350=CARTESIAN_POINT('Ctrl Pts',(-0.240829917627408,0.227340704164944,
-1.05526514219097));
#83351=CARTESIAN_POINT('Ctrl Pts',(-0.29346455100378,0.0642778682396108,
-1.0464989902168));
#83352=CARTESIAN_POINT('Ctrl Pts',(-0.293910006811105,-0.000218120950975208,
-1.04301761170896));
#83353=CARTESIAN_POINT('',(-0.294664342707076,-6.04394989484003E-5,-0.943017611708961));
#83354=CARTESIAN_POINT('Ctrl Pts',(-0.293910006811105,-0.000218120950975208,
-1.04301761170896));
#83355=CARTESIAN_POINT('Ctrl Pts',(-0.294140758151515,-0.0336278009059762,
-1.04121421675047));
#83356=CARTESIAN_POINT('Ctrl Pts',(-0.273471204903555,-0.164666211870492,
-1.03412604832565));
#83357=CARTESIAN_POINT('Ctrl Pts',(-0.0808290374716516,-0.338034092489328,
-1.02175310643452));
#83358=CARTESIAN_POINT('Ctrl Pts',(0.23980855062429,-0.251579490481548,
-1.00589878603552));
#83359=CARTESIAN_POINT('Ctrl Pts',(0.341516588451039,0.0645507613917535,
-0.990044465636539));
#83360=CARTESIAN_POINT('Ctrl Pts',(0.131442277715391,0.321750382459031,
-0.97419014523755));
#83361=CARTESIAN_POINT('Ctrl Pts',(-0.194909829171702,0.28562474370573,
-0.958514527261694));
#83362=CARTESIAN_POINT('Ctrl Pts',(-0.294400112794844,0.0939112419462086,
-0.948123682752163));
#83363=CARTESIAN_POINT('Ctrl Pts',(-0.294664342707076,-6.04394989484003E-5,
-0.943017611708961));
#83364=CARTESIAN_POINT('',(-0.294199883530078,0.00026178404932804,-0.843017611708961));
#83365=CARTESIAN_POINT('Ctrl Pts',(-0.294664342707076,-6.04394989484003E-5,
-0.943017611708961));
#83366=CARTESIAN_POINT('Ctrl Pts',(-0.294673590233242,-0.00334926314386741,
-0.942838909285835));
#83367=CARTESIAN_POINT('Ctrl Pts',(-0.293135403529261,-0.103889734782347,
-0.93737543339637));
#83368=CARTESIAN_POINT('Ctrl Pts',(-0.178979626789081,-0.297937366199709,
-0.926627184040607));
#83369=CARTESIAN_POINT('Ctrl Pts',(0.152803789238326,-0.312172040672919,
-0.910772863641607));
#83370=CARTESIAN_POINT('Ctrl Pts',(0.345087321836773,-0.0414140228791957,
-0.894918543242629));
#83371=CARTESIAN_POINT('Ctrl Pts',(0.222328659415099,0.267152293993907,
-0.879064222843639));
#83372=CARTESIAN_POINT('Ctrl Pts',(-0.103401553816396,0.331826008100429,
-0.863209902444658));
#83373=CARTESIAN_POINT('Ctrl Pts',(-0.278720695596675,0.151254505853962,
-0.851194384871808));
#83374=CARTESIAN_POINT('Ctrl Pts',(-0.294314128361141,0.027011048903306,
-0.844463640765287));
#83375=CARTESIAN_POINT('Ctrl Pts',(-0.294082633309355,0.000262760320685067,
-0.843017670125095));
#83376=CARTESIAN_POINT('',(-0.294199973461913,-0.000124960031393308,-0.743017611706046));
#83377=CARTESIAN_POINT('Ctrl Pts',(-0.294199883530078,0.00026178404932804,
-0.843017611708961));
#83378=CARTESIAN_POINT('Ctrl Pts',(-0.294214504485591,-0.0161696349771595,
-0.842129701439759));
#83379=CARTESIAN_POINT('Ctrl Pts',(-0.292848235671175,-0.0326311939379088,
-0.841241791170558));
#83380=CARTESIAN_POINT('Ctrl Pts',(-0.290112361285408,-0.0488718510945222,
-0.840353880901356));
#83381=CARTESIAN_POINT('Ctrl Pts',(-0.287376021304854,-0.0651152721080342,
-0.83946581952639));
#83382=CARTESIAN_POINT('Ctrl Pts',(-0.283269711147539,-0.0811369162079659,
-0.838577758151423));
#83383=CARTESIAN_POINT('Ctrl Pts',(-0.277856351568672,-0.0966927499502755,
-0.837689696776457));
#83384=CARTESIAN_POINT('Ctrl Pts',(-0.27244232273868,-0.112250506853071,
-0.836801525610876));
#83385=CARTESIAN_POINT('Ctrl Pts',(-0.26572121935906,-0.127341588578431,
-0.835913354445295));
#83386=CARTESIAN_POINT('Ctrl Pts',(-0.257804613108441,-0.141740683856143,
-0.835025183279714));
#83387=CARTESIAN_POINT('Ctrl Pts',(-0.249870591876541,-0.15617145431976,
-0.834135058311741));
#83388=CARTESIAN_POINT('Ctrl Pts',(-0.240736264007773,-0.169906526785005,
-0.833244933343769));
#83389=CARTESIAN_POINT('Ctrl Pts',(-0.230557071075997,-0.182748671614481,
-0.832354808375797));
#83390=CARTESIAN_POINT('Ctrl Pts',(-0.227303439228586,-0.186853477534391,
-0.832070292799426));
#83391=CARTESIAN_POINT('Ctrl Pts',(-0.22394335567284,-0.190867321422932,
-0.831785777223056));
#83392=CARTESIAN_POINT('Ctrl Pts',(-0.220482689971872,-0.194784556427781,
-0.831501261646685));
#83393=CARTESIAN_POINT('Ctrl Pts',(-0.20955581992897,-0.207153020048383,
-0.830602918669694));
#83394=CARTESIAN_POINT('Ctrl Pts',(-0.19755022185266,-0.218638487290109,
-0.829704575692702));
#83395=CARTESIAN_POINT('Ctrl Pts',(-0.184633792939896,-0.229050218302947,
-0.82880623271571));
#83396=CARTESIAN_POINT('Ctrl Pts',(-0.171742372501976,-0.239441790375967,
-0.827909629088495));
#83397=CARTESIAN_POINT('Ctrl Pts',(-0.157944189321307,-0.248763210945512,
-0.827013025461279));
#83398=CARTESIAN_POINT('Ctrl Pts',(-0.143443054015968,-0.256861305483275,
-0.826116421834064));
#83399=CARTESIAN_POINT('Ctrl Pts',(-0.128944408513228,-0.264958009601846,
-0.825219972151074));
#83400=CARTESIAN_POINT('Ctrl Pts',(-0.113743713373344,-0.27183137425185,
-0.824323522468084));
#83401=CARTESIAN_POINT('Ctrl Pts',(-0.0980725302068118,-0.27737234688922,
-0.823427072785094));
#83402=CARTESIAN_POINT('Ctrl Pts',(-0.0824054748249273,-0.282911860036165,
-0.822530859226665));
#83403=CARTESIAN_POINT('Ctrl Pts',(-0.0662689271156775,-0.287119424498268,
-0.821634645668236));
#83404=CARTESIAN_POINT('Ctrl Pts',(-0.0499114997054081,-0.289935306917176,
-0.820738432109806));
#83405=CARTESIAN_POINT('Ctrl Pts',(-0.0335150425948892,-0.292757908182758,
-0.819840080137697));
#83406=CARTESIAN_POINT('Ctrl Pts',(-0.0168974405960642,-0.294182086879795,
-0.818941728165588));
#83407=CARTESIAN_POINT('Ctrl Pts',(-0.000314816413647557,-0.294199831561178,
-0.818043376193478));
#83408=CARTESIAN_POINT('Ctrl Pts',(0.0144303990168213,-0.294215610074088,
-0.817244564544886));
#83409=CARTESIAN_POINT('Ctrl Pts',(0.02914751516652,-0.293120156158774,
-0.816445752896294));
#83410=CARTESIAN_POINT('Ctrl Pts',(0.0436602857802432,-0.290942295731624,
-0.815646941247702));
#83411=CARTESIAN_POINT('Ctrl Pts',(0.0599813366568894,-0.288493075539295,
-0.81474859827071));
#83412=CARTESIAN_POINT('Ctrl Pts',(0.0761475348421451,-0.284658446591712,
-0.813850255293718));
#83413=CARTESIAN_POINT('Ctrl Pts',(0.0919075179817019,-0.27947566645138,
-0.812951912316726));
#83414=CARTESIAN_POINT('Ctrl Pts',(0.107636987026026,-0.274302921083635,
-0.812055308689511));
#83415=CARTESIAN_POINT('Ctrl Pts',(0.12296103885853,-0.267787387647584,
-0.811158705062295));
#83416=CARTESIAN_POINT('Ctrl Pts',(0.137640322889568,-0.260016886980164,
-0.81026210143508));
#83417=CARTESIAN_POINT('Ctrl Pts',(0.152317086530392,-0.252247720485024,
-0.80936565175209));
#83418=CARTESIAN_POINT('Ctrl Pts',(0.166348580559642,-0.243224336992414,
-0.8084692020691));
#83419=CARTESIAN_POINT('Ctrl Pts',(0.179517406282843,-0.233081832928868,
-0.80757275238611));
#83420=CARTESIAN_POINT('Ctrl Pts',(0.19268276334155,-0.222942000397656,
-0.80667653882768));
#83421=CARTESIAN_POINT('Ctrl Pts',(0.204985283023187,-0.211684124036696,
-0.805780325269251));
#83422=CARTESIAN_POINT('Ctrl Pts',(0.216239696783704,-0.199484419278528,
-0.804884111710821));
#83423=CARTESIAN_POINT('Ctrl Pts',(0.227520964179854,-0.187255605369643,
-0.803985759738711));
#83424=CARTESIAN_POINT('Ctrl Pts',(0.237748611876534,-0.174081076772951,
-0.803087407766602));
#83425=CARTESIAN_POINT('Ctrl Pts',(0.246776704110147,-0.160171465338034,
-0.802189055794492));
#83426=CARTESIAN_POINT('Ctrl Pts',(0.254804454329073,-0.14780308413939,
-0.8013902441459));
#83427=CARTESIAN_POINT('Ctrl Pts',(0.261884176472585,-0.134854298041266,
-0.800591432497308));
#83428=CARTESIAN_POINT('Ctrl Pts',(0.267944271076834,-0.121488713867191,
-0.799792620848715));
#83429=CARTESIAN_POINT('Ctrl Pts',(0.274759448894066,-0.106457787994576,
-0.798894277871724));
#83430=CARTESIAN_POINT('Ctrl Pts',(0.280327563692435,-0.0908038287342872,
-0.797995934894732));
#83431=CARTESIAN_POINT('Ctrl Pts',(0.284543265378996,-0.0747580773392285,
-0.79709759191774));
#83432=CARTESIAN_POINT('Ctrl Pts',(0.288750804726704,-0.0587433933369265,
-0.796200988290524));
#83433=CARTESIAN_POINT('Ctrl Pts',(0.29161086635382,-0.0423391625408519,
-0.795304384663309));
#83434=CARTESIAN_POINT('Ctrl Pts',(0.293067071160927,-0.0257940264626506,
-0.794407781036093));
#83435=CARTESIAN_POINT('Ctrl Pts',(0.294523025941919,-0.00925173113602084,
-0.793511331353103));
#83436=CARTESIAN_POINT('Ctrl Pts',(0.294575480890083,0.0074306404827253,
-0.792614881670114));
#83437=CARTESIAN_POINT('Ctrl Pts',(0.293219671041644,0.0239971772137955,
-0.791718431987124));
#83438=CARTESIAN_POINT('Ctrl Pts',(0.291864218313086,0.0405593503243735,
-0.790822218428694));
#83439=CARTESIAN_POINT('Ctrl Pts',(0.289101312695973,0.0570049613871002,
-0.789926004870265));
#83440=CARTESIAN_POINT('Ctrl Pts',(0.284978167813586,0.0730827193638239,
-0.789029791311836));
#83441=CARTESIAN_POINT('Ctrl Pts',(0.280845184886083,0.0891988397345135,
-0.788131439339727));
#83442=CARTESIAN_POINT('Ctrl Pts',(0.275345703668974,0.104944591145454,
-0.787233087367617));
#83443=CARTESIAN_POINT('Ctrl Pts',(0.268577205164191,0.120082991577459,
-0.786334735395508));
#83444=CARTESIAN_POINT('Ctrl Pts',(0.262558678331769,0.133544007951413,
-0.785535923746915));
#83445=CARTESIAN_POINT('Ctrl Pts',(0.255537682367956,0.146524729915943,
-0.784737112098323));
#83446=CARTESIAN_POINT('Ctrl Pts',(0.247612630236219,0.158876132088812,
-0.783938300449731));
#83447=CARTESIAN_POINT('Ctrl Pts',(0.238700122591408,0.172766509648471,
-0.783039957472739));
#83448=CARTESIAN_POINT('Ctrl Pts',(0.228586828719118,0.185948756421437,
-0.782141614495747));
#83449=CARTESIAN_POINT('Ctrl Pts',(0.217409588544599,0.198208755631198,
-0.781243271518755));
#83450=CARTESIAN_POINT('Ctrl Pts',(0.206253989470077,0.21044501732931,-0.78034666789154));
#83451=CARTESIAN_POINT('Ctrl Pts',(0.19403901135192,0.2217619537564,-0.779450064264324));
#83452=CARTESIAN_POINT('Ctrl Pts',(0.18094271701787,0.231977096193118,-0.778553460637108));
#83453=CARTESIAN_POINT('Ctrl Pts',(0.16784867127933,0.242190484719696,-0.777657010954118));
#83454=CARTESIAN_POINT('Ctrl Pts',(0.153874199203373,0.251301928323536,
-0.776760561271128));
#83455=CARTESIAN_POINT('Ctrl Pts',(0.139231519657763,0.25916833127099,-0.775864111588138));
#83456=CARTESIAN_POINT('Ctrl Pts',(0.12459269698927,0.26703266221042,-0.774967898029708));
#83457=CARTESIAN_POINT('Ctrl Pts',(0.109286718519198,0.273652238764066,
-0.774071684471278));
#83458=CARTESIAN_POINT('Ctrl Pts',(0.0935501770825538,0.278930106599884,
-0.773175470912849));
#83459=CARTESIAN_POINT('Ctrl Pts',(0.0777760874129412,0.284220567711797,
-0.772277118940739));
#83460=CARTESIAN_POINT('Ctrl Pts',(0.0615701445870226,0.28816269889627,
-0.771378766968629));
#83461=CARTESIAN_POINT('Ctrl Pts',(0.045184252581767,0.290709517076113,
-0.77048041499652));
#83462=CARTESIAN_POINT('Ctrl Pts',(0.0306139707626918,0.292974139509263,
-0.769681603347928));
#83463=CARTESIAN_POINT('Ctrl Pts',(0.0159019676247145,0.294136245662769,
-0.768882791699337));
#83464=CARTESIAN_POINT('Ctrl Pts',(0.00122682394808608,0.294197442040206,
-0.768083980050745));
#83465=CARTESIAN_POINT('Ctrl Pts',(-0.0152768315525506,0.294266263440075,
-0.767185637073753));
#83466=CARTESIAN_POINT('Ctrl Pts',(-0.0318387570596783,0.292942267055195,
-0.766287294096761));
#83467=CARTESIAN_POINT('Ctrl Pts',(-0.0482048485476907,0.290223935223293,
-0.765388951119769));
#83468=CARTESIAN_POINT('Ctrl Pts',(-0.0645392524082683,0.287510866559228,
-0.764492347492553));
#83469=CARTESIAN_POINT('Ctrl Pts',(-0.0806777927326734,0.283408884511531,
-0.763595743865337));
#83470=CARTESIAN_POINT('Ctrl Pts',(-0.0963705245024942,0.277968275181025,
-0.762699140238121));
#83471=CARTESIAN_POINT('Ctrl Pts',(-0.112060561876071,0.272528599987262,
-0.761802690555131));
#83472=CARTESIAN_POINT('Ctrl Pts',(-0.12730418032624,0.265750962427366,
-0.760906240872141));
#83473=CARTESIAN_POINT('Ctrl Pts',(-0.141865919124776,0.257735719276321,
-0.76000979118915));
#83474=CARTESIAN_POINT('Ctrl Pts',(-0.156423822365954,0.249722587337767,
-0.759113577630721));
#83475=CARTESIAN_POINT('Ctrl Pts',(-0.170299514631689,0.240472888163074,
-0.758217364072292));
#83476=CARTESIAN_POINT('Ctrl Pts',(-0.183283017687103,0.23013251710158,
-0.757321150513862));
#83477=CARTESIAN_POINT('Ctrl Pts',(-0.196297500078069,0.219767473359417,
-0.756422798541753));
#83478=CARTESIAN_POINT('Ctrl Pts',(-0.208414936754856,0.208307075917067,
-0.755524446569643));
#83479=CARTESIAN_POINT('Ctrl Pts',(-0.219458972650302,0.19593723312141,
-0.754626094597533));
#83480=CARTESIAN_POINT('Ctrl Pts',(-0.229279293409457,0.184938009183379,
-0.753827282948942));
#83481=CARTESIAN_POINT('Ctrl Pts',(-0.238251205363472,0.173220572478498,
-0.753028471300351));
#83482=CARTESIAN_POINT('Ctrl Pts',(-0.246278992508625,0.160935694763271,
-0.752229659651761));
#83483=CARTESIAN_POINT('Ctrl Pts',(-0.255487172745188,0.146844468110076,
-0.751313392005111));
#83484=CARTESIAN_POINT('Ctrl Pts',(-0.263509256906277,0.131919432687266,
-0.750397124358462));
#83485=CARTESIAN_POINT('Ctrl Pts',(-0.270201849148427,0.116381273050137,
-0.749480856711813));
#83486=CARTESIAN_POINT('Ctrl Pts',(-0.276879016293115,0.100878925788558,
-0.748566700880322));
#83487=CARTESIAN_POINT('Ctrl Pts',(-0.28223242070145,0.0847669120513509,
-0.747652545048832));
#83488=CARTESIAN_POINT('Ctrl Pts',(-0.286164346184093,0.0682906067701156,
-0.746738389217342));
#83489=CARTESIAN_POINT('Ctrl Pts',(-0.290089851922504,0.0518412027275383,
-0.745825725948885));
#83490=CARTESIAN_POINT('Ctrl Pts',(-0.292598275702172,0.0350294021982569,
-0.744913062680429));
#83491=CARTESIAN_POINT('Ctrl Pts',(-0.29364173715284,0.0181154685797119,
-0.744000399411972));
#83492=CARTESIAN_POINT('Ctrl Pts',(-0.29401628240508,0.01204429697153,-0.743672803510968));
#83493=CARTESIAN_POINT('Ctrl Pts',(-0.294202558046068,0.00596006500085705,
-0.743345207609965));
#83494=CARTESIAN_POINT('Ctrl Pts',(-0.294199973461936,-0.000124959977242106,
-0.743017611708961));
#83495=CARTESIAN_POINT('',(-0.29419994452424,-0.000180670788710602,-0.643017611712501));
#83496=CARTESIAN_POINT('Ctrl Pts',(-0.294199973461913,-0.000124960031394621,
-0.743017611706046));
#83497=CARTESIAN_POINT('Ctrl Pts',(-0.294192255021624,-0.0182968899125074,
-0.742039300234221));
#83498=CARTESIAN_POINT('Ctrl Pts',(-0.292496705742507,-0.0364142011968275,
-0.741060988762396));
#83499=CARTESIAN_POINT('Ctrl Pts',(-0.289168196490808,-0.0541792777568467,
-0.740082677290572));
#83500=CARTESIAN_POINT('Ctrl Pts',(-0.28581688854588,-0.0720660365776137,
-0.739097664854008));
#83501=CARTESIAN_POINT('Ctrl Pts',(-0.280810398565039,-0.0895952168965191,
-0.738112652417445));
#83502=CARTESIAN_POINT('Ctrl Pts',(-0.274254017629792,-0.106481800388225,
-0.737127639980882));
#83503=CARTESIAN_POINT('Ctrl Pts',(-0.272584877908559,-0.110780828699772,
-0.736876873071513));
#83504=CARTESIAN_POINT('Ctrl Pts',(-0.270815523574129,-0.115038324182596,
-0.736626106162144));
#83505=CARTESIAN_POINT('Ctrl Pts',(-0.268948167693537,-0.11924983477678,
-0.736375339252776));
#83506=CARTESIAN_POINT('Ctrl Pts',(-0.262258584745376,-0.134337076448095,
-0.735476996275783));
#83507=CARTESIAN_POINT('Ctrl Pts',(-0.254274257069447,-0.148907623949626,
-0.734578653298791));
#83508=CARTESIAN_POINT('Ctrl Pts',(-0.245097765117353,-0.162728994142036,
-0.733680310321798));
#83509=CARTESIAN_POINT('Ctrl Pts',(-0.235939040465313,-0.176523603734355,
-0.732783706694582));
#83510=CARTESIAN_POINT('Ctrl Pts',(-0.225593111081812,-0.189571227491716,
-0.731887103067366));
#83511=CARTESIAN_POINT('Ctrl Pts',(-0.21420812514189,-0.201664372468704,
-0.73099049944015));
#83512=CARTESIAN_POINT('Ctrl Pts',(-0.20282509397082,-0.213755441088002,
-0.73009404975716));
#83513=CARTESIAN_POINT('Ctrl Pts',(-0.190403862688639,-0.224891746030959,
-0.729197600074169));
#83514=CARTESIAN_POINT('Ctrl Pts',(-0.177132341269818,-0.234899496968965,
-0.728301150391179));
#83515=CARTESIAN_POINT('Ctrl Pts',(-0.163864315565505,-0.244904611868566,
-0.727404936832749));
#83516=CARTESIAN_POINT('Ctrl Pts',(-0.149747082751248,-0.253781295277588,
-0.726508723274319));
#83517=CARTESIAN_POINT('Ctrl Pts',(-0.134999679343011,-0.261397640726316,
-0.725612509715889));
#83518=CARTESIAN_POINT('Ctrl Pts',(-0.120217087838255,-0.269032159184309,
-0.724714157743779));
#83519=CARTESIAN_POINT('Ctrl Pts',(-0.10480204073917,-0.275399992731581,
-0.723815805771669));
#83520=CARTESIAN_POINT('Ctrl Pts',(-0.0889963284700256,-0.280416286115581,
-0.722917453799559));
#83521=CARTESIAN_POINT('Ctrl Pts',(-0.0749419405832901,-0.284876757859713,
-0.72211864215097));
#83522=CARTESIAN_POINT('Ctrl Pts',(-0.0605793272098095,-0.288269229543724,
-0.72131983050238));
#83523=CARTESIAN_POINT('Ctrl Pts',(-0.0460852246718732,-0.290568050664458,
-0.72052101885379));
#83524=CARTESIAN_POINT('Ctrl Pts',(-0.0297851678991138,-0.293153303161486,
-0.719622675876799));
#83525=CARTESIAN_POINT('Ctrl Pts',(-0.013215082003028,-0.294370922283767,
-0.718724332899807));
#83526=CARTESIAN_POINT('Ctrl Pts',(0.00337413362794727,-0.294180650659184,
-0.717825989922815));
#83527=CARTESIAN_POINT('Ctrl Pts',(0.0199312296239529,-0.293990747433883,
-0.7169293862956));
#83528=CARTESIAN_POINT('Ctrl Pts',(0.0365065991775859,-0.292398307581924,
-0.716032782668384));
#83529=CARTESIAN_POINT('Ctrl Pts',(0.0528455518248773,-0.289414905718977,
-0.715136179041169));
#83530=CARTESIAN_POINT('Ctrl Pts',(0.0691816991216972,-0.28643201609742,
-0.714239729358179));
#83531=CARTESIAN_POINT('Ctrl Pts',(0.0852807248679252,-0.282058728504559,
-0.713343279675189));
#83532=CARTESIAN_POINT('Ctrl Pts',(0.100894616336768,-0.276358311606972,
-0.712446829992199));
#83533=CARTESIAN_POINT('Ctrl Pts',(0.116504395111576,-0.270659396197379,
-0.711550616433769));
#83534=CARTESIAN_POINT('Ctrl Pts',(0.131628553785732,-0.263634327153267,
-0.71065440287534));
#83535=CARTESIAN_POINT('Ctrl Pts',(0.14603731815087,-0.255395265632121,
-0.70975818931691));
#83536=CARTESIAN_POINT('Ctrl Pts',(0.160480462601583,-0.247136545267719,
-0.708859837344801));
#83537=CARTESIAN_POINT('Ctrl Pts',(0.174204127161342,-0.237658464649597,
-0.707961485372691));
#83538=CARTESIAN_POINT('Ctrl Pts',(0.187005664358342,-0.227117858165964,
-0.707063133400582));
#83539=CARTESIAN_POINT('Ctrl Pts',(0.198388749552488,-0.21774518520062,
-0.706264321751989));
#83540=CARTESIAN_POINT('Ctrl Pts',(0.20904289889353,-0.207533298554993,
-0.705465510103397));
#83541=CARTESIAN_POINT('Ctrl Pts',(0.218850519695666,-0.19661660669673,
-0.704666698454805));
#83542=CARTESIAN_POINT('Ctrl Pts',(0.229880162646069,-0.184339703273834,
-0.703768355477813));
#83543=CARTESIAN_POINT('Ctrl Pts',(0.239908600155231,-0.17109278725329,
-0.702870012500821));
#83544=CARTESIAN_POINT('Ctrl Pts',(0.248765668658983,-0.157064579382651,
-0.70197166952383));
#83545=CARTESIAN_POINT('Ctrl Pts',(0.257605588322575,-0.143063532586175,
-0.701075065896615));
#83546=CARTESIAN_POINT('Ctrl Pts',(0.26527816780488,-0.12828482274366,-0.700178462269399));
#83547=CARTESIAN_POINT('Ctrl Pts',(0.271654690118552,-0.112948525163427,
-0.699281858642184));
#83548=CARTESIAN_POINT('Ctrl Pts',(0.278030117601958,-0.0976148607807189,
-0.698385408959195));
#83549=CARTESIAN_POINT('Ctrl Pts',(0.283109578367738,-0.0817245067042235,
-0.697488959276205));
#83550=CARTESIAN_POINT('Ctrl Pts',(0.286811376364256,-0.0655200304337614,
-0.696592509593215));
#83551=CARTESIAN_POINT('Ctrl Pts',(0.290512199308362,-0.0493198224171825,
-0.695696296034786));
#83552=CARTESIAN_POINT('Ctrl Pts',(0.292835914388295,-0.0328064303094779,
-0.694800082476357));
#83553=CARTESIAN_POINT('Ctrl Pts',(0.293751778554187,-0.0162336870812481,
-0.693903868917928));
#83554=CARTESIAN_POINT('Ctrl Pts',(0.294669828021164,0.0003785996023382,
-0.693005516945819));
#83555=CARTESIAN_POINT('Ctrl Pts',(0.294173300279452,0.0170497255797299,
-0.692107164973709));
#83556=CARTESIAN_POINT('Ctrl Pts',(0.292283694721163,0.0335243463790987,
-0.6912088130016));
#83557=CARTESIAN_POINT('Ctrl Pts',(0.290603463611231,0.0481735255530376,
-0.690410001353007));
#83558=CARTESIAN_POINT('Ctrl Pts',(0.287822606151975,0.0626669847273044,
-0.689611189704414));
#83559=CARTESIAN_POINT('Ctrl Pts',(0.283990027738915,0.0768329626192458,
-0.688812378055821));
#83560=CARTESIAN_POINT('Ctrl Pts',(0.279679912948768,0.0927640106627477,
-0.687914035078829));
#83561=CARTESIAN_POINT('Ctrl Pts',(0.274011393354672,0.108381892354642,
-0.687015692101837));
#83562=CARTESIAN_POINT('Ctrl Pts',(0.267050389441296,0.123441198549156,
-0.686117349124845));
#83563=CARTESIAN_POINT('Ctrl Pts',(0.260102863254034,0.138471347282061,
-0.68522074549763));
#83564=CARTESIAN_POINT('Ctrl Pts',(0.251868088519605,0.152944329890869,
-0.684324141870414));
#83565=CARTESIAN_POINT('Ctrl Pts',(0.24246083193315,0.16663248476298,-0.683427538243199));
#83566=CARTESIAN_POINT('Ctrl Pts',(0.233055190545188,0.18031828941886,-0.682531088560209));
#83567=CARTESIAN_POINT('Ctrl Pts',(0.222477870275601,0.193218854145344,
-0.681634638877219));
#83568=CARTESIAN_POINT('Ctrl Pts',(0.21088807490934,0.205133760900133,-0.680738189194228));
#83569=CARTESIAN_POINT('Ctrl Pts',(0.199301332291482,0.217045529272281,
-0.679841975635799));
#83570=CARTESIAN_POINT('Ctrl Pts',(0.186703203618274,0.227971595563905,
-0.678945762077369));
#83571=CARTESIAN_POINT('Ctrl Pts',(0.173290043395749,0.237748187921379,
-0.67804954851894));
#83572=CARTESIAN_POINT('Ctrl Pts',(0.159844878652601,0.247548107753255,
-0.67715119654683));
#83573=CARTESIAN_POINT('Ctrl Pts',(0.145581456020645,0.256192629485234,
-0.676252844574721));
#83574=CARTESIAN_POINT('Ctrl Pts',(0.13072579421455,0.263561011393899,-0.675354492602611));
#83575=CARTESIAN_POINT('Ctrl Pts',(0.117516188106169,0.27011295259585,-0.674555680954019));
#83576=CARTESIAN_POINT('Ctrl Pts',(0.103839065152268,0.275656402311337,
-0.673756869305427));
#83577=CARTESIAN_POINT('Ctrl Pts',(0.0898651813964756,0.280139053279935,
-0.672958057656835));
#83578=CARTESIAN_POINT('Ctrl Pts',(0.0741501622734572,0.285180239175313,
-0.672059714679843));
#83579=CARTESIAN_POINT('Ctrl Pts',(0.0579596738832171,0.288910980203061,
-0.671161371702851));
#83580=CARTESIAN_POINT('Ctrl Pts',(0.0415355396605274,0.291253221347179,
-0.670263028725859));
#83581=CARTESIAN_POINT('Ctrl Pts',(0.0251432054462076,0.293590927501082,
-0.669366425098644));
#83582=CARTESIAN_POINT('Ctrl Pts',(0.00851888820143327,0.294545294656183,
-0.668469821471429));
#83583=CARTESIAN_POINT('Ctrl Pts',(-0.00808393619602547,0.294088915084501,
-0.667573217844213));
#83584=CARTESIAN_POINT('Ctrl Pts',(-0.0246839099370022,0.293632613871858,
-0.666676768161224));
#83585=CARTESIAN_POINT('Ctrl Pts',(-0.0412616084004215,0.291766015895987,
-0.665780318478234));
#83586=CARTESIAN_POINT('Ctrl Pts',(-0.0575622706264213,0.288513821159976,
-0.664883868795244));
#83587=CARTESIAN_POINT('Ctrl Pts',(-0.0738586392631893,0.285262483051021,
-0.663987655236814));
#83588=CARTESIAN_POINT('Ctrl Pts',(-0.0898773427086045,0.280626438335591,
-0.663091441678385));
#83589=CARTESIAN_POINT('Ctrl Pts',(-0.10537418774529,0.274681489287175,
-0.662195228119956));
#83590=CARTESIAN_POINT('Ctrl Pts',(-0.120908009086468,0.268722355271065,
-0.661296876147846));
#83591=CARTESIAN_POINT('Ctrl Pts',(-0.135916752965931,0.261448388793748,
-0.660398524175737));
#83592=CARTESIAN_POINT('Ctrl Pts',(-0.150176221676798,0.252983680190801,
-0.659500172203628));
#83593=CARTESIAN_POINT('Ctrl Pts',(-0.162855694826091,0.245456888861901,
-0.658701360555035));
#83594=CARTESIAN_POINT('Ctrl Pts',(-0.174942762960054,0.236989521445209,
-0.657902548906443));
#83595=CARTESIAN_POINT('Ctrl Pts',(-0.186300708506579,0.227696477816295,
-0.657103737257851));
#83596=CARTESIAN_POINT('Ctrl Pts',(-0.198905453671994,0.217383305748889,
-0.656217237386512));
#83597=CARTESIAN_POINT('Ctrl Pts',(-0.210696351313985,0.205983107096295,
-0.655330737515173));
#83598=CARTESIAN_POINT('Ctrl Pts',(-0.22147910828788,0.193650831632621,
-0.654444237643834));
#83599=CARTESIAN_POINT('Ctrl Pts',(-0.232240944388006,0.181342483442729,
-0.653559457773414));
#83600=CARTESIAN_POINT('Ctrl Pts',(-0.24199793812666,0.168106205160555,
-0.652674677902993));
#83601=CARTESIAN_POINT('Ctrl Pts',(-0.250591645736961,0.154134574599086,
-0.651789898032573));
#83602=CARTESIAN_POINT('Ctrl Pts',(-0.25918261293684,0.140167399390736,
-0.650905400305797));
#83603=CARTESIAN_POINT('Ctrl Pts',(-0.266610566372324,0.125466004264436,
-0.65002090257902));
#83604=CARTESIAN_POINT('Ctrl Pts',(-0.272760083063504,0.110252333704057,
-0.649136404852244));
#83605=CARTESIAN_POINT('Ctrl Pts',(-0.278908646488963,0.0950410214868358,
-0.648252044235651));
#83606=CARTESIAN_POINT('Ctrl Pts',(-0.283778880199586,0.0793183525715875,
-0.647367683619057));
#83607=CARTESIAN_POINT('Ctrl Pts',(-0.287303993989222,0.0633249953639239,
-0.646483323002464));
#83608=CARTESIAN_POINT('Ctrl Pts',(-0.290835491119008,0.0473026770942102,
-0.645597360969586));
#83609=CARTESIAN_POINT('Ctrl Pts',(-0.293016886047028,0.0310094971912828,
-0.644711398936707));
#83610=CARTESIAN_POINT('Ctrl Pts',(-0.293832794792137,0.0146945127391705,
-0.643825436903829));
#83611=CARTESIAN_POINT('Ctrl Pts',(-0.29408077819461,0.00973581437986222,
-0.643556161840053));
#83612=CARTESIAN_POINT('Ctrl Pts',(-0.294202987909769,0.00477510463055562,
-0.643286886776277));
#83613=CARTESIAN_POINT('Ctrl Pts',(-0.29419994452424,-0.000180670788711742,
-0.643017611712501));
#83614=CARTESIAN_POINT('',(-0.294199888424845,0.000256224137824597,-0.543017611708961));
#83615=CARTESIAN_POINT('Ctrl Pts',(-0.2941999445242,-0.000180670853884201,
-0.64301761170896));
#83616=CARTESIAN_POINT('Ctrl Pts',(-0.294193283057564,-0.011028038166241,
-0.642428213425595));
#83617=CARTESIAN_POINT('Ctrl Pts',(-0.293586727488202,-0.0218568137071715,
-0.64183881514223));
#83618=CARTESIAN_POINT('Ctrl Pts',(-0.292386214611939,-0.0326181162071238,
-0.641249416858865));
#83619=CARTESIAN_POINT('Ctrl Pts',(-0.290556429317991,-0.0490201669035152,
-0.640351073881873));
#83620=CARTESIAN_POINT('Ctrl Pts',(-0.287336367282512,-0.0653199074971147,
-0.639452730904881));
#83621=CARTESIAN_POINT('Ctrl Pts',(-0.282753746412743,-0.0812647456746065,
-0.638554387927889));
#83622=CARTESIAN_POINT('Ctrl Pts',(-0.278179998301807,-0.097178711845047,
-0.637657784300673));
#83623=CARTESIAN_POINT('Ctrl Pts',(-0.272249080833386,-0.112738369890925,
-0.636761180673457));
#83624=CARTESIAN_POINT('Ctrl Pts',(-0.265039693558183,-0.127701217059919,
-0.635864577046242));
#83625=CARTESIAN_POINT('Ctrl Pts',(-0.257831544113728,-0.142661495151736,
-0.634968127363251));
#83626=CARTESIAN_POINT('Ctrl Pts',(-0.249345655567605,-0.157024432522995,
-0.634071677680261));
#83627=CARTESIAN_POINT('Ctrl Pts',(-0.239708799974846,-0.170567673416211,
-0.63317522799727));
#83628=CARTESIAN_POINT('Ctrl Pts',(-0.230074482726777,-0.184107347024094,
-0.63227901443884));
#83629=CARTESIAN_POINT('Ctrl Pts',(-0.219290268003284,-0.196827114454101,
-0.631382800880411));
#83630=CARTESIAN_POINT('Ctrl Pts',(-0.207525233393089,-0.208535170906838,
-0.630486587321981));
#83631=CARTESIAN_POINT('Ctrl Pts',(-0.195732126778491,-0.220271163411035,
-0.629588235349871));
#83632=CARTESIAN_POINT('Ctrl Pts',(-0.182954108098386,-0.230990082188767,
-0.628689883377761));
#83633=CARTESIAN_POINT('Ctrl Pts',(-0.169396135275969,-0.240538124532402,
-0.627791531405651));
#83634=CARTESIAN_POINT('Ctrl Pts',(-0.157340429986674,-0.249028212696192,
-0.626992719757061));
#83635=CARTESIAN_POINT('Ctrl Pts',(-0.144668856891886,-0.256592917736481,
-0.626193908108471));
#83636=CARTESIAN_POINT('Ctrl Pts',(-0.131542195880845,-0.263154499681927,
-0.62539509645988));
#83637=CARTESIAN_POINT('Ctrl Pts',(-0.116779962816974,-0.270533649784523,
-0.624496753482888));
#83638=CARTESIAN_POINT('Ctrl Pts',(-0.101347946836035,-0.276690209350932,
-0.623598410505896));
#83639=CARTESIAN_POINT('Ctrl Pts',(-0.0854732364897492,-0.281510152292892,
-0.622700067528904));
#83640=CARTESIAN_POINT('Ctrl Pts',(-0.0696292623707145,-0.286320762978807,
-0.621803463901689));
#83641=CARTESIAN_POINT('Ctrl Pts',(-0.0533450244017,-0.289799603919447,
-0.620906860274473));
#83642=CARTESIAN_POINT('Ctrl Pts',(-0.0368668522651501,-0.291880926413597,
-0.620010256647257));
#83643=CARTESIAN_POINT('Ctrl Pts',(-0.0203915093826523,-0.29396189155075,
-0.619113806964267));
#83644=CARTESIAN_POINT('Ctrl Pts',(-0.00372307423914003,-0.294645663599207,
-0.618217357281277));
#83645=CARTESIAN_POINT('Ctrl Pts',(0.012882905653892,-0.293917795891833,
-0.617320907598286));
#83646=CARTESIAN_POINT('Ctrl Pts',(0.029484511537114,-0.29319011990458,
-0.616424694039857));
#83647=CARTESIAN_POINT('Ctrl Pts',(0.0460229048034565,-0.291051587968063,
-0.615528480481427));
#83648=CARTESIAN_POINT('Ctrl Pts',(0.0622451876113885,-0.287539869616759,
-0.614632266922998));
#83649=CARTESIAN_POINT('Ctrl Pts',(0.078506177657293,-0.284019772116878,
-0.613733914950888));
#83650=CARTESIAN_POINT('Ctrl Pts',(0.0944487800500677,-0.279120138447055,
-0.612835562978778));
#83651=CARTESIAN_POINT('Ctrl Pts',(0.10983249331608,-0.27292941104244,-0.611937211006669));
#83652=CARTESIAN_POINT('Ctrl Pts',(0.123511641063281,-0.267424636391091,
-0.611138399358077));
#83653=CARTESIAN_POINT('Ctrl Pts',(0.136748777549695,-0.260899933740103,
-0.610339587709486));
#83654=CARTESIAN_POINT('Ctrl Pts',(0.149391259655662,-0.253448005591866,
-0.609540776060895));
#83655=CARTESIAN_POINT('Ctrl Pts',(0.163608985488364,-0.245067572821736,
-0.608642433083903));
#83656=CARTESIAN_POINT('Ctrl Pts',(0.177164532338704,-0.235460414421937,
-0.607744090106912));
#83657=CARTESIAN_POINT('Ctrl Pts',(0.189838758032202,-0.22475516890339,
-0.60684574712992));
#83658=CARTESIAN_POINT('Ctrl Pts',(0.202488444198825,-0.214070650620292,
-0.605949143502705));
#83659=CARTESIAN_POINT('Ctrl Pts',(0.214259556556526,-0.202292719801003,
-0.605052539875489));
#83660=CARTESIAN_POINT('Ctrl Pts',(0.224963018208994,-0.189592406067068,
-0.604155936248274));
#83661=CARTESIAN_POINT('Ctrl Pts',(0.235664642108343,-0.176894272939925,
-0.603259486565284));
#83662=CARTESIAN_POINT('Ctrl Pts',(0.245298430800219,-0.163274640426973,
-0.602363036882294));
#83663=CARTESIAN_POINT('Ctrl Pts',(0.253713359510653,-0.148940159815337,
-0.601466587199305));
#83664=CARTESIAN_POINT('Ctrl Pts',(0.262126071731548,-0.134609454901324,
-0.600570373640875));
#83665=CARTESIAN_POINT('Ctrl Pts',(0.26932017023549,-0.119564963637371,
-0.599674160082446));
#83666=CARTESIAN_POINT('Ctrl Pts',(0.275189816146444,-0.104039440066191,
-0.598777946524017));
#83667=CARTESIAN_POINT('Ctrl Pts',(0.281073467347761,-0.0884768717619945,
-0.597879594551908));
#83668=CARTESIAN_POINT('Ctrl Pts',(0.285626098317954,-0.0724317313013547,
-0.596981242579798));
#83669=CARTESIAN_POINT('Ctrl Pts',(0.288791226176685,-0.056153964093078,
-0.596082890607689));
#83670=CARTESIAN_POINT('Ctrl Pts',(0.291605647563108,-0.0416798264913989,
-0.595284078959096));
#83671=CARTESIAN_POINT('Ctrl Pts',(0.293323706045839,-0.0270223436892772,
-0.594485267310503));
#83672=CARTESIAN_POINT('Ctrl Pts',(0.293940248477391,-0.01236002933045,
-0.593686455661911));
#83673=CARTESIAN_POINT('Ctrl Pts',(0.294633611630492,0.00412919832901943,
-0.59278811268492));
#83674=CARTESIAN_POINT('Ctrl Pts',(0.293937360080827,0.0207293663013482,
-0.591889769707929));
#83675=CARTESIAN_POINT('Ctrl Pts',(0.29184036052926,0.0371866100384445,
-0.590991426730939));
#83676=CARTESIAN_POINT('Ctrl Pts',(0.289747421137114,0.0536119896613369,
-0.590094823103724));
#83677=CARTESIAN_POINT('Ctrl Pts',(0.286259150804987,0.0698942103517408,
-0.58919821947651));
#83678=CARTESIAN_POINT('Ctrl Pts',(0.281416340284715,0.0857816030437603,
-0.588301615849295));
#83679=CARTESIAN_POINT('Ctrl Pts',(0.276574361260873,0.101666267916833,
-0.587405166166306));
#83680=CARTESIAN_POINT('Ctrl Pts',(0.270378483389427,0.117155469695785,
-0.586508716483318));
#83681=CARTESIAN_POINT('Ctrl Pts',(0.262920080392568,0.132010118272675,
-0.585612266800329));
#83682=CARTESIAN_POINT('Ctrl Pts',(0.25546364193668,0.146860854139867,-0.5847160532419));
#83683=CARTESIAN_POINT('Ctrl Pts',(0.246745703427356,0.161076666421359,
-0.583819839683472));
#83684=CARTESIAN_POINT('Ctrl Pts',(0.236904108937943,0.174442205811321,
-0.582923626125044));
#83685=CARTESIAN_POINT('Ctrl Pts',(0.22703903187555,0.187839636096043,-0.582025274152935));
#83686=CARTESIAN_POINT('Ctrl Pts',(0.216045436576349,0.20038211765071,-0.581126922180827));
#83687=CARTESIAN_POINT('Ctrl Pts',(0.204102423935433,0.211886385932841,
-0.580228570208718));
#83688=CARTESIAN_POINT('Ctrl Pts',(0.193482735981139,0.222115943831838,
-0.57942975856012));
#83689=CARTESIAN_POINT('Ctrl Pts',(0.182113241232746,0.231524881934175,
-0.578630946911523));
#83690=CARTESIAN_POINT('Ctrl Pts',(0.170140981002164,0.240011846756824,
-0.577832135262925));
#83691=CARTESIAN_POINT('Ctrl Pts',(0.156676986184649,0.24955628098961,-0.57693379228593));
#83692=CARTESIAN_POINT('Ctrl Pts',(0.142364568443402,0.257994588955791,
-0.576035449308936));
#83693=CARTESIAN_POINT('Ctrl Pts',(0.12741076732988,0.26517944182838,-0.575137106331942));
#83694=CARTESIAN_POINT('Ctrl Pts',(0.112485919401599,0.272350383563956,
-0.574240502704724));
#83695=CARTESIAN_POINT('Ctrl Pts',(0.0969228294530991,0.278272289657258,
-0.573343899077506));
#83696=CARTESIAN_POINT('Ctrl Pts',(0.0809549165910538,0.28284260902441,
-0.572447295450288));
#83697=CARTESIAN_POINT('Ctrl Pts',(0.064989745373034,0.287412143681069,
-0.571550845767296));
#83698=CARTESIAN_POINT('Ctrl Pts',(0.0486206329227484,0.290630284749886,
-0.570654396084304));
#83699=CARTESIAN_POINT('Ctrl Pts',(0.032097933215732,0.292443776961108,
-0.569757946401311));
#83700=CARTESIAN_POINT('Ctrl Pts',(0.0155795855825511,0.29425679149906,
-0.56886173284288));
#83701=CARTESIAN_POINT('Ctrl Pts',(-0.00109148125168673,0.294665816296967,
-0.567965519284448));
#83702=CARTESIAN_POINT('Ctrl Pts',(-0.0176595829037503,0.293669506642528,
-0.567069305726016));
#83703=CARTESIAN_POINT('Ctrl Pts',(-0.0342672169361189,0.292670819739748,
-0.566170953753905));
#83704=CARTESIAN_POINT('Ctrl Pts',(-0.0507706037386733,0.290260175593658,
-0.565272601781793));
#83705=CARTESIAN_POINT('Ctrl Pts',(-0.066918566065098,0.286488299090541,
-0.564374249809681));
#83706=CARTESIAN_POINT('Ctrl Pts',(-0.0812772815882203,0.283134358785145,
-0.563575438161101));
#83707=CARTESIAN_POINT('Ctrl Pts',(-0.0953547231456902,0.278705005984337,
-0.56277662651252));
#83708=CARTESIAN_POINT('Ctrl Pts',(-0.108985894084055,0.273268576478707,
-0.561977814863939));
#83709=CARTESIAN_POINT('Ctrl Pts',(-0.124315498631508,0.267154771960502,
-0.561079471886949));
#83710=CARTESIAN_POINT('Ctrl Pts',(-0.139177779585522,0.259727595661658,
-0.560181128909958));
#83711=CARTESIAN_POINT('Ctrl Pts',(-0.153336538137476,0.251080756076635,
-0.559282785932967));
#83712=CARTESIAN_POINT('Ctrl Pts',(-0.167467882846218,0.242450658291663,
-0.558386182305753));
#83713=CARTESIAN_POINT('Ctrl Pts',(-0.18089770736005,0.232605936149883,
-0.557489578678539));
#83714=CARTESIAN_POINT('Ctrl Pts',(-0.19341306062255,0.221686778993737,
-0.556592975051324));
#83715=CARTESIAN_POINT('Ctrl Pts',(-0.205926265035431,0.210769496624997,
-0.555696525368335));
#83716=CARTESIAN_POINT('Ctrl Pts',(-0.21752468109241,0.198778624291577,
-0.554800075685346));
#83717=CARTESIAN_POINT('Ctrl Pts',(-0.228027531399338,0.185895360146304,
-0.553903626002357));
#83718=CARTESIAN_POINT('Ctrl Pts',(-0.238527615258844,0.173015489448698,
-0.553007412443928));
#83719=CARTESIAN_POINT('Ctrl Pts',(-0.247932214807086,0.159244313826685,
-0.5521111988855));
#83720=CARTESIAN_POINT('Ctrl Pts',(-0.2561012284999,0.144795720796031,-0.551214985327071));
#83721=CARTESIAN_POINT('Ctrl Pts',(-0.264289733898089,0.130312652646466,
-0.550316633354963));
#83722=CARTESIAN_POINT('Ctrl Pts',(-0.271236397514644,0.115149643520624,
-0.549418281382854));
#83723=CARTESIAN_POINT('Ctrl Pts',(-0.276847274179232,0.0995450992240658,
-0.548519929410745));
#83724=CARTESIAN_POINT('Ctrl Pts',(-0.281836447440568,0.0856695892434102,
-0.547721117762148));
#83725=CARTESIAN_POINT('Ctrl Pts',(-0.285770050743515,0.0714456554660817,
-0.546922306113551));
#83726=CARTESIAN_POINT('Ctrl Pts',(-0.288615763265484,0.0570489368409436,
-0.546123494464955));
#83727=CARTESIAN_POINT('Ctrl Pts',(-0.292303929082806,0.0383901703264396,
-0.545088200212957));
#83728=CARTESIAN_POINT('Ctrl Pts',(-0.294183248271218,0.0193626650139326,
-0.544052905960959));
#83729=CARTESIAN_POINT('Ctrl Pts',(-0.294199888424845,0.000256224137824597,
-0.543017611708961));
#83730=CARTESIAN_POINT('',(-0.293720787035063,-5.32817649356945E-6,-0.443017611708961));
#83731=CARTESIAN_POINT('Ctrl Pts',(-0.294309160300636,0.000255261948186358,
-0.543017554436766));
#83732=CARTESIAN_POINT('Ctrl Pts',(-0.293592516521209,-0.0781986943848365,
-0.538768094313166));
#83733=CARTESIAN_POINT('Ctrl Pts',(-0.221008030116168,-0.25539079515841,
-0.529233860723241));
#83734=CARTESIAN_POINT('Ctrl Pts',(0.0780070236891849,-0.338696449993926,
-0.514414853666984));
#83735=CARTESIAN_POINT('Ctrl Pts',(0.326697109816754,-0.118614414899743,
-0.498560533268));
#83736=CARTESIAN_POINT('Ctrl Pts',(0.277134063845491,0.2097548369844,-0.482706212869015));
#83737=CARTESIAN_POINT('Ctrl Pts',(-0.0254342890729399,0.346631617026237,
-0.466851892470028));
#83738=CARTESIAN_POINT('Ctrl Pts',(-0.258534819861522,0.196786222189288,
-0.453622358750011));
#83739=CARTESIAN_POINT('Ctrl Pts',(-0.293712791820078,0.0493531751511997,
-0.445677598496322));
#83740=CARTESIAN_POINT('Ctrl Pts',(-0.293720787035063,-5.32817649356945E-6,
-0.443017611708961));
#83741=CARTESIAN_POINT('',(-0.294328611994138,-0.000252932005302681,-0.343017611708961));
#83742=CARTESIAN_POINT('Ctrl Pts',(-0.293720787035063,-5.32817649356945E-6,
-0.443017611708961));
#83743=CARTESIAN_POINT('Ctrl Pts',(-0.293728676447855,-0.0487106610916299,
-0.440392825029993));
#83744=CARTESIAN_POINT('Ctrl Pts',(-0.25921725196049,-0.195469311288766,
-0.432483264884698));
#83745=CARTESIAN_POINT('Ctrl Pts',(-0.0277336353910758,-0.346455230082455,
-0.419288931273073));
#83746=CARTESIAN_POINT('Ctrl Pts',(0.275736237085626,-0.211589008666704,
-0.403434610874089));
#83747=CARTESIAN_POINT('Ctrl Pts',(0.327476926891764,0.116444163611204,
-0.387580290475104));
#83748=CARTESIAN_POINT('Ctrl Pts',(0.0802525630696079,0.338171416792465,
-0.371725970076119));
#83749=CARTESIAN_POINT('Ctrl Pts',(-0.220020588114288,0.25665829857542,
-0.356871743820737));
#83750=CARTESIAN_POINT('Ctrl Pts',(-0.293610504889156,0.0788377678713336,
-0.347302291031685));
#83751=CARTESIAN_POINT('Ctrl Pts',(-0.294328611994138,-0.000252932005302681,
-0.343017611708961));
#83752=CARTESIAN_POINT('',(-0.294199939266707,0.000189038265259436,-0.24301761170896));
#83753=CARTESIAN_POINT('Ctrl Pts',(-0.294328611994138,-0.000252932005302681,
-0.343017611708961));
#83754=CARTESIAN_POINT('Ctrl Pts',(-0.294496226570651,-0.0187136241137339,
-0.342017517565357));
#83755=CARTESIAN_POINT('Ctrl Pts',(-0.28451436399033,-0.134545057927369,
-0.335732649955417));
#83756=CARTESIAN_POINT('Ctrl Pts',(-0.130893495664707,-0.321974027223704,
-0.324163008879169));
#83757=CARTESIAN_POINT('Ctrl Pts',(0.199116261936156,-0.2848738263823,-0.308308688480176));
#83758=CARTESIAN_POINT('Ctrl Pts',(0.347345858346149,0.0122975804198618,
-0.292454368081194));
#83759=CARTESIAN_POINT('Ctrl Pts',(0.178471389733922,0.298242097044996,
-0.276600047682209));
#83760=CARTESIAN_POINT('Ctrl Pts',(-0.153335856191516,0.311911054555737,
-0.260745727283223));
#83761=CARTESIAN_POINT('Ctrl Pts',(-0.288773891993813,0.12050769107895,
-0.249551581958806));
#83762=CARTESIAN_POINT('Ctrl Pts',(-0.294606220383172,0.0116992042168328,
-0.243642210100719));
#83763=CARTESIAN_POINT('Ctrl Pts',(-0.294520052322006,0.000189243954005722,
-0.24301761170896));
#83764=CARTESIAN_POINT('',(-0.294169629819823,0.000115538129147393,-0.143017616992071));
#83765=CARTESIAN_POINT('Ctrl Pts',(-0.294199939266707,0.000189038265259436,
-0.24301761170896));
#83766=CARTESIAN_POINT('Ctrl Pts',(-0.294210413722791,-0.0161123403967751,
-0.242132035518253));
#83767=CARTESIAN_POINT('Ctrl Pts',(-0.292861724548747,-0.0324669545263656,
-0.241246459327547));
#83768=CARTESIAN_POINT('Ctrl Pts',(-0.290153646990399,-0.0486261363689395,
-0.24036088313684));
#83769=CARTESIAN_POINT('Ctrl Pts',(-0.287450020653816,-0.0647587576347344,
-0.239476762552899));
#83770=CARTESIAN_POINT('Ctrl Pts',(-0.283391515145389,-0.0806957786567614,
-0.238592641968958));
#83771=CARTESIAN_POINT('Ctrl Pts',(-0.278029686489317,-0.0961932088593155,
-0.237708521385016));
#83772=CARTESIAN_POINT('Ctrl Pts',(-0.272667312880232,-0.111692214153473,
-0.236824310942892));
#83773=CARTESIAN_POINT('Ctrl Pts',(-0.266001583678496,-0.126750759356636,
-0.235940100500768));
#83774=CARTESIAN_POINT('Ctrl Pts',(-0.25813384502719,-0.141140207068994,
-0.235055890058644));
#83775=CARTESIAN_POINT('Ctrl Pts',(-0.250265301789429,-0.155531126303888,
-0.234171589193621));
#83776=CARTESIAN_POINT('Ctrl Pts',(-0.241194924416618,-0.169252114418672,
-0.233287288328597));
#83777=CARTESIAN_POINT('Ctrl Pts',(-0.231068947211838,-0.182101020410136,
-0.232402987463573));
#83778=CARTESIAN_POINT('Ctrl Pts',(-0.220921403518602,-0.194977292232783,
-0.231516803198655));
#83779=CARTESIAN_POINT('Ctrl Pts',(-0.209714330199498,-0.206977181085204,
-0.230630618933737));
#83780=CARTESIAN_POINT('Ctrl Pts',(-0.197632477220963,-0.217933576916237,
-0.229744434668819));
#83781=CARTESIAN_POINT('Ctrl Pts',(-0.194417917489317,-0.220848691750443,
-0.229508651940963));
#83782=CARTESIAN_POINT('Ctrl Pts',(-0.191141609549977,-0.223690161447638,
-0.229272869213108));
#83783=CARTESIAN_POINT('Ctrl Pts',(-0.187807393754267,-0.226455344055356,
-0.229037086485253));
#83784=CARTESIAN_POINT('Ctrl Pts',(-0.175103930922266,-0.236990773263638,
-0.228138747174525));
#83785=CARTESIAN_POINT('Ctrl Pts',(-0.161470816744965,-0.246487426797759,
-0.227240407863797));
#83786=CARTESIAN_POINT('Ctrl Pts',(-0.14710335224885,-0.254782738342202,
-0.226342068553069));
#83787=CARTESIAN_POINT('Ctrl Pts',(-0.132763705733188,-0.263061988680128,
-0.225445468587887));
#83788=CARTESIAN_POINT('Ctrl Pts',(-0.117693175521697,-0.270144066179261,
-0.224548868622706));
#83789=CARTESIAN_POINT('Ctrl Pts',(-0.10211675364506,-0.275909058613512,
-0.223652268657524));
#83790=CARTESIAN_POINT('Ctrl Pts',(-0.0865430051706365,-0.281673061594365,
-0.222755822576999));
#83791=CARTESIAN_POINT('Ctrl Pts',(-0.0704642587339777,-0.286120105226655,
-0.221859376496474));
#83792=CARTESIAN_POINT('Ctrl Pts',(-0.054126121438416,-0.289178150934738,
-0.220962930415949));
#83793=CARTESIAN_POINT('Ctrl Pts',(-0.0377922871394121,-0.292235391241328,
-0.220066720433599));
#83794=CARTESIAN_POINT('Ctrl Pts',(-0.0211999773968291,-0.293904225111132,
-0.219170510451249));
#83795=CARTESIAN_POINT('Ctrl Pts',(-0.00460404081541506,-0.294163972654997,
-0.218274300468899));
#83796=CARTESIAN_POINT('Ctrl Pts',(0.012031496910059,-0.294424340007203,
-0.217375951954599));
#83797=CARTESIAN_POINT('Ctrl Pts',(0.0286698840294532,-0.293268919895812,
-0.2164776034403));
#83798=CARTESIAN_POINT('Ctrl Pts',(0.0450568278068779,-0.290729293790601,
-0.215579254926));
#83799=CARTESIAN_POINT('Ctrl Pts',(0.0596284286406299,-0.288471007048743,
-0.214780425312756));
#83800=CARTESIAN_POINT('Ctrl Pts',(0.074000894406622,-0.285119064062116,
-0.213981595699512));
#83801=CARTESIAN_POINT('Ctrl Pts',(0.0880045204636365,-0.28072912990633,
-0.213182766086268));
#83802=CARTESIAN_POINT('Ctrl Pts',(0.103752671668509,-0.275792312357557,
-0.212284420937299));
#83803=CARTESIAN_POINT('Ctrl Pts',(0.1191341754452,-0.269510533335221,-0.211386075788329));
#83804=CARTESIAN_POINT('Ctrl Pts',(0.133906420974025,-0.261959367883508,
-0.21048773063936));
#83805=CARTESIAN_POINT('Ctrl Pts',(0.148650064165126,-0.254422823159838,
-0.209591124885481));
#83806=CARTESIAN_POINT('Ctrl Pts',(0.162786064520269,-0.245622068074354,
-0.208694519131603));
#83807=CARTESIAN_POINT('Ctrl Pts',(0.176091476700562,-0.235680783759337,
-0.207797913377724));
#83808=CARTESIAN_POINT('Ctrl Pts',(0.189394602919401,-0.225741207425437,
-0.206901461666889));
#83809=CARTESIAN_POINT('Ctrl Pts',(0.201866761036284,-0.214661920754577,
-0.206005009956054));
#83810=CARTESIAN_POINT('Ctrl Pts',(0.21331398541005,-0.202609929738108,
-0.205108558245219));
#83811=CARTESIAN_POINT('Ctrl Pts',(0.224758193948028,-0.190561113886608,
-0.20421234270964));
#83812=CARTESIAN_POINT('Ctrl Pts',(0.235177467856935,-0.177540683728999,
-0.203316127174062));
#83813=CARTESIAN_POINT('Ctrl Pts',(0.244415928217322,-0.163751317654744,
-0.202419911638483));
#83814=CARTESIAN_POINT('Ctrl Pts',(0.253676430712878,-0.149929051393764,
-0.201521557813275));
#83815=CARTESIAN_POINT('Ctrl Pts',(0.261750072845164,-0.135334859899756,
-0.200623203988068));
#83816=CARTESIAN_POINT('Ctrl Pts',(0.268525145292401,-0.120199360837298,
-0.19972485016286));
#83817=CARTESIAN_POINT('Ctrl Pts',(0.274549428627597,-0.10674112323439,
-0.198926048671001));
#83818=CARTESIAN_POINT('Ctrl Pts',(0.279547545477995,-0.0928556306069915,
-0.198127247179142));
#83819=CARTESIAN_POINT('Ctrl Pts',(0.283473983847011,-0.0787155669604466,
-0.197328445687283));
#83820=CARTESIAN_POINT('Ctrl Pts',(0.287889753237969,-0.0628133027789086,
-0.19643009383614));
#83821=CARTESIAN_POINT('Ctrl Pts',(0.290977268887811,-0.0464877677436698,
-0.195531741984997));
#83822=CARTESIAN_POINT('Ctrl Pts',(0.29266810287148,-0.0299836882589333,
-0.194633390133854));
#83823=CARTESIAN_POINT('Ctrl Pts',(0.294355663284042,-0.0135115618093629,
-0.1937367775538));
#83824=CARTESIAN_POINT('Ctrl Pts',(0.294651764465417,0.00313765176718028,
-0.192840164973746));
#83825=CARTESIAN_POINT('Ctrl Pts',(0.29353904714589,0.0197095865173061,
-0.191943552393691));
#83826=CARTESIAN_POINT('Ctrl Pts',(0.292426520889953,0.0362786757169076,
-0.191047093770096));
#83827=CARTESIAN_POINT('Ctrl Pts',(0.289905656740242,0.0527697220904914,
-0.190150635146501));
#83828=CARTESIAN_POINT('Ctrl Pts',(0.286011213202392,0.0689291369632328,
-0.189254176522906));
#83829=CARTESIAN_POINT('Ctrl Pts',(0.282117795410594,0.0850842956551185,
-0.188357954014917));
#83830=CARTESIAN_POINT('Ctrl Pts',(0.276851712539556,0.100907229606026,
-0.187461731506927));
#83831=CARTESIAN_POINT('Ctrl Pts',(0.27029836736703,0.116156930911237,-0.186565508998938));
#83832=CARTESIAN_POINT('Ctrl Pts',(0.26372938699065,0.13144301549588,-0.185667148251433));
#83833=CARTESIAN_POINT('Ctrl Pts',(0.255867348588167,0.146152416636982,
-0.184768787503927));
#83834=CARTESIAN_POINT('Ctrl Pts',(0.24684511433834,0.160066016153623,-0.183870426756422));
#83835=CARTESIAN_POINT('Ctrl Pts',(0.238823098224119,0.172437133599555,
-0.18307165960038));
#83836=CARTESIAN_POINT('Ctrl Pts',(0.229884776593514,0.184179177484849,
-0.182272892444339));
#83837=CARTESIAN_POINT('Ctrl Pts',(0.220150343724061,0.19516010391004,-0.181474125288298));
#83838=CARTESIAN_POINT('Ctrl Pts',(0.209202719326891,0.207509570966636,
-0.18057580867115));
#83839=CARTESIAN_POINT('Ctrl Pts',(0.197177922521696,0.218974268614063,
-0.179677492054003));
#83840=CARTESIAN_POINT('Ctrl Pts',(0.184244161819628,0.229363747866533,
-0.178779175436855));
#83841=CARTESIAN_POINT('Ctrl Pts',(0.171335443855333,0.239733110695752,
-0.17788259816745));
#83842=CARTESIAN_POINT('Ctrl Pts',(0.157521823952818,0.249030846584296,
-0.176986020898045));
#83843=CARTESIAN_POINT('Ctrl Pts',(0.143007361014738,0.257104132008026,
-0.176089443628641));
#83844=CARTESIAN_POINT('Ctrl Pts',(0.128495383990392,0.265176034708109,
-0.175193019917363));
#83845=CARTESIAN_POINT('Ctrl Pts',(0.113283465872141,0.272023473939963,
-0.174296596206086));
#83846=CARTESIAN_POINT('Ctrl Pts',(0.0976033421864677,0.277537794892932,
-0.173400172494808));
#83847=CARTESIAN_POINT('Ctrl Pts',(0.0819273458496677,0.283050664356944,
-0.172503984741707));
#83848=CARTESIAN_POINT('Ctrl Pts',(0.0657841387658264,0.287230860039296,
-0.171607796988606));
#83849=CARTESIAN_POINT('Ctrl Pts',(0.049422423466539,0.290019075335906,
-0.170711609235505));
#83850=CARTESIAN_POINT('Ctrl Pts',(0.0330216522433993,0.292813946189243,
-0.169813282254335));
#83851=CARTESIAN_POINT('Ctrl Pts',(0.0164021187292266,0.294210093330215,
-0.168914955273163));
#83852=CARTESIAN_POINT('Ctrl Pts',(-0.000180052817078031,0.294199944903093,
-0.168016628291992));
#83853=CARTESIAN_POINT('Ctrl Pts',(-0.0149276661258505,0.294190919240895,
-0.167217687157766));
#83854=CARTESIAN_POINT('Ctrl Pts',(-0.0296452847826954,0.293070348302885,
-0.166418746023539));
#83855=CARTESIAN_POINT('Ctrl Pts',(-0.044156621559926,0.290867380041856,
-0.165619804889313));
#83856=CARTESIAN_POINT('Ctrl Pts',(-0.0604738211404214,0.288390263471789,
-0.164721439553274));
#83857=CARTESIAN_POINT('Ctrl Pts',(-0.0766337890607189,0.284527946234074,
-0.163823074217236));
#83858=CARTESIAN_POINT('Ctrl Pts',(-0.0923852179586884,0.279318118822832,
-0.162924708881197));
#83859=CARTESIAN_POINT('Ctrl Pts',(-0.10810614497223,0.274118379991783,
-0.162028083186422));
#83860=CARTESIAN_POINT('Ctrl Pts',(-0.123419340305597,0.267576493686629,
-0.161131457491645));
#83861=CARTESIAN_POINT('Ctrl Pts',(-0.138085594998159,0.259780692997006,
-0.160234831796869));
#83862=CARTESIAN_POINT('Ctrl Pts',(-0.152749319206812,0.251986237377996,
-0.159338360803954));
#83863=CARTESIAN_POINT('Ctrl Pts',(-0.166765603379859,0.242938620565314,
-0.158441889811039));
#83864=CARTESIAN_POINT('Ctrl Pts',(-0.179917271215686,0.232773313587064,
-0.157545418818124));
#83865=CARTESIAN_POINT('Ctrl Pts',(-0.193065469434417,0.222610688376883,
-0.156649184328374));
#83866=CARTESIAN_POINT('Ctrl Pts',(-0.205348884843153,0.211331450939192,
-0.155752949838626));
#83867=CARTESIAN_POINT('Ctrl Pts',(-0.216582540762771,0.199112136839377,
-0.154856715348876));
#83868=CARTESIAN_POINT('Ctrl Pts',(-0.227842986920704,0.186863681884695,
-0.153958343501909));
#83869=CARTESIAN_POINT('Ctrl Pts',(-0.238048155564684,0.173671275485725,
-0.153059971654942));
#83870=CARTESIAN_POINT('Ctrl Pts',(-0.247052460849956,0.15974580303714,
-0.152161599807974));
#83871=CARTESIAN_POINT('Ctrl Pts',(-0.255057814791698,0.14736524371301,
-0.151362894702092));
#83872=CARTESIAN_POINT('Ctrl Pts',(-0.262114403808015,0.134406053636018,
-0.15056418959621));
#83873=CARTESIAN_POINT('Ctrl Pts',(-0.268150931039178,0.121031889115316,
-0.149765484490327));
#83874=CARTESIAN_POINT('Ctrl Pts',(-0.275566463726504,0.1046024835364,-0.148784320388287));
#83875=CARTESIAN_POINT('Ctrl Pts',(-0.281483199746428,0.087456415148466,
-0.147803156286247));
#83876=CARTESIAN_POINT('Ctrl Pts',(-0.285782874348049,0.0698697984065166,
-0.146821992184207));
#83877=CARTESIAN_POINT('Ctrl Pts',(-0.290055134026178,0.0523953147437289,
-0.145847084029717));
#83878=CARTESIAN_POINT('Ctrl Pts',(-0.292730644909085,0.0344863793794888,
-0.144872175875227));
#83879=CARTESIAN_POINT('Ctrl Pts',(-0.293740628263162,0.0164342114980555,
-0.143897267720738));
#83880=CARTESIAN_POINT('Ctrl Pts',(-0.294044394380078,0.0110047785107428,
-0.14360405094321));
#83881=CARTESIAN_POINT('Ctrl Pts',(-0.29419783782663,0.0055625008341258,
-0.143310834165682));
#83882=CARTESIAN_POINT('Ctrl Pts',(-0.294199977305384,0.0001155573961467,
-0.143017617388154));
#83883=CARTESIAN_POINT('',(-0.294174533184472,-0.000257752421235655,-0.0430176117089602));
#83884=CARTESIAN_POINT('Ctrl Pts',(-0.293764843131769,0.000115281138339288,
-0.143017611708961));
#83885=CARTESIAN_POINT('Ctrl Pts',(-0.293566552975499,-0.0561900665379691,
-0.139982129169754));
#83886=CARTESIAN_POINT('Ctrl Pts',(-0.250873929139425,-0.210802370330722,
-0.13166187316422));
#83887=CARTESIAN_POINT('Ctrl Pts',(-0.000847465076883103,-0.347563185600196,
-0.118056843692358));
#83888=CARTESIAN_POINT('Ctrl Pts',(0.29125633667054,-0.189629242622781,
-0.10220252329337));
#83889=CARTESIAN_POINT('Ctrl Pts',(0.317524590866241,0.141418773562067,
-0.0863482028943878));
#83890=CARTESIAN_POINT('Ctrl Pts',(0.0537942024322259,0.343370337337008,
-0.0704938824954019));
#83891=CARTESIAN_POINT('Ctrl Pts',(-0.231000450644502,0.241754108313963,
-0.05605035210026));
#83892=CARTESIAN_POINT('Ctrl Pts',(-0.293533922271702,0.0713929714457434,
-0.0468915951714457));
#83893=CARTESIAN_POINT('Ctrl Pts',(-0.294174533184472,-0.000257752421235655,
-0.0430176117089602));
#83894=CARTESIAN_POINT('',(-0.288931858183476,-0.0555073112399963,-0.0399923557954013));
#83895=CARTESIAN_POINT('Origin',(0.000858682044037384,0.000109768145102293,
-0.0410035060336729));
#83896=CARTESIAN_POINT('',(-0.2942,-3.60291088309151E-17,-0.04));
#83897=CARTESIAN_POINT('Origin',(0.,0.,-0.04));
#83898=CARTESIAN_POINT('',(-0.221686865784456,0.19341296114445,-0.0399999999999998));
#83899=CARTESIAN_POINT('Origin',(0.,0.,-0.04));
#83900=CARTESIAN_POINT('',(-0.294104385983628,0.00013338358664356,-0.1285823930633));
#83901=CARTESIAN_POINT('Ctrl Pts',(-0.221686865784456,0.19341296114445,
-0.0399999999999998));
#83902=CARTESIAN_POINT('Ctrl Pts',(-0.157463683943977,0.267024552677283,
-0.0452847734663282));
#83903=CARTESIAN_POINT('Ctrl Pts',(0.0489519852740736,0.343994364943719,
-0.0558543203989852));
#83904=CARTESIAN_POINT('Ctrl Pts',(0.315889904847724,0.145505811952091,
-0.0717086407979697));
#83905=CARTESIAN_POINT('Ctrl Pts',(0.293560564371313,-0.185886097454744,
-0.0875629611969554));
#83906=CARTESIAN_POINT('Ctrl Pts',(0.00367026792673841,-0.34753924213355,
-0.10341728159594));
#83907=CARTESIAN_POINT('Ctrl Pts',(-0.249424653403535,-0.213339276299583,
-0.117090423960635));
#83908=CARTESIAN_POINT('Ctrl Pts',(-0.29355313769381,-0.0574282297979894,
-0.125478792859001));
#83909=CARTESIAN_POINT('Ctrl Pts',(-0.293784724436548,0.000133150074073662,
-0.128582388291039));
#83910=CARTESIAN_POINT('',(-0.294199949415823,0.000172521672589196,-0.228582388287483));
#83911=CARTESIAN_POINT('Ctrl Pts',(-0.294199969731792,0.000133453410514708,
-0.12858239449028));
#83912=CARTESIAN_POINT('Ctrl Pts',(-0.294191701222119,0.0183615023300105,
-0.129563829546113));
#83913=CARTESIAN_POINT('Ctrl Pts',(-0.292485195566189,0.0365335283349674,
-0.130545264601945));
#83914=CARTESIAN_POINT('Ctrl Pts',(-0.289136128846234,0.0543501517552088,
-0.131526699657778));
#83915=CARTESIAN_POINT('Ctrl Pts',(-0.285763463296785,0.0722923180485561,
-0.132515050287553));
#83916=CARTESIAN_POINT('Ctrl Pts',(-0.280725230354817,0.0898735663263774,
-0.133503400917329));
#83917=CARTESIAN_POINT('Ctrl Pts',(-0.274127512705431,0.106807053970858,
-0.134491751547104));
#83918=CARTESIAN_POINT('Ctrl Pts',(-0.272716380507792,0.110428819997125,
-0.134703141829373));
#83919=CARTESIAN_POINT('Ctrl Pts',(-0.27123407947722,0.11402103739158,-0.134914532111641));
#83920=CARTESIAN_POINT('Ctrl Pts',(-0.269681920613827,0.117581043089598,
-0.13512592239391));
#83921=CARTESIAN_POINT('Ctrl Pts',(-0.263084384787075,0.132713041295475,
-0.136024448307453));
#83922=CARTESIAN_POINT('Ctrl Pts',(-0.255188419008939,0.147335891811453,
-0.136922974220996));
#83923=CARTESIAN_POINT('Ctrl Pts',(-0.246095307587498,0.161216437075798,
-0.137821500134539));
#83924=CARTESIAN_POINT('Ctrl Pts',(-0.237019737980359,0.175070204932921,
-0.138718292672784));
#83925=CARTESIAN_POINT('Ctrl Pts',(-0.2267519806427,0.188183820408594,-0.139615085211028));
#83926=CARTESIAN_POINT('Ctrl Pts',(-0.215439029375543,0.200348857300769,
-0.140511877749273));
#83927=CARTESIAN_POINT('Ctrl Pts',(-0.20412793911738,0.212511893013718,
-0.141408522762885));
#83928=CARTESIAN_POINT('Ctrl Pts',(-0.191772494739143,0.2237260470423,-0.142305167776498));
#83929=CARTESIAN_POINT('Ctrl Pts',(-0.178559646876333,0.233816364926408,
-0.14320181279011));
#83930=CARTESIAN_POINT('Ctrl Pts',(-0.165350221551189,0.243904069105025,
-0.144098225544835));
#83931=CARTESIAN_POINT('Ctrl Pts',(-0.151284469005638,0.252868043929967,
-0.144994638299561));
#83932=CARTESIAN_POINT('Ctrl Pts',(-0.136580711609862,0.260575035673304,
-0.145891051054287));
#83933=CARTESIAN_POINT('Ctrl Pts',(-0.121841840425093,0.268300432350466,
-0.146789604516824));
#83934=CARTESIAN_POINT('Ctrl Pts',(-0.106462637101275,0.274762505820998,
-0.147688157979362));
#83935=CARTESIAN_POINT('Ctrl Pts',(-0.0906844573864716,0.279874917040669,
-0.148586711441899));
#83936=CARTESIAN_POINT('Ctrl Pts',(-0.0766746926614438,0.284414330310121,
-0.149384555225565));
#83937=CARTESIAN_POINT('Ctrl Pts',(-0.0623510382474998,0.287890292128622,
-0.15018239900923));
#83938=CARTESIAN_POINT('Ctrl Pts',(-0.0478893678051186,0.290276158943903,
-0.150980242792895));
#83939=CARTESIAN_POINT('Ctrl Pts',(-0.0316092376920983,0.292962032774307,
-0.151878410169872));
#83940=CARTESIAN_POINT('Ctrl Pts',(-0.0150504980546004,0.294282606115574,
-0.152776577546849));
#83941=CARTESIAN_POINT('Ctrl Pts',(0.001536311502479,0.294195988665664,
-0.153674744923825));
#83942=CARTESIAN_POINT('Ctrl Pts',(0.0180909301430988,0.294109539318913,
-0.154571169178902));
#83943=CARTESIAN_POINT('Ctrl Pts',(0.0346727279743466,0.292621258171847,
-0.155467593433978));
#83944=CARTESIAN_POINT('Ctrl Pts',(0.0510270319741756,0.289741060272628,
-0.156364017689054));
#83945=CARTESIAN_POINT('Ctrl Pts',(0.0673784699368128,0.286861367118478,
-0.157260284848771));
#83946=CARTESIAN_POINT('Ctrl Pts',(0.0835017070694002,0.282590326317674,
-0.158156552008489));
#83947=CARTESIAN_POINT('Ctrl Pts',(0.099148411371516,0.276989589195162,
-0.159052819168206));
#83948=CARTESIAN_POINT('Ctrl Pts',(0.114790957672683,0.271390340428908,
-0.159948848151268));
#83949=CARTESIAN_POINT('Ctrl Pts',(0.129956480907957,0.264462373902354,
-0.16084487713433));
#83950=CARTESIAN_POINT('Ctrl Pts',(0.144414573058269,0.256316349631462,
-0.161740906117392));
#83951=CARTESIAN_POINT('Ctrl Pts',(0.158907177420407,0.248150880380399,
-0.162639073967861));
#83952=CARTESIAN_POINT('Ctrl Pts',(0.17268829868724,0.238761959669275,-0.163537241818329));
#83953=CARTESIAN_POINT('Ctrl Pts',(0.185554371171481,0.228305092670217,
-0.164435409668798));
#83954=CARTESIAN_POINT('Ctrl Pts',(0.197010167216985,0.218994424184329,
-0.165235127509825));
#83955=CARTESIAN_POINT('Ctrl Pts',(0.207740673292139,0.208837991528443,
-0.166034845350853));
#83956=CARTESIAN_POINT('Ctrl Pts',(0.21762704093381,0.197969975133588,-0.16683456319188));
#83957=CARTESIAN_POINT('Ctrl Pts',(0.228733260419431,0.185760983941939,
-0.167732956028454));
#83958=CARTESIAN_POINT('Ctrl Pts',(0.238844159081668,0.17257571088313,-0.168631348865028));
#83959=CARTESIAN_POINT('Ctrl Pts',(0.247788404176165,0.15860184978691,-0.169529741701603));
#83960=CARTESIAN_POINT('Ctrl Pts',(0.256715337775117,0.144655034956926,
-0.170426395707966));
#83961=CARTESIAN_POINT('Ctrl Pts',(0.264479623162017,0.129923284883128,
-0.171323049714328));
#83962=CARTESIAN_POINT('Ctrl Pts',(0.270951181620278,0.114625900993516,
-0.172219703720691));
#83963=CARTESIAN_POINT('Ctrl Pts',(0.277421629308804,0.0993311427266418,
-0.173116203826547));
#83964=CARTESIAN_POINT('Ctrl Pts',(0.282599434943443,0.0834716491056846,
-0.174012703932402));
#83965=CARTESIAN_POINT('Ctrl Pts',(0.286401401731565,0.0672895020504313,
-0.174909204038257));
#83966=CARTESIAN_POINT('Ctrl Pts',(0.290202367615189,0.0511116151017642,
-0.175805468131796));
#83967=CARTESIAN_POINT('Ctrl Pts',(0.292628043471786,0.0346120160572335,
-0.176701732225335));
#83968=CARTESIAN_POINT('Ctrl Pts',(0.293646114971536,0.0180443664927103,
-0.177597996318874));
#83969=CARTESIAN_POINT('Ctrl Pts',(0.294666614501627,0.00143720422616354,
-0.178496397940487));
#83970=CARTESIAN_POINT('Ctrl Pts',(0.294272782802821,-0.015237538264258,
-0.1793947995621));
#83971=CARTESIAN_POINT('Ctrl Pts',(0.292484537501183,-0.0317243648119074,
-0.180293201183713));
#83972=CARTESIAN_POINT('Ctrl Pts',(0.29089502278017,-0.0463789837706543,
-0.181091761986097));
#83973=CARTESIAN_POINT('Ctrl Pts',(0.288204638700452,-0.0608847794893923,
-0.181890322788482));
#83974=CARTESIAN_POINT('Ctrl Pts',(0.284461167510929,-0.0750698619841497,
-0.182688883590866));
#83975=CARTESIAN_POINT('Ctrl Pts',(0.280249847676779,-0.0910277567387323,
-0.183587246307071));
#83976=CARTESIAN_POINT('Ctrl Pts',(0.274678143546929,-0.106680871673802,
-0.184485609023275));
#83977=CARTESIAN_POINT('Ctrl Pts',(0.267810467978768,-0.121783386555775,
-0.18538397173948));
#83978=CARTESIAN_POINT('Ctrl Pts',(0.26095608348652,-0.136856673401306,
-0.186280595846029));
#83979=CARTESIAN_POINT('Ctrl Pts',(0.25281096995915,-0.151380736369602,
-0.187177219952578));
#83980=CARTESIAN_POINT('Ctrl Pts',(0.24348849462934,-0.16512720243236,-0.188073844059127));
#83981=CARTESIAN_POINT('Ctrl Pts',(0.234167611168175,-0.178871321203489,
-0.188970315061725));
#83982=CARTESIAN_POINT('Ctrl Pts',(0.223670164123284,-0.19183742451964,
-0.189866786064323));
#83983=CARTESIAN_POINT('Ctrl Pts',(0.212154124729109,-0.203824108879263,
-0.190763257066921));
#83984=CARTESIAN_POINT('Ctrl Pts',(0.200641112176925,-0.215807642693953,
-0.191659492443713));
#83985=CARTESIAN_POINT('Ctrl Pts',(0.188110594892172,-0.22681170567809,
-0.192555727820504));
#83986=CARTESIAN_POINT('Ctrl Pts',(0.17475791996057,-0.236671310916755,
-0.193451963197295));
#83987=CARTESIAN_POINT('Ctrl Pts',(0.161373379956778,-0.246554445301025,
-0.194350337366885));
#83988=CARTESIAN_POINT('Ctrl Pts',(0.147163418609258,-0.255287216820715,
-0.195248711536474));
#83989=CARTESIAN_POINT('Ctrl Pts',(0.132353312221677,-0.262747484752854,
-0.196147085706064));
#83990=CARTESIAN_POINT('Ctrl Pts',(0.119186279337399,-0.269380090260021,
-0.196945791800659));
#83991=CARTESIAN_POINT('Ctrl Pts',(0.105545630605282,-0.275007390975032,
-0.197744497895255));
#83992=CARTESIAN_POINT('Ctrl Pts',(0.0916017203586297,-0.279576044802375,
-0.198543203989851));
#83993=CARTESIAN_POINT('Ctrl Pts',(0.075918771298104,-0.284714486170827,
-0.199441522092471));
#83994=CARTESIAN_POINT('Ctrl Pts',(0.0597522313714575,-0.288545548764624,
-0.20033984019509));
#83995=CARTESIAN_POINT('Ctrl Pts',(0.0433434185875271,-0.290989670031681,
-0.20123815829771));
#83996=CARTESIAN_POINT('Ctrl Pts',(0.0269663873069511,-0.293429057388413,
-0.20213473648775));
#83997=CARTESIAN_POINT('Ctrl Pts',(0.0103487783849169,-0.294486655384115,
-0.20303131467779));
#83998=CARTESIAN_POINT('Ctrl Pts',(-0.00625612079583699,-0.294133474722936,
-0.203927892867829));
#83999=CARTESIAN_POINT('Ctrl Pts',(-0.022858159815875,-0.29378035489642,
-0.204824316624066));
#84000=CARTESIAN_POINT('Ctrl Pts',(-0.0394467038434414,-0.292016902995582,
-0.205720740380304));
#84001=CARTESIAN_POINT('Ctrl Pts',(-0.055766854845611,-0.288866228383708,
-0.206617164136541));
#84002=CARTESIAN_POINT('Ctrl Pts',(-0.072082701278467,-0.285716384787261,
-0.2075133514539));
#84003=CARTESIAN_POINT('Ctrl Pts',(-0.0881295203357389,-0.281180205650575,
-0.208409538771259));
#84004=CARTESIAN_POINT('Ctrl Pts',(-0.103662662809,-0.275331967521658,-0.209305726088618));
#84005=CARTESIAN_POINT('Ctrl Pts',(-0.119232869743055,-0.269469774599421,
-0.210204051846396));
#84006=CARTESIAN_POINT('Ctrl Pts',(-0.134286217966099,-0.262289574713627,
-0.211102377604173));
#84007=CARTESIAN_POINT('Ctrl Pts',(-0.148597752722107,-0.253914056101547,
-0.212000703361951));
#84008=CARTESIAN_POINT('Ctrl Pts',(-0.161325944447373,-0.246465155022065,
-0.212799643704246));
#84009=CARTESIAN_POINT('Ctrl Pts',(-0.173467401274235,-0.238071699307785,
-0.213598584046541));
#84010=CARTESIAN_POINT('Ctrl Pts',(-0.184884624867529,-0.228847799831227,
-0.214397524388836));
#84011=CARTESIAN_POINT('Ctrl Pts',(-0.197558202061853,-0.21860890058452,
-0.215284380288521));
#84012=CARTESIAN_POINT('Ctrl Pts',(-0.209423871849072,-0.207277209066597,
-0.216171236188206));
#84013=CARTESIAN_POINT('Ctrl Pts',(-0.220286301231099,-0.195006629348649,
-0.217058092087892));
#84014=CARTESIAN_POINT('Ctrl Pts',(-0.231127668029687,-0.182759842660794,
-0.21794322834681));
#84015=CARTESIAN_POINT('Ctrl Pts',(-0.240969068641305,-0.169578334548641,
-0.218828364605729));
#84016=CARTESIAN_POINT('Ctrl Pts',(-0.24965079348673,-0.15565385093677,
-0.219713500864648));
#84017=CARTESIAN_POINT('Ctrl Pts',(-0.25832987956455,-0.141733599603267,
-0.220598368090751));
#84018=CARTESIAN_POINT('Ctrl Pts',(-0.265849521406037,-0.1270714842788,
-0.221483235316853));
#84019=CARTESIAN_POINT('Ctrl Pts',(-0.272092843718152,-0.111888893092072,
-0.222368102542956));
#84020=CARTESIAN_POINT('Ctrl Pts',(-0.278335182273219,-0.0967086942183384,
-0.22325283034099));
#84021=CARTESIAN_POINT('Ctrl Pts',(-0.283301309523408,-0.0810089409982683,
-0.224137558139024));
#84022=CARTESIAN_POINT('Ctrl Pts',(-0.286922867717612,-0.0650300544417854,
-0.225022285937058));
#84023=CARTESIAN_POINT('Ctrl Pts',(-0.290551131806588,-0.0490215804187825,
-0.225908651950246));
#84024=CARTESIAN_POINT('Ctrl Pts',(-0.292829730847923,-0.0327337450470522,
-0.226795017963435));
#84025=CARTESIAN_POINT('Ctrl Pts',(-0.293741661854769,-0.0164157269348249,
-0.227681383976623));
#84026=CARTESIAN_POINT('Ctrl Pts',(-0.294050659024542,-0.0108865571016537,
-0.22798171874691));
#84027=CARTESIAN_POINT('Ctrl Pts',(-0.294203190180107,-0.00535393001506612,
-0.228282053517196));
#84028=CARTESIAN_POINT('Ctrl Pts',(-0.294199949415822,0.000172521672587396,
-0.228582388287483));
#84029=CARTESIAN_POINT('',(-0.294199886004729,-0.000258988038798538,-0.328582388295919));
#84030=CARTESIAN_POINT('Ctrl Pts',(-0.294199949415784,0.000172521738035792,
-0.22858238829104));
#84031=CARTESIAN_POINT('Ctrl Pts',(-0.294193944653124,0.010412395801695,
-0.229138873789967));
#84032=CARTESIAN_POINT('Ctrl Pts',(-0.293653364929884,0.0206363609331256,
-0.229695359288894));
#84033=CARTESIAN_POINT('Ctrl Pts',(-0.292582944662443,0.0308035792182318,
-0.230251844787821));
#84034=CARTESIAN_POINT('Ctrl Pts',(-0.290854945465596,0.0472167073747313,
-0.231150189601024));
#84035=CARTESIAN_POINT('Ctrl Pts',(-0.28773605490522,0.0635361486740394,
-0.232048534414226));
#84036=CARTESIAN_POINT('Ctrl Pts',(-0.283252424887927,0.0795091428397342,
-0.232946879227429));
#84037=CARTESIAN_POINT('Ctrl Pts',(-0.278777475512749,0.0954512120974134,
-0.233843484778072));
#84038=CARTESIAN_POINT('Ctrl Pts',(-0.27294317949145,0.111047395018861,
-0.234740090328715));
#84039=CARTESIAN_POINT('Ctrl Pts',(-0.265826731931281,0.126054704754464,
-0.235636695879358));
#84040=CARTESIAN_POINT('Ctrl Pts',(-0.25871150539682,0.141059439566153,
-0.23653314759223));
#84041=CARTESIAN_POINT('Ctrl Pts',(-0.250314854427535,0.155474766692411,
-0.237429599305103));
#84042=CARTESIAN_POINT('Ctrl Pts',(-0.240762170601427,0.169077547910092,
-0.238326051017975));
#84043=CARTESIAN_POINT('Ctrl Pts',(-0.231212002282678,0.182676747108638,
-0.2392222666683));
#84044=CARTESIAN_POINT('Ctrl Pts',(-0.220506869199112,0.19546318396303,
-0.240118482318625));
#84045=CARTESIAN_POINT('Ctrl Pts',(-0.208814657038346,0.207244008371672,
-0.241014697968949));
#84046=CARTESIAN_POINT('Ctrl Pts',(-0.197094545909162,0.219052943187789,
-0.24191305209331));
#84047=CARTESIAN_POINT('Ctrl Pts',(-0.184383230203443,0.229850928152899,
-0.24281140621767));
#84048=CARTESIAN_POINT('Ctrl Pts',(-0.170884710868931,0.239482892063801,
-0.243709760342031));
#84049=CARTESIAN_POINT('Ctrl Pts',(-0.158882050947728,0.24804747491403,
-0.244508561956956));
#84050=CARTESIAN_POINT('Ctrl Pts',(-0.146257812316769,0.255690536204456,
-0.245307363571881));
#84051=CARTESIAN_POINT('Ctrl Pts',(-0.133172282886074,0.262333343421898,
-0.246106165186807));
#84052=CARTESIAN_POINT('Ctrl Pts',(-0.118456177850664,0.269803904644476,
-0.247004504725146));
#84053=CARTESIAN_POINT('Ctrl Pts',(-0.103062719738412,0.276056066664602,
-0.247902844263485));
#84054=CARTESIAN_POINT('Ctrl Pts',(-0.0872182828589932,0.280974395871098,
-0.248801183801824));
#84055=CARTESIAN_POINT('Ctrl Pts',(-0.0714045251525122,0.285883201844082,
-0.249697783908572));
#84056=CARTESIAN_POINT('Ctrl Pts',(-0.0551422493111504,0.289463006917553,
-0.25059438401532));
#84057=CARTESIAN_POINT('Ctrl Pts',(-0.0386773703079941,0.291646534397476,
-0.251490984122068));
#84058=CARTESIAN_POINT('Ctrl Pts',(-0.0222153196436664,0.293829686790796,
-0.252387430210746));
#84059=CARTESIAN_POINT('Ctrl Pts',(-0.00555150976642623,0.294616881939503,
-0.253283876299423));
#84060=CARTESIAN_POINT('Ctrl Pts',(0.0110586081036425,0.293992086945908,
-0.254180322388101));
#84061=CARTESIAN_POINT('Ctrl Pts',(0.0276643499883317,0.293367456556428,
-0.255076532305367));
#84062=CARTESIAN_POINT('Ctrl Pts',(0.0442156376475864,0.291331615258301,
-0.255972742222633));
#84063=CARTESIAN_POINT('Ctrl Pts',(0.0604593459098051,0.287920661801404,
-0.256868952139899));
#84064=CARTESIAN_POINT('Ctrl Pts',(0.0767418126579441,0.284501569599992,
-0.257767300469091));
#84065=CARTESIAN_POINT('Ctrl Pts',(0.0927144622668592,0.279701001499387,
-0.258665648798282));
#84066=CARTESIAN_POINT('Ctrl Pts',(0.108136250535384,0.273605905126605,
-0.259563997127474));
#84067=CARTESIAN_POINT('Ctrl Pts',(0.121849616272327,0.268186022276024,
-0.26036282661358));
#84068=CARTESIAN_POINT('Ctrl Pts',(0.135127289411086,0.261743441032272,
-0.261161656099686));
#84069=CARTESIAN_POINT('Ctrl Pts',(0.147816043666688,0.254369922032318,
-0.261960485585791));
#84070=CARTESIAN_POINT('Ctrl Pts',(0.162085511569116,0.24607783988002,-0.262858830015976));
#84071=CARTESIAN_POINT('Ctrl Pts',(0.175700419929859,0.236554944148342,
-0.26375717444616));
#84072=CARTESIAN_POINT('Ctrl Pts',(0.18844083243448,0.225928512302897,-0.264655518876344));
#84073=CARTESIAN_POINT('Ctrl Pts',(0.201156577624219,0.215322654794453,
-0.265552123979413));
#84074=CARTESIAN_POINT('Ctrl Pts',(0.213000545222434,0.203617952657063,
-0.266448729082483));
#84075=CARTESIAN_POINT('Ctrl Pts',(0.223782600749857,0.190984260088705,
-0.267345334185551));
#84076=CARTESIAN_POINT('Ctrl Pts',(0.234562805187525,0.178352736503693,
-0.268241785357256));
#84077=CARTESIAN_POINT('Ctrl Pts',(0.244280907548326,0.164793104827646,
-0.26913823652896));
#84078=CARTESIAN_POINT('Ctrl Pts',(0.252784603828789,0.150511076227374,
-0.270034687700664));
#84079=CARTESIAN_POINT('Ctrl Pts',(0.261286060333827,0.136232809348548,
-0.27093090275748));
#84080=CARTESIAN_POINT('Ctrl Pts',(0.268573350408997,0.121233208783969,
-0.271827117814295));
#84081=CARTESIAN_POINT('Ctrl Pts',(0.27453919317641,0.10574436821905,-0.27272333287111));
#84082=CARTESIAN_POINT('Ctrl Pts',(0.280519270637902,0.0902185707788522,
-0.27362168632608));
#84083=CARTESIAN_POINT('Ctrl Pts',(0.285171342869688,0.0742019527911405,
-0.27452003978105));
#84084=CARTESIAN_POINT('Ctrl Pts',(0.288437377398787,0.057944105129944,
-0.275418393236019));
#84085=CARTESIAN_POINT('Ctrl Pts',(0.291341492974571,0.0434878376897345,
-0.276217197485605));
#84086=CARTESIAN_POINT('Ctrl Pts',(0.293150424617141,0.0288414314146981,
-0.277016001735191));
#84087=CARTESIAN_POINT('Ctrl Pts',(0.293857911790558,0.0141833591963492,
-0.277814805984776));
#84088=CARTESIAN_POINT('Ctrl Pts',(0.29465355880314,-0.00230125255203541,
-0.278713149076639));
#84089=CARTESIAN_POINT('Ctrl Pts',(0.294060305604828,-0.018905423218435,
-0.279611492168502));
#84090=CARTESIAN_POINT('Ctrl Pts',(0.292065444299675,-0.0353753621328946,
-0.280509835260364));
#84091=CARTESIAN_POINT('Ctrl Pts',(0.290074445374746,-0.0518134125315055,
-0.281406439011962));
#84092=CARTESIAN_POINT('Ctrl Pts',(0.286687253816457,-0.0681169628772702,
-0.282303042763559));
#84093=CARTESIAN_POINT('Ctrl Pts',(0.28194309840091,-0.0840340958426677,
-0.283199646515156));
#84094=CARTESIAN_POINT('Ctrl Pts',(0.277199757474612,-0.099948496112248,
-0.284096096335432));
#84095=CARTESIAN_POINT('Ctrl Pts',(0.271100090040711,-0.115475839928488,
-0.284992546155707));
#84096=CARTESIAN_POINT('Ctrl Pts',(0.263733984905181,-0.130376474894951,
-0.285888995975982));
#84097=CARTESIAN_POINT('Ctrl Pts',(0.256369819938901,-0.145273185161287,
-0.286785209679022));
#84098=CARTESIAN_POINT('Ctrl Pts',(0.247740240005153,-0.159542809832304,
-0.287681423382063));
#84099=CARTESIAN_POINT('Ctrl Pts',(0.237981750640039,-0.172969148585238,
-0.288577637085103));
#84100=CARTESIAN_POINT('Ctrl Pts',(0.228199976897607,-0.186427523437801,
-0.289475989211135));
#84101=CARTESIAN_POINT('Ctrl Pts',(0.21728440252953,-0.199037966770191,
-0.290374341337167));
#84102=CARTESIAN_POINT('Ctrl Pts',(0.205412988136211,-0.210616106470879,
-0.291272693463199));
#84103=CARTESIAN_POINT('Ctrl Pts',(0.194856975840137,-0.220911340130224,
-0.29207150443672));
#84104=CARTESIAN_POINT('Ctrl Pts',(0.183546081686859,-0.230390622836365,
-0.29287031541024));
#84105=CARTESIAN_POINT('Ctrl Pts',(0.171626714977173,-0.238951691155648,
-0.293669126383761));
#84106=CARTESIAN_POINT('Ctrl Pts',(0.158222199756597,-0.248579465297118,
-0.294567468897565));
#84107=CARTESIAN_POINT('Ctrl Pts',(0.143962416157296,-0.25710639961715,
-0.295465811411368));
#84108=CARTESIAN_POINT('Ctrl Pts',(0.129053485385659,-0.26438388360453,
-0.296364153925172));
#84109=CARTESIAN_POINT('Ctrl Pts',(0.114173421130027,-0.271647277003442,
-0.297260757077585));
#84110=CARTESIAN_POINT('Ctrl Pts',(0.0986473784290514,-0.277665619974595,
-0.298157360229998));
#84111=CARTESIAN_POINT('Ctrl Pts',(0.0827081353827211,-0.282334915200925,
-0.299053963382412));
#84112=CARTESIAN_POINT('Ctrl Pts',(0.0667716292524032,-0.287003408665915,
-0.29995041257974));
#84113=CARTESIAN_POINT('Ctrl Pts',(0.0504228056499476,-0.290323042082076,
-0.300846861777067));
#84114=CARTESIAN_POINT('Ctrl Pts',(0.0339116830863558,-0.292239007920316,
-0.301743310974395));
#84115=CARTESIAN_POINT('Ctrl Pts',(0.017404909675056,-0.294154469078927,
-0.302639524040348));
#84116=CARTESIAN_POINT('Ctrl Pts',(0.000736709434253774,-0.294666916399377,
-0.3035357371063));
#84117=CARTESIAN_POINT('Ctrl Pts',(-0.0158372467384842,-0.293773418837962,
-0.304431950172253));
#84118=CARTESIAN_POINT('Ctrl Pts',(-0.032450749263123,-0.292877789343251,
-0.30533030165084));
#84119=CARTESIAN_POINT('Ctrl Pts',(-0.0489687667855883,-0.290569584354962,
-0.306228653129427));
#84120=CARTESIAN_POINT('Ctrl Pts',(-0.0651398124002172,-0.286897969390626,
-0.307127004608014));
#84121=CARTESIAN_POINT('Ctrl Pts',(-0.0795191047834089,-0.283633169677061,
-0.307925818666258));
#84122=CARTESIAN_POINT('Ctrl Pts',(-0.0936237990135215,-0.279291226420072,
-0.308724632724502));
#84123=CARTESIAN_POINT('Ctrl Pts',(-0.107288476053316,-0.273939451167876,
-0.309523446782746));
#84124=CARTESIAN_POINT('Ctrl Pts',(-0.122655719149766,-0.267920865360209,
-0.310421789991748));
#84125=CARTESIAN_POINT('Ctrl Pts',(-0.137563795122085,-0.260586033187026,
-0.31132013320075));
#84126=CARTESIAN_POINT('Ctrl Pts',(-0.151775928281638,-0.252027196140113,
-0.312218476409752));
#84127=CARTESIAN_POINT('Ctrl Pts',(-0.165960544325783,-0.243484930462476,
-0.313115080272979));
#84128=CARTESIAN_POINT('Ctrl Pts',(-0.179451188460889,-0.233723711154993,
-0.314011684136206));
#84129=CARTESIAN_POINT('Ctrl Pts',(-0.192034043964477,-0.222882403878478,
-0.314908287999433));
#84130=CARTESIAN_POINT('Ctrl Pts',(-0.204614739066192,-0.212042957990307,
-0.315804737921079));
#84131=CARTESIAN_POINT('Ctrl Pts',(-0.216287323190704,-0.200124267192905,
-0.316701187842726));
#84132=CARTESIAN_POINT('Ctrl Pts',(-0.226869898260171,-0.187306404758139,
-0.317597637764372));
#84133=CARTESIAN_POINT('Ctrl Pts',(-0.237449685905562,-0.174491918516607,
-0.318493851563328));
#84134=CARTESIAN_POINT('Ctrl Pts',(-0.246939539186348,-0.160779348005506,
-0.319390065362285));
#84135=CARTESIAN_POINT('Ctrl Pts',(-0.255198032299019,-0.146381707568634,
-0.320286279161241));
#84136=CARTESIAN_POINT('Ctrl Pts',(-0.263476230596468,-0.131949713629094,
-0.321184631371923));
#84137=CARTESIAN_POINT('Ctrl Pts',(-0.270516828579833,-0.11683008743659,
-0.322082983582605));
#84138=CARTESIAN_POINT('Ctrl Pts',(-0.276224403826267,-0.101260647493601,
-0.322981335793287));
#84139=CARTESIAN_POINT('Ctrl Pts',(-0.281299552270207,-0.0874163764173602,
-0.323780146256102));
#84140=CARTESIAN_POINT('Ctrl Pts',(-0.285321315774006,-0.0732171408516279,
-0.324578956718916));
#84141=CARTESIAN_POINT('Ctrl Pts',(-0.288256284627069,-0.0588383750030366,
-0.325377767181731));
#84142=CARTESIAN_POINT('Ctrl Pts',(-0.292181063440704,-0.0396104109618327,
-0.326445974218167));
#84143=CARTESIAN_POINT('Ctrl Pts',(-0.294182527786001,-0.0199772121636394,
-0.327514181254603));
#84144=CARTESIAN_POINT('Ctrl Pts',(-0.29419988600465,-0.000258988128887952,
-0.328582388291039));
#84145=CARTESIAN_POINT('',(-0.29415272857916,1.53286667352925E-5,-0.428582389436499));
#84146=CARTESIAN_POINT('Ctrl Pts',(-0.294199886004729,-0.000258988038800302,
-0.328582388295919));
#84147=CARTESIAN_POINT('Ctrl Pts',(-0.294214252459464,0.016060720643228,
-0.329466485546049));
#84148=CARTESIAN_POINT('Ctrl Pts',(-0.292866399682999,0.0324238984400597,
-0.330350582796178));
#84149=CARTESIAN_POINT('Ctrl Pts',(-0.290161070293889,0.0485818205289264,
-0.331234680046308));
#84150=CARTESIAN_POINT('Ctrl Pts',(-0.28745670063117,0.064734010530484,
-0.332118463659412));
#84151=CARTESIAN_POINT('Ctrl Pts',(-0.28339588448832,0.0806802781392302,
-0.333002247272515));
#84152=CARTESIAN_POINT('Ctrl Pts',(-0.278035191199422,0.0961772969816719,
-0.333886030885619));
#84153=CARTESIAN_POINT('Ctrl Pts',(-0.2726762672925,0.111669200786873,-0.334769522791902));
#84154=CARTESIAN_POINT('Ctrl Pts',(-0.266018593680786,0.126711382273948,
-0.335653014698185));
#84155=CARTESIAN_POINT('Ctrl Pts',(-0.258167955624118,0.141077803671816,
-0.336536506604468));
#84156=CARTESIAN_POINT('Ctrl Pts',(-0.250299611096769,0.155476627355642,
-0.337421991154333));
#84157=CARTESIAN_POINT('Ctrl Pts',(-0.241233352702085,0.169195946460847,
-0.338307475704197));
#84158=CARTESIAN_POINT('Ctrl Pts',(-0.231119882409214,0.182036369869186,
-0.339192960254062));
#84159=CARTESIAN_POINT('Ctrl Pts',(-0.223356655053582,0.19189284083067,
-0.339872669362947));
#84160=CARTESIAN_POINT('Ctrl Pts',(-0.214977367630312,0.201231959199419,
-0.340552378471831));
#84161=CARTESIAN_POINT('Ctrl Pts',(-0.206064928528032,0.20997829704695,
-0.341232087580716));
#84162=CARTESIAN_POINT('Ctrl Pts',(-0.194285732941616,0.221537963597106,
-0.342130430497121));
#84163=CARTESIAN_POINT('Ctrl Pts',(-0.1814933687614,0.232140120048867,-0.343028773413525));
#84164=CARTESIAN_POINT('Ctrl Pts',(-0.167868878810078,0.241606455888594,
-0.34392711632993));
#84165=CARTESIAN_POINT('Ctrl Pts',(-0.154270768290315,0.251054463221398,
-0.344823719894948));
#84166=CARTESIAN_POINT('Ctrl Pts',(-0.139844334731844,0.259370515031801,
-0.345720323459967));
#84167=CARTESIAN_POINT('Ctrl Pts',(-0.124803770583353,0.26641632616673,
-0.346616927024986));
#84168=CARTESIAN_POINT('Ctrl Pts',(-0.10976578888216,0.273460927544117,
-0.347513376644219));
#84169=CARTESIAN_POINT('Ctrl Pts',(-0.0941145777494428,0.27923533905974,
-0.348409826263453));
#84170=CARTESIAN_POINT('Ctrl Pts',(-0.0780888710090381,0.283647260209814,
-0.349306275882687));
#84171=CARTESIAN_POINT('Ctrl Pts',(-0.062067385452284,0.288058019256417,
-0.350202489376392));
#84172=CARTESIAN_POINT('Ctrl Pts',(-0.0456723659216754,0.291106800988731,
-0.351098702870097));
#84173=CARTESIAN_POINT('Ctrl Pts',(-0.0291560449745601,0.292751712277557,
-0.351994916363802));
#84174=CARTESIAN_POINT('Ctrl Pts',(-0.0126003152006319,0.294400548412861,
-0.352893268270927));
#84175=CARTESIAN_POINT('Ctrl Pts',(0.00407650091495812,0.294638771795434,
-0.353791620178052));
#84176=CARTESIAN_POINT('Ctrl Pts',(0.0206183597940802,0.293476614467664,
-0.354689972085177));
#84177=CARTESIAN_POINT('Ctrl Pts',(0.0353273337368774,0.292443227471891,
-0.355488784050018));
#84178=CARTESIAN_POINT('Ctrl Pts',(0.0499292150980614,0.290303422713045,
-0.35628759601486));
#84179=CARTESIAN_POINT('Ctrl Pts',(0.0642502550476124,0.287098493075663,
-0.357086407979701));
#84180=CARTESIAN_POINT('Ctrl Pts',(0.0803556800310626,0.283494232907833,
-0.357984750992566));
#84181=CARTESIAN_POINT('Ctrl Pts',(0.0962080725173854,0.278519092851921,
-0.358883094005431));
#84182=CARTESIAN_POINT('Ctrl Pts',(0.111559358074178,0.272228120564495,
-0.359781437018295));
#84183=CARTESIAN_POINT('Ctrl Pts',(0.126880920858645,0.265949328699114,
-0.360678040682052));
#84184=CARTESIAN_POINT('Ctrl Pts',(0.141702554112727,0.258359997366554,
-0.361574644345809));
#84185=CARTESIAN_POINT('Ctrl Pts',(0.155791762320314,0.249564754709336,
-0.362471248009565));
#84186=CARTESIAN_POINT('Ctrl Pts',(0.169878551459699,0.240771022164788,
-0.363367697729582));
#84187=CARTESIAN_POINT('Ctrl Pts',(0.183232468392925,0.230772162330733,
-0.364264147449598));
#84188=CARTESIAN_POINT('Ctrl Pts',(0.195646277537678,0.219718397239853,
-0.365160597169614));
#84189=CARTESIAN_POINT('Ctrl Pts',(0.208056816893781,0.208667543702969,
-0.3660568107654));
#84190=CARTESIAN_POINT('Ctrl Pts',(0.21952715642872,0.196562870950218,-0.366953024361187));
#84191=CARTESIAN_POINT('Ctrl Pts',(0.229885034909869,0.183593329738551,
-0.367849237956974));
#84192=CARTESIAN_POINT('Ctrl Pts',(0.240267627841583,0.170592842509734,
-0.368747589966206));
#84193=CARTESIAN_POINT('Ctrl Pts',(0.249531983405,0.156724002687977,-0.369645941975438));
#84194=CARTESIAN_POINT('Ctrl Pts',(0.257547522201203,0.142207291683727,
-0.37054429398467));
#84195=CARTESIAN_POINT('Ctrl Pts',(0.264674911264882,0.129299083030145,
-0.371343105449342));
#84196=CARTESIAN_POINT('Ctrl Pts',(0.270815379416652,0.115879393160618,
-0.372141916914014));
#84197=CARTESIAN_POINT('Ctrl Pts',(0.275909149363032,0.102116508448771,
-0.372940728378687));
#84198=CARTESIAN_POINT('Ctrl Pts',(0.281637600494086,0.0866387751934325,
-0.373839071351861));
#84199=CARTESIAN_POINT('Ctrl Pts',(0.28607782017348,0.070628316426023,-0.374737414325036));
#84200=CARTESIAN_POINT('Ctrl Pts',(0.289141178182896,0.0543232830286123,
-0.375635757298211));
#84201=CARTESIAN_POINT('Ctrl Pts',(0.29219860499338,0.0380498190384939,
-0.37653236092167));
#84202=CARTESIAN_POINT('Ctrl Pts',(0.293884252773285,0.0214836689143827,
-0.377428964545129));
#84203=CARTESIAN_POINT('Ctrl Pts',(0.294159576219129,0.00487685539899314,
-0.378325568168588));
#84204=CARTESIAN_POINT('Ctrl Pts',(0.294434852392787,-0.0117271067777837,
-0.379222017847973));
#84205=CARTESIAN_POINT('Ctrl Pts',(0.293300219297199,-0.0283709308565512,
-0.380118467527358));
#84206=CARTESIAN_POINT('Ctrl Pts',(0.29076913219291,-0.0447990152099595,
-0.381014917206743));
#84207=CARTESIAN_POINT('Ctrl Pts',(0.288238711775943,-0.0612227724125754,
-0.381911130761644));
#84208=CARTESIAN_POINT('Ctrl Pts',(0.28431269893803,-0.0774301223399919,
-0.382807344316545));
#84209=CARTESIAN_POINT('Ctrl Pts',(0.279056067068374,-0.0931737700875695,
-0.383703557871446));
#84210=CARTESIAN_POINT('Ctrl Pts',(0.273786892591526,-0.10895498302791,
-0.384601909840232));
#84211=CARTESIAN_POINT('Ctrl Pts',(0.267181034925924,-0.124269538959438,
-0.385500261809018));
#84212=CARTESIAN_POINT('Ctrl Pts',(0.259352589351685,-0.138887992269224,
-0.386398613777804));
#84213=CARTESIAN_POINT('Ctrl Pts',(0.252391560853387,-0.151886673696521,
-0.387197425444426));
#84214=CARTESIAN_POINT('Ctrl Pts',(0.244464776903971,-0.164334952001692,
-0.387996237111049));
#84215=CARTESIAN_POINT('Ctrl Pts',(0.235681004253934,-0.176091181590269,
-0.388795048777672));
#84216=CARTESIAN_POINT('Ctrl Pts',(0.225802780469574,-0.189312228099913,
-0.389693391747013));
#84217=CARTESIAN_POINT('Ctrl Pts',(0.214777197428199,-0.201741502271168,
-0.390591734716355));
#84218=CARTESIAN_POINT('Ctrl Pts',(0.202755982708064,-0.213175166180508,
-0.391490077685696));
#84219=CARTESIAN_POINT('Ctrl Pts',(0.190758043173981,-0.224586692505507,
-0.392386681305044));
#84220=CARTESIAN_POINT('Ctrl Pts',(0.177768819723121,-0.235005848416589,
-0.393283284924392));
#84221=CARTESIAN_POINT('Ctrl Pts',(0.163978906594322,-0.244263296858391,
-0.394179888543739));
#84222=CARTESIAN_POINT('Ctrl Pts',(0.150191361156735,-0.253519155821049,
-0.395076338218643));
#84223=CARTESIAN_POINT('Ctrl Pts',(0.135604024403656,-0.261613220080211,
-0.395972787893546));
#84224=CARTESIAN_POINT('Ctrl Pts',(0.120438758651496,-0.268417855990407,
-0.39686923756845));
#84225=CARTESIAN_POINT('Ctrl Pts',(0.105277487427806,-0.275220699560639,
-0.397765451118659));
#84226=CARTESIAN_POINT('Ctrl Pts',(0.0895393158397275,-0.280734475153809,
-0.398661664668868));
#84227=CARTESIAN_POINT('Ctrl Pts',(0.073467135425447,-0.2848793077996,-0.399557878219076));
#84228=CARTESIAN_POINT('Ctrl Pts',(0.0573566059261533,-0.289034030238524,
-0.400456230182913));
#84229=CARTESIAN_POINT('Ctrl Pts',(0.0409112517815999,-0.291813113504055,
-0.401354582146749));
#84230=CARTESIAN_POINT('Ctrl Pts',(0.0243856814000187,-0.293187616625697,
-0.402252934110586));
#84231=CARTESIAN_POINT('Ctrl Pts',(0.0096911971505409,-0.294409820398726,
-0.403051745799276));
#84232=CARTESIAN_POINT('Ctrl Pts',(-0.00506620492991027,-0.294522218476699,
-0.403850557487967));
#84233=CARTESIAN_POINT('Ctrl Pts',(-0.0197085109287172,-0.293539119363966,
-0.404649369176657));
#84234=CARTESIAN_POINT('Ctrl Pts',(-0.0361752364739775,-0.292433526892775,
-0.405547712159046));
#84235=CARTESIAN_POINT('Ctrl Pts',(-0.0526009849869378,-0.289934500638107,
-0.406446055141434));
#84236=CARTESIAN_POINT('Ctrl Pts',(-0.0687321884564251,-0.286058606355394,
-0.407344398123822));
#84237=CARTESIAN_POINT('Ctrl Pts',(-0.0848321590850295,-0.282190216484218,
-0.408241001756541));
#84238=CARTESIAN_POINT('Ctrl Pts',(-0.100637941009124,-0.276950369006611,
-0.409137605389259));
#84239=CARTESIAN_POINT('Ctrl Pts',(-0.11590380053619,-0.270407006235539,
-0.410034209021978));
#84240=CARTESIAN_POINT('Ctrl Pts',(-0.131167038961171,-0.263864766940141,
-0.410930658710554));
#84241=CARTESIAN_POINT('Ctrl Pts',(-0.145889793476127,-0.256019719010459,
-0.41182710839913));
#84242=CARTESIAN_POINT('Ctrl Pts',(-0.159844340511968,-0.246988717973704,
-0.412723558087707));
#84243=CARTESIAN_POINT('Ctrl Pts',(-0.173795211925462,-0.237960095699165,
-0.413619771651778));
#84244=CARTESIAN_POINT('Ctrl Pts',(-0.18697761925489,-0.227746579614595,
-0.414515985215849));
#84245=CARTESIAN_POINT('Ctrl Pts',(-0.199192496923741,-0.216508635322671,
-0.415412198779921));
#84246=CARTESIAN_POINT('Ctrl Pts',(-0.211436519946146,-0.205243876692652,
-0.416310550757646));
#84247=CARTESIAN_POINT('Ctrl Pts',(-0.222707836000168,-0.192950365449024,
-0.417208902735371));
#84248=CARTESIAN_POINT('Ctrl Pts',(-0.232843764398215,-0.179826086485995,
-0.418107254713096));
#84249=CARTESIAN_POINT('Ctrl Pts',(-0.241856598558109,-0.168156020842599,
-0.418906066333944));
#84250=CARTESIAN_POINT('Ctrl Pts',(-0.249972073146481,-0.155829927224543,
-0.419704877954793));
#84251=CARTESIAN_POINT('Ctrl Pts',(-0.257105442200693,-0.143005005474584,
-0.420503689575642));
#84252=CARTESIAN_POINT('Ctrl Pts',(-0.265498603903353,-0.127915131215549,
-0.421443575771462));
#84253=CARTESIAN_POINT('Ctrl Pts',(-0.272580779171265,-0.112046037639118,
-0.422383461967282));
#84254=CARTESIAN_POINT('Ctrl Pts',(-0.278220391500258,-0.0956402308311883,
-0.423323348163103));
#84255=CARTESIAN_POINT('Ctrl Pts',(-0.28383932615922,-0.0792945760053446,
-0.424259788260948));
#84256=CARTESIAN_POINT('Ctrl Pts',(-0.288025935021425,-0.0624167389765852,
-0.425196228358794));
#84257=CARTESIAN_POINT('Ctrl Pts',(-0.290696210763236,-0.045269780736122,
-0.42613266845664));
#84258=CARTESIAN_POINT('Ctrl Pts',(-0.293024684117832,-0.0303176786928218,
-0.426949241734773));
#84259=CARTESIAN_POINT('Ctrl Pts',(-0.294200789390909,-0.0151615645798832,
-0.427765815012907));
#84260=CARTESIAN_POINT('Ctrl Pts',(-0.294199999601645,1.53098717317831E-5,
-0.42858238829104));
#84261=CARTESIAN_POINT('',(-0.294346683130411,0.000249348936495447,-0.52858238829104));
#84262=CARTESIAN_POINT('Ctrl Pts',(-0.293721445376834,1.55001453468206E-5,
-0.428582399887245));
#84263=CARTESIAN_POINT('Ctrl Pts',(-0.293743763360868,0.04810977684068,
-0.431174269916372));
#84264=CARTESIAN_POINT('Ctrl Pts',(-0.259849801060223,0.194237660365639,
-0.439050913411827));
#84265=CARTESIAN_POINT('Ctrl Pts',(-0.0298824682073853,0.346276530597267,
-0.452212330373611));
#84266=CARTESIAN_POINT('Ctrl Pts',(0.274418277941293,0.213295584266401,
-0.468066650772598));
#84267=CARTESIAN_POINT('Ctrl Pts',(0.328193052433044,-0.114410305001873,
-0.483920971171582));
#84268=CARTESIAN_POINT('Ctrl Pts',(0.0823489968487952,-0.337667055345944,
-0.499775291570567));
#84269=CARTESIAN_POINT('Ctrl Pts',(-0.219090521244163,-0.257841877924801,
-0.514662430610386));
#84270=CARTESIAN_POINT('Ctrl Pts',(-0.293628149939983,-0.0794362743206141,
-0.524264796183877));
#84271=CARTESIAN_POINT('Ctrl Pts',(-0.294346683130411,0.000249348936495447,
-0.52858238829104));
#84272=CARTESIAN_POINT('',(-0.294505057048355,-0.00019672582264435,-0.62858238829104));
#84273=CARTESIAN_POINT('Ctrl Pts',(-0.294346683130411,0.000249348936495447,
-0.52858238829104));
#84274=CARTESIAN_POINT('Ctrl Pts',(-0.294507641342876,0.0180996802079338,
-0.529549569650206));
#84275=CARTESIAN_POINT('Ctrl Pts',(-0.284909911715827,0.133313276848973,
-0.5358015244757));
#84276=CARTESIAN_POINT('Ctrl Pts',(-0.132888470050069,0.3211558065429,-0.547338252767522));
#84277=CARTESIAN_POINT('Ctrl Pts',(0.197345118413126,0.286103655668621,
-0.563192573166507));
#84278=CARTESIAN_POINT('Ctrl Pts',(0.347415497895151,-0.0101424538979736,
-0.579046893565493));
#84279=CARTESIAN_POINT('Ctrl Pts',(0.180318209615228,-0.29712916522912,
-0.594901213964478));
#84280=CARTESIAN_POINT('Ctrl Pts',(-0.151397831555328,-0.312856347464733,
-0.610755534363463));
#84281=CARTESIAN_POINT('Ctrl Pts',(-0.28842246464897,-0.121736620937465,
-0.621982592472317));
#84282=CARTESIAN_POINT('Ctrl Pts',(-0.294598450780843,-0.0123148159016998,
-0.627924877114843));
#84283=CARTESIAN_POINT('Ctrl Pts',(-0.294505057048355,-0.00019672582264435,
-0.62858238829104));
#84284=CARTESIAN_POINT('',(-0.294170636188799,-0.000106379757622669,-0.728582382959596));
#84285=CARTESIAN_POINT('Ctrl Pts',(-0.294505057048355,-0.00019672582264435,
-0.62858238829104));
#84286=CARTESIAN_POINT('Ctrl Pts',(-0.293847794765797,0.0850848378695851,
-0.633209650581171));
#84287=CARTESIAN_POINT('Ctrl Pts',(-0.210031811032951,0.268892279222193,
-0.64312168633763));
#84288=CARTESIAN_POINT('Ctrl Pts',(0.101907672028251,0.332287863050133,
-0.658318495560419));
#84289=CARTESIAN_POINT('Ctrl Pts',(0.334308601219868,0.0950692205661775,
-0.674172815959403));
#84290=CARTESIAN_POINT('Ctrl Pts',(0.261507603601085,-0.228941413482704,
-0.69002713635839));
#84291=CARTESIAN_POINT('Ctrl Pts',(-0.0500327629821309,-0.343943483986855,
-0.705881456757374));
#84292=CARTESIAN_POINT('Ctrl Pts',(-0.265545445146438,-0.182634770131956,
-0.71873318059113));
#84293=CARTESIAN_POINT('Ctrl Pts',(-0.293894681053642,-0.0424423890586008,
-0.72630013095856));
#84294=CARTESIAN_POINT('Ctrl Pts',(-0.293757281291689,-0.000107623531536137,
-0.72858230785966));
#84295=CARTESIAN_POINT('',(-0.294199880503211,0.000265163904499537,-0.828582388296047));
#84296=CARTESIAN_POINT('Ctrl Pts',(-0.294199980798989,-0.000106291460469518,
-0.72858238829104));
#84297=CARTESIAN_POINT('Ctrl Pts',(-0.294206132841855,0.0169217076386292,
-0.72949895127087));
#84298=CARTESIAN_POINT('Ctrl Pts',(-0.292729603762024,0.0339394245619945,
-0.7304155142507));
#84299=CARTESIAN_POINT('Ctrl Pts',(-0.289801721942549,0.0506813768472577,
-0.731332077230531));
#84300=CARTESIAN_POINT('Ctrl Pts',(-0.28687104797667,0.0674392949346736,
-0.732249514281852));
#84301=CARTESIAN_POINT('Ctrl Pts',(-0.282486448202963,0.0839202070110717,
-0.733166951333173));
#84302=CARTESIAN_POINT('Ctrl Pts',(-0.276729988221166,0.0998706844830533,
-0.734084388384494));
#84303=CARTESIAN_POINT('Ctrl Pts',(-0.270956766783648,0.115867605988818,
-0.735004496796436));
#84304=CARTESIAN_POINT('Ctrl Pts',(-0.263804024025265,0.131330338213574,
-0.735924605208378));
#84305=CARTESIAN_POINT('Ctrl Pts',(-0.255401444990078,0.146026510938871,
-0.736844713620321));
#84306=CARTESIAN_POINT('Ctrl Pts',(-0.253132456051998,0.149994989331775,
-0.737093174931995));
#84307=CARTESIAN_POINT('Ctrl Pts',(-0.250772576722466,0.153907732507795,
-0.73734163624367));
#84308=CARTESIAN_POINT('Ctrl Pts',(-0.248324887602851,0.157760547023112,
-0.737590097555344));
#84309=CARTESIAN_POINT('Ctrl Pts',(-0.239474961167038,0.171690880233385,
-0.738488440532336));
#84310=CARTESIAN_POINT('Ctrl Pts',(-0.229421074866712,0.184918492005382,
-0.739386783509328));
#84311=CARTESIAN_POINT('Ctrl Pts',(-0.218299103958587,0.197228652104297,
-0.740285126486319));
#84312=CARTESIAN_POINT('Ctrl Pts',(-0.207198667139453,0.209514977571271,
-0.741181730113535));
#84313=CARTESIAN_POINT('Ctrl Pts',(-0.195034726071907,0.220886753080267,
-0.74207833374075));
#84314=CARTESIAN_POINT('Ctrl Pts',(-0.181984520878497,0.231160710676844,
-0.742974937367966));
#84315=CARTESIAN_POINT('Ctrl Pts',(-0.168936556367226,0.241432904264893,
-0.743871387050956));
#84316=CARTESIAN_POINT('Ctrl Pts',(-0.155003216920538,0.250607125006237,
-0.744767836733946));
#84317=CARTESIAN_POINT('Ctrl Pts',(-0.140396075489323,0.258539323870076,
-0.745664286416936));
#84318=CARTESIAN_POINT('Ctrl Pts',(-0.125792781574502,0.266469433395266,
-0.746560499975365));
#84319=CARTESIAN_POINT('Ctrl Pts',(-0.110516738620478,0.273157802579337,
-0.747456713533794));
#84320=CARTESIAN_POINT('Ctrl Pts',(-0.09480410088293,0.278506413670815,
-0.748352927092224));
#84321=CARTESIAN_POINT('Ctrl Pts',(-0.0790539719479187,0.283867786835596,
-0.749251279064333));
#84322=CARTESIAN_POINT('Ctrl Pts',(-0.062865928264738,0.287882786569572,
-0.750149631036442));
#84323=CARTESIAN_POINT('Ctrl Pts',(-0.0464916598902995,0.290503296987564,
-0.751047983008552));
#84324=CARTESIAN_POINT('Ctrl Pts',(-0.0319317137658783,0.292833446318938,
-0.751846794657144));
#84325=CARTESIAN_POINT('Ctrl Pts',(-0.0172250876784197,0.294061728114009,
-0.752645606305737));
#84326=CARTESIAN_POINT('Ctrl Pts',(-0.00255036782839512,0.294188945448227,
-0.753444417954329));
#84327=CARTESIAN_POINT('Ctrl Pts',(0.0139528110371371,0.294332013966253,
-0.754342760931321));
#84328=CARTESIAN_POINT('Ctrl Pts',(0.0305205254267988,0.293082540944039,
-0.755241103908313));
#84329=CARTESIAN_POINT('Ctrl Pts',(0.0468986807142758,0.290437865553478,
-0.756139446885304));
#84330=CARTESIAN_POINT('Ctrl Pts',(0.0632451250166731,0.28779831071895,
-0.75703605051252));
#84331=CARTESIAN_POINT('Ctrl Pts',(0.0794019563069647,0.283768975391802,
-0.757932654139735));
#84332=CARTESIAN_POINT('Ctrl Pts',(0.0951190058655022,0.278399020693605,
-0.75882925776695));
#84333=CARTESIAN_POINT('Ctrl Pts',(0.110833356852515,0.273029988000954,
-0.75972570744994));
#84334=CARTESIAN_POINT('Ctrl Pts',(0.126107312753752,0.266320998101228,
-0.76062215713293));
#84335=CARTESIAN_POINT('Ctrl Pts',(0.140704963731675,0.258371347446399,
-0.76151860681592));
#84336=CARTESIAN_POINT('Ctrl Pts',(0.155298769692987,0.250423790727017,
-0.762414820374349));
#84337=CARTESIAN_POINT('Ctrl Pts',(0.169215934739101,0.24123661010645,-0.763311033932779));
#84338=CARTESIAN_POINT('Ctrl Pts',(0.182245826395781,0.230954754792619,
-0.764207247491208));
#84339=CARTESIAN_POINT('Ctrl Pts',(0.195306808073703,0.220648366419839,
-0.765105599463317));
#84340=CARTESIAN_POINT('Ctrl Pts',(0.207475680970353,0.209242599739005,
-0.766003951435427));
#84341=CARTESIAN_POINT('Ctrl Pts',(0.218575255425636,0.196922567816942,
-0.766902303407536));
#84342=CARTESIAN_POINT('Ctrl Pts',(0.228444960891387,0.185967635545503,
-0.767701115056129));
#84343=CARTESIAN_POINT('Ctrl Pts',(0.237469497284348,0.174290680893861,
-0.768499926704721));
#84344=CARTESIAN_POINT('Ctrl Pts',(0.245552471266777,0.162042043478779,
-0.769298738353313));
#84345=CARTESIAN_POINT('Ctrl Pts',(0.25464257770566,0.148267235088153,-0.770197081330305));
#84346=CARTESIAN_POINT('Ctrl Pts',(0.262598878608108,0.133681364566294,
-0.771095424307297));
#84347=CARTESIAN_POINT('Ctrl Pts',(0.269281031782881,0.118496269654141,
-0.771993767284289));
#84348=CARTESIAN_POINT('Ctrl Pts',(0.275950247135542,0.103340575752651,
-0.772890370911504));
#84349=CARTESIAN_POINT('Ctrl Pts',(0.281349836516313,0.0875886496786563,
-0.77378697453872));
#84350=CARTESIAN_POINT('Ctrl Pts',(0.285385090316645,0.07147720073534,-0.774683578165935));
#84351=CARTESIAN_POINT('Ctrl Pts',(0.289419651275681,0.0553685180807732,
-0.775580027848925));
#84352=CARTESIAN_POINT('Ctrl Pts',(0.292090099088861,0.0389011873066432,
-0.776476477531915));
#84353=CARTESIAN_POINT('Ctrl Pts',(0.293351557311752,0.0223271991698397,
-0.777372927214905));
#84354=CARTESIAN_POINT('Ctrl Pts',(0.294612683266951,0.00575757661622281,
-0.778269140773334));
#84355=CARTESIAN_POINT('Ctrl Pts',(0.294465507332073,-0.0109178577085512,
-0.779165354331764));
#84356=CARTESIAN_POINT('Ctrl Pts',(0.292917212511679,-0.0274435168006569,
-0.780061567890193));
#84357=CARTESIAN_POINT('Ctrl Pts',(0.291365223376695,-0.0440086070028396,
-0.780959919862303));
#84358=CARTESIAN_POINT('Ctrl Pts',(0.288405539004933,-0.0604224197705049,
-0.781858271834412));
#84359=CARTESIAN_POINT('Ctrl Pts',(0.284097232724547,-0.0764356092293033,
-0.782756623806522));
#84360=CARTESIAN_POINT('Ctrl Pts',(0.280266300807744,-0.0906744851575982,
-0.783555435455115));
#84361=CARTESIAN_POINT('Ctrl Pts',(0.27536993496698,-0.104596379015757,
-0.784354247103707));
#84362=CARTESIAN_POINT('Ctrl Pts',(0.269481935551342,-0.118038664900542,
-0.7851530587523));
#84363=CARTESIAN_POINT('Ctrl Pts',(0.262860295853311,-0.133155849459113,
-0.786051401729291));
#84364=CARTESIAN_POINT('Ctrl Pts',(0.254941599989955,-0.147762169966145,
-0.786949744706283));
#84365=CARTESIAN_POINT('Ctrl Pts',(0.245827381463146,-0.161624684138818,
-0.787848087683274));
#84366=CARTESIAN_POINT('Ctrl Pts',(0.2367308096641,-0.175460358049434,-0.78874469131049));
#84367=CARTESIAN_POINT('Ctrl Pts',(0.226443684555273,-0.188554394765326,
-0.789641294937705));
#84368=CARTESIAN_POINT('Ctrl Pts',(0.215113219328487,-0.200698636941396,
-0.790537898564921));
#84369=CARTESIAN_POINT('Ctrl Pts',(0.203784699509509,-0.212840793986531,
-0.791434348247911));
#84370=CARTESIAN_POINT('Ctrl Pts',(0.191413694727506,-0.224032867745722,
-0.792330797930901));
#84371=CARTESIAN_POINT('Ctrl Pts',(0.17818733119506,-0.234100224266407,
-0.793227247613891));
#84372=CARTESIAN_POINT('Ctrl Pts',(0.164964451482551,-0.244164929048594,
-0.79412346117232));
#84373=CARTESIAN_POINT('Ctrl Pts',(0.150887296586511,-0.25310503423301,
-0.795019674730749));
#84374=CARTESIAN_POINT('Ctrl Pts',(0.136174307376091,-0.260787649267832,
-0.795915888289178));
#84375=CARTESIAN_POINT('Ctrl Pts',(0.121426212183275,-0.268488595434711,
-0.796814240261288));
#84376=CARTESIAN_POINT('Ctrl Pts',(0.106039969144742,-0.274925714845722,
-0.797712592233397));
#84377=CARTESIAN_POINT('Ctrl Pts',(0.0902569844850293,-0.280013065323155,
-0.798610944205506));
#84378=CARTESIAN_POINT('Ctrl Pts',(0.0762228059145374,-0.284536720803427,
-0.799409755854099));
#84379=CARTESIAN_POINT('Ctrl Pts',(0.0618756001821937,-0.287993773698357,
-0.800208567502692));
#84380=CARTESIAN_POINT('Ctrl Pts',(0.0473919864234226,-0.290357778650482,
-0.801007379151284));
#84381=CARTESIAN_POINT('Ctrl Pts',(0.0311037253238565,-0.293016336835076,
-0.801905722128276));
#84382=CARTESIAN_POINT('Ctrl Pts',(0.0145392850277297,-0.294308490311483,
-0.802804065105268));
#84383=CARTESIAN_POINT('Ctrl Pts',(-0.00205061872833332,-0.294192853351048,
-0.803702408082259));
#84384=CARTESIAN_POINT('Ctrl Pts',(-0.0186084015171033,-0.294077440284076,
-0.804599011709475));
#84385=CARTESIAN_POINT('Ctrl Pts',(-0.0351907675097167,-0.292559586994451,
-0.805495615336691));
#84386=CARTESIAN_POINT('Ctrl Pts',(-0.0515429767469632,-0.289649722161203,
-0.806392218963906));
#84387=CARTESIAN_POINT('Ctrl Pts',(-0.0678923783576141,-0.286740356943253,
-0.807288668646896));
#84388=CARTESIAN_POINT('Ctrl Pts',(-0.0840109160382376,-0.282439541045554,
-0.808185118329886));
#84389=CARTESIAN_POINT('Ctrl Pts',(-0.0996502949343614,-0.276809426717182,
-0.809081568012876));
#84390=CARTESIAN_POINT('Ctrl Pts',(-0.115285554423077,-0.271180795359126,
-0.809977781571306));
#84391=CARTESIAN_POINT('Ctrl Pts',(-0.130441164919528,-0.264223839045072,
-0.810873995129736));
#84392=CARTESIAN_POINT('Ctrl Pts',(-0.144886849942095,-0.256049684072949,
-0.811770208688165));
#84393=CARTESIAN_POINT('Ctrl Pts',(-0.159367003144902,-0.247856025128086,
-0.812668560660275));
#84394=CARTESIAN_POINT('Ctrl Pts',(-0.17313316948217,-0.238439781422285,
-0.813566912632384));
#84395=CARTESIAN_POINT('Ctrl Pts',(-0.185981997955222,-0.227956874071794,
-0.814465264604493));
#84396=CARTESIAN_POINT('Ctrl Pts',(-0.197407134398052,-0.218635506987775,
-0.815264076253085));
#84397=CARTESIAN_POINT('Ctrl Pts',(-0.20810711787855,-0.208471655328033,
-0.816062887901677));
#84398=CARTESIAN_POINT('Ctrl Pts',(-0.217963752214611,-0.197599197165696,
-0.816861699550269));
#84399=CARTESIAN_POINT('Ctrl Pts',(-0.228933235913372,-0.185499199487901,
-0.817750699898548));
#84400=CARTESIAN_POINT('Ctrl Pts',(-0.23893064891016,-0.172440167272248,
-0.818639700246826));
#84401=CARTESIAN_POINT('Ctrl Pts',(-0.247786228830629,-0.158605248342844,
-0.819528700595104));
#84402=CARTESIAN_POINT('Ctrl Pts',(-0.256625587779185,-0.144795671156542,
-0.820416072540747));
#84403=CARTESIAN_POINT('Ctrl Pts',(-0.264326770282118,-0.130213661237864,
-0.821303444486391));
#84404=CARTESIAN_POINT('Ctrl Pts',(-0.270761035164523,-0.115074331788787,
-0.822190816432034));
#84405=CARTESIAN_POINT('Ctrl Pts',(-0.277188498774112,-0.0999510052105465,
-0.823077250390385));
#84406=CARTESIAN_POINT('Ctrl Pts',(-0.282351362761424,-0.0842722594194868,
-0.823963684348736));
#84407=CARTESIAN_POINT('Ctrl Pts',(-0.286167972763128,-0.0682754081982774,
-0.824850118307087));
#84408=CARTESIAN_POINT('Ctrl Pts',(-0.289986862924126,-0.0522689999699433,
-0.825737081848138));
#84409=CARTESIAN_POINT('Ctrl Pts',(-0.292457708475443,-0.0359448942765146,
-0.826624045389189));
#84410=CARTESIAN_POINT('Ctrl Pts',(-0.293549560455702,-0.0195523798107569,
-0.82751100893024));
#84411=CARTESIAN_POINT('Ctrl Pts',(-0.293989183064208,-0.0129521078877307,
-0.82786813538384));
#84412=CARTESIAN_POINT('Ctrl Pts',(-0.294205834500301,-0.00634081004028046,
-0.82822526183744));
#84413=CARTESIAN_POINT('Ctrl Pts',(-0.294199880503295,0.000265163811891233,
-0.82858238829104));
#84414=CARTESIAN_POINT('',(-0.294199988411901,-8.25738279543517E-5,-0.928582388295833));
#84415=CARTESIAN_POINT('Ctrl Pts',(-0.294199880503211,0.00026516390450072,
-0.828582388296047));
#84416=CARTESIAN_POINT('Ctrl Pts',(-0.294180819917147,0.0214129221291205,
-0.829725660138392));
#84417=CARTESIAN_POINT('Ctrl Pts',(-0.291877645470538,0.0424583192963313,
-0.830868931980738));
#84418=CARTESIAN_POINT('Ctrl Pts',(-0.287378498393475,0.0629860195687247,
-0.832012203823083));
#84419=CARTESIAN_POINT('Ctrl Pts',(-0.286455249827511,0.0671984112763944,
-0.832246809198474));
#84420=CARTESIAN_POINT('Ctrl Pts',(-0.285439688017423,0.0713890804885765,
-0.832481414573864));
#84421=CARTESIAN_POINT('Ctrl Pts',(-0.284332815343903,0.0755545506148362,
-0.832716019949255));
#84422=CARTESIAN_POINT('Ctrl Pts',(-0.280094415899626,0.0915048280863658,
-0.833614362926246));
#84423=CARTESIAN_POINT('Ctrl Pts',(-0.27449621650345,0.107148053663296,
-0.834512705903237));
#84424=CARTESIAN_POINT('Ctrl Pts',(-0.267603032908877,0.122238524115643,
-0.835411048880228));
#84425=CARTESIAN_POINT('Ctrl Pts',(-0.260723195728369,0.137299776766904,
-0.836307652507442));
#84426=CARTESIAN_POINT('Ctrl Pts',(-0.252553616409181,0.151809660097539,
-0.837204256134657));
#84427=CARTESIAN_POINT('Ctrl Pts',(-0.243208036264824,0.165539998478337,
-0.838100859761872));
#84428=CARTESIAN_POINT('Ctrl Pts',(-0.233864060729297,0.179267979400118,
-0.838997309444861));
#84429=CARTESIAN_POINT('Ctrl Pts',(-0.223344885476473,0.192215999571075,
-0.83989375912785));
#84430=CARTESIAN_POINT('Ctrl Pts',(-0.211808811025279,0.204182926739866,
-0.840790208810839));
#84431=CARTESIAN_POINT('Ctrl Pts',(-0.200275775172416,0.216146701823857,
-0.841686422369268));
#84432=CARTESIAN_POINT('Ctrl Pts',(-0.187726928953047,0.227129334897843,
-0.842582635927696));
#84433=CARTESIAN_POINT('Ctrl Pts',(-0.174357888097682,0.236966172392002,
-0.843478849486125));
#84434=CARTESIAN_POINT('Ctrl Pts',(-0.160956947992875,0.246826481108693,
-0.844377201458233));
#84435=CARTESIAN_POINT('Ctrl Pts',(-0.146732560293176,0.255535084654648,
-0.845275553430342));
#84436=CARTESIAN_POINT('Ctrl Pts',(-0.131910198224532,0.262970225699345,
-0.846173905402451));
#84437=CARTESIAN_POINT('Ctrl Pts',(-0.118730202134191,0.269581528907729,
-0.846972717051047));
#84438=CARTESIAN_POINT('Ctrl Pts',(-0.10507815685663,0.275186454133451,
-0.847771528699643));
#84439=CARTESIAN_POINT('Ctrl Pts',(-0.0911245813838285,0.279731926436047,
-0.848570340348239));
#84440=CARTESIAN_POINT('Ctrl Pts',(-0.0754324009406084,0.284843761156189,
-0.849468683325231));
#84441=CARTESIAN_POINT('Ctrl Pts',(-0.0592588605196882,0.28864730334519,
-0.850367026302223));
#84442=CARTESIAN_POINT('Ctrl Pts',(-0.0428454299491573,0.291063410844565,
-0.851265369279215));
#84443=CARTESIAN_POINT('Ctrl Pts',(-0.0264637786628479,0.293474840335487,
-0.85216197290643));
#84444=CARTESIAN_POINT('Ctrl Pts',(-0.00984392323024985,0.294503988488651,
-0.853058576533646));
#84445=CARTESIAN_POINT('Ctrl Pts',(0.00676078633986324,0.294122307498202,
-0.853955180160861));
#84446=CARTESIAN_POINT('Ctrl Pts',(0.0233626449298178,0.293740692041265,
-0.854851629843851));
#84447=CARTESIAN_POINT('Ctrl Pts',(0.0399485732106359,0.291948693879664,
-0.855748079526841));
#84448=CARTESIAN_POINT('Ctrl Pts',(0.0562637016785053,0.288769866629869,
-0.856644529209831));
#84449=CARTESIAN_POINT('Ctrl Pts',(0.0725745327467388,0.285591876682158,
-0.85754074276826));
#84450=CARTESIAN_POINT('Ctrl Pts',(0.0886139310497688,0.281027944961326,
-0.85843695632669));
#84451=CARTESIAN_POINT('Ctrl Pts',(0.104137364816809,0.27515277438,-0.859333169885119));
#84452=CARTESIAN_POINT('Ctrl Pts',(0.119697838330478,0.269263585326149,
-0.860231521857229));
#84453=CARTESIAN_POINT('Ctrl Pts',(0.134739154957633,0.262057214861473,
-0.861129873829338));
#84454=CARTESIAN_POINT('Ctrl Pts',(0.149036560993871,0.253656743429226,
-0.862028225801448));
#84455=CARTESIAN_POINT('Ctrl Pts',(0.161749767889358,0.246187071583362,
-0.86282703745004));
#84456=CARTESIAN_POINT('Ctrl Pts',(0.173874807294979,0.237774168014653,
-0.863625849098632));
#84457=CARTESIAN_POINT('Ctrl Pts',(0.185274446102504,0.228532316361189,
-0.864424660747224));
#84458=CARTESIAN_POINT('Ctrl Pts',(0.198094471299975,0.218138936968282,
-0.865323003724216));
#84459=CARTESIAN_POINT('Ctrl Pts',(0.210077966267995,0.206630410073749,
-0.866221346701208));
#84460=CARTESIAN_POINT('Ctrl Pts',(0.221027253292019,0.194166406214323,
-0.8671196896782));
#84461=CARTESIAN_POINT('Ctrl Pts',(0.231955340573379,0.18172653485538,-0.868016293305416));
#84462=CARTESIAN_POINT('Ctrl Pts',(0.241852629174775,0.168335402757517,
-0.868912896932632));
#84463=CARTESIAN_POINT('Ctrl Pts',(0.250557452409647,0.154190152221169,
-0.869809500559847));
#84464=CARTESIAN_POINT('Ctrl Pts',(0.259260781051781,0.140047330383046,
-0.870705950242837));
#84465=CARTESIAN_POINT('Ctrl Pts',(0.26677159269054,0.125151291215711,-0.871602399925827));
#84466=CARTESIAN_POINT('Ctrl Pts',(0.272971128054464,0.109728771289363,
-0.872498849608818));
#84467=CARTESIAN_POINT('Ctrl Pts',(0.279169030462751,0.0943103136498444,
-0.873395063167247));
#84468=CARTESIAN_POINT('Ctrl Pts',(0.284056057367643,0.0783663888285661,
-0.874291276725677));
#84469=CARTESIAN_POINT('Ctrl Pts',(0.287562002499989,0.0621428573385242,
-0.875187490284106));
#84470=CARTESIAN_POINT('Ctrl Pts',(0.291076313005703,0.0458806156310878,
-0.876085842256216));
#84471=CARTESIAN_POINT('Ctrl Pts',(0.293202818486535,0.0293382169056149,
-0.876984194228326));
#84472=CARTESIAN_POINT('Ctrl Pts',(0.293922670218187,0.0127712149700344,
-0.877882546200435));
#84473=CARTESIAN_POINT('Ctrl Pts',(0.294562760034155,-0.00196010920939629,
-0.878681357849027));
#84474=CARTESIAN_POINT('Ctrl Pts',(0.294091424201564,-0.0167104098699517,
-0.879480169497618));
#84475=CARTESIAN_POINT('Ctrl Pts',(0.292530000364165,-0.0313023782952973,
-0.880278981146209));
#84476=CARTESIAN_POINT('Ctrl Pts',(0.290774024295327,-0.0477124949711212,
-0.881177324123201));
#84477=CARTESIAN_POINT('Ctrl Pts',(0.287627325274582,-0.0640265572550334,
-0.882075667100193));
#84478=CARTESIAN_POINT('Ctrl Pts',(0.283116484548468,-0.0799918506906604,
-0.882974010077184));
#84479=CARTESIAN_POINT('Ctrl Pts',(0.278614377602224,-0.0959262325142659,
-0.883870613704399));
#84480=CARTESIAN_POINT('Ctrl Pts',(0.272753521046517,-0.111512415528557,
-0.884767217331615));
#84481=CARTESIAN_POINT('Ctrl Pts',(0.26561152264705,-0.126507545376218,
-0.88566382095883));
#84482=CARTESIAN_POINT('Ctrl Pts',(0.258470750507858,-0.141500100603859,
-0.88656027064182));
#84483=CARTESIAN_POINT('Ctrl Pts',(0.250049564838929,-0.15590106953921,
-0.88745672032481));
#84484=CARTESIAN_POINT('Ctrl Pts',(0.240473736062526,-0.169487528343918,
-0.8883531700078));
#84485=CARTESIAN_POINT('Ctrl Pts',(0.23090042955637,-0.18307040847971,-0.889249383566229));
#84486=CARTESIAN_POINT('Ctrl Pts',(0.220173548559716,-0.195838563975285,
-0.890145597124658));
#84487=CARTESIAN_POINT('Ctrl Pts',(0.208461306045207,-0.207599431314073,
-0.891041810683087));
#84488=CARTESIAN_POINT('Ctrl Pts',(0.196721117491071,-0.219388360713931,
-0.891940162655197));
#84489=CARTESIAN_POINT('Ctrl Pts',(0.183991451155372,-0.230164657672262,
-0.892838514627306));
#84490=CARTESIAN_POINT('Ctrl Pts',(0.170476570948616,-0.239773598958687,
-0.893736866599416));
#84491=CARTESIAN_POINT('Ctrl Pts',(0.158459183472808,-0.248317838264157,
-0.894535678248009));
#84492=CARTESIAN_POINT('Ctrl Pts',(0.145821771244907,-0.255939474520686,
-0.895334489896602));
#84493=CARTESIAN_POINT('Ctrl Pts',(0.132724762784979,-0.262560045215701,
-0.896133301545195));
#84494=CARTESIAN_POINT('Ctrl Pts',(0.11799587695776,-0.270005534021504,
-0.897031644522186));
#84495=CARTESIAN_POINT('Ctrl Pts',(0.102591714714734,-0.276231457930542,
-0.897929987499178));
#84496=CARTESIAN_POINT('Ctrl Pts',(0.0867388493208474,-0.281122770366428,
-0.89882833047617));
#84497=CARTESIAN_POINT('Ctrl Pts',(0.070916677858549,-0.286004612362393,
-0.899724934103385));
#84498=CARTESIAN_POINT('Ctrl Pts',(0.0546482555416442,-0.289556678780755,
-0.900621537730601));
#84499=CARTESIAN_POINT('Ctrl Pts',(0.0381796137648128,-0.291712113380246,
-0.901518141357816));
#84500=CARTESIAN_POINT('Ctrl Pts',(0.0217137996056978,-0.293867177897909,
-0.902414591040806));
#84501=CARTESIAN_POINT('Ctrl Pts',(0.00504860934839983,-0.294625932163573,
-0.903311040723796));
#84502=CARTESIAN_POINT('Ctrl Pts',(-0.0115604770754096,-0.293972779981054,
-0.904207490406786));
#84503=CARTESIAN_POINT('Ctrl Pts',(-0.0281651886711505,-0.293319799838611,
-0.905103703965216));
#84504=CARTESIAN_POINT('Ctrl Pts',(-0.0447130355484239,-0.291255693639326,
-0.905999917523645));
#84505=CARTESIAN_POINT('Ctrl Pts',(-0.0609509529546465,-0.287816992781734,
-0.906896131082075));
#84506=CARTESIAN_POINT('Ctrl Pts',(-0.0772276149038328,-0.284370086999225,
-0.907794483054184));
#84507=CARTESIAN_POINT('Ctrl Pts',(-0.0931920987770226,-0.27954222662271,
-0.908692835026294));
#84508=CARTESIAN_POINT('Ctrl Pts',(-0.108603507643358,-0.273420771207235,
-0.909591186998403));
#84509=CARTESIAN_POINT('Ctrl Pts',(-0.122307282228212,-0.267977592983072,
-0.910389998646995));
#84510=CARTESIAN_POINT('Ctrl Pts',(-0.135573638549765,-0.261512508529333,
-0.911188810295588));
#84511=CARTESIAN_POINT('Ctrl Pts',(-0.148249517976513,-0.25411753268858,
-0.91198762194418));
#84512=CARTESIAN_POINT('Ctrl Pts',(-0.162504802410936,-0.245801148440465,
-0.912885964921172));
#84513=CARTESIAN_POINT('Ctrl Pts',(-0.176103433444403,-0.236255071919387,
-0.913784307898164));
#84514=CARTESIAN_POINT('Ctrl Pts',(-0.1888256923921,-0.22560695444211,-0.914682650875156));
#84515=CARTESIAN_POINT('Ctrl Pts',(-0.201523318812107,-0.21497945359036,
-0.915579254502371));
#84516=CARTESIAN_POINT('Ctrl Pts',(-0.213347299436118,-0.203254598677624,
-0.916475858129586));
#84517=CARTESIAN_POINT('Ctrl Pts',(-0.224107789841095,-0.190602566962095,
-0.917372461756802));
#84518=CARTESIAN_POINT('Ctrl Pts',(-0.234866432701281,-0.177952707563477,
-0.918268911439792));
#84519=CARTESIAN_POINT('Ctrl Pts',(-0.244561396867179,-0.164376554051912,
-0.919165361122782));
#84520=CARTESIAN_POINT('Ctrl Pts',(-0.253040729395735,-0.150080076182265,
-0.920061810805772));
#84521=CARTESIAN_POINT('Ctrl Pts',(-0.261517828470805,-0.135787364000332,
-0.920958024364201));
#84522=CARTESIAN_POINT('Ctrl Pts',(-0.26877953739386,-0.12077539030623,
-0.92185423792263));
#84523=CARTESIAN_POINT('Ctrl Pts',(-0.274718971229571,-0.105276430631771,
-0.92275045148106));
#84524=CARTESIAN_POINT('Ctrl Pts',(-0.280672576873383,-0.0897404896071807,
-0.923648803453169));
#84525=CARTESIAN_POINT('Ctrl Pts',(-0.285297346785762,-0.0737159932216456,
-0.924547155425279));
#84526=CARTESIAN_POINT('Ctrl Pts',(-0.288535674185864,-0.0574526302453492,
-0.925445507397388));
#84527=CARTESIAN_POINT('Ctrl Pts',(-0.291415184366136,-0.0429913008398588,
-0.926244319045981));
#84528=CARTESIAN_POINT('Ctrl Pts',(-0.293199167584255,-0.0283416956942673,
-0.927043130694573));
#84529=CARTESIAN_POINT('Ctrl Pts',(-0.293881667635058,-0.0136823034624134,
-0.927841942343165));
#84530=CARTESIAN_POINT('Ctrl Pts',(-0.294092545212991,-0.00915287211042962,
-0.928088757659124));
#84531=CARTESIAN_POINT('Ctrl Pts',(-0.294198715293188,-0.00461852814225763,
-0.928335572975082));
#84532=CARTESIAN_POINT('Ctrl Pts',(-0.294199988411877,-8.25739160334692E-5,
-0.92858238829104));
#84533=CARTESIAN_POINT('',(-0.294199928089091,-0.000205699718015333,-1.0285823844888));
#84534=CARTESIAN_POINT('Ctrl Pts',(-0.294199988411901,-8.25738279557236E-5,
-0.928582388295833));
#84535=CARTESIAN_POINT('Ctrl Pts',(-0.294204588369096,0.0163064853534643,
-0.929474167757955));
#84536=CARTESIAN_POINT('Ctrl Pts',(-0.292835398088322,0.0327506834817695,
-0.930365947220078));
#84537=CARTESIAN_POINT('Ctrl Pts',(-0.290090925180525,0.0489989298649158,
-0.931257726682201));
#84538=CARTESIAN_POINT('Ctrl Pts',(-0.287351618275598,0.065216591691298,
-0.932147827521355));
#84539=CARTESIAN_POINT('Ctrl Pts',(-0.283242232594176,0.0812382391810373,
-0.933037928360509));
#84540=CARTESIAN_POINT('Ctrl Pts',(-0.277813078325176,0.0968170104449095,
-0.933928029199663));
#84541=CARTESIAN_POINT('Ctrl Pts',(-0.272384564382425,0.112393944314655,
-0.934818025058391));
#84542=CARTESIAN_POINT('Ctrl Pts',(-0.265636807836933,0.127527332514309,
-0.935708020917118));
#84543=CARTESIAN_POINT('Ctrl Pts',(-0.257670104915801,0.141985059188213,
-0.936598016775846));
#84544=CARTESIAN_POINT('Ctrl Pts',(-0.249704640544348,0.156440538180369,
-0.937487874270673));
#84545=CARTESIAN_POINT('Ctrl Pts',(-0.240521009294745,0.170219868849409,
-0.938377731765501));
#84546=CARTESIAN_POINT('Ctrl Pts',(-0.230264818119774,0.183116775682261,
-0.939267589260328));
#84547=CARTESIAN_POINT('Ctrl Pts',(-0.219985348277369,0.196042954863879,
-0.940159466481225));
#84548=CARTESIAN_POINT('Ctrl Pts',(-0.208628991984662,0.20808210742422,
-0.941051343702122));
#84549=CARTESIAN_POINT('Ctrl Pts',(-0.196380791085716,0.219062148470585,
-0.941943220923018));
#84550=CARTESIAN_POINT('Ctrl Pts',(-0.188355916554445,0.226256139855299,
-0.942527568196062));
#84551=CARTESIAN_POINT('Ctrl Pts',(-0.179948978537917,0.232996246832922,
-0.943111915469106));
#84552=CARTESIAN_POINT('Ctrl Pts',(-0.171219041481126,0.23924397554439,
-0.94369626274215));
#84553=CARTESIAN_POINT('Ctrl Pts',(-0.157798122095816,0.248848885961546,
-0.944594605719142));
#84554=CARTESIAN_POINT('Ctrl Pts',(-0.143523812053577,0.257351498251228,
-0.945492948696134));
#84555=CARTESIAN_POINT('Ctrl Pts',(-0.128602485997264,0.264603553633211,
-0.946391291673125));
#84556=CARTESIAN_POINT('Ctrl Pts',(-0.113710050248783,0.271841567762318,
-0.947287895300341));
#84557=CARTESIAN_POINT('Ctrl Pts',(-0.0981737596890333,0.277833430257783,
-0.948184498927556));
#84558=CARTESIAN_POINT('Ctrl Pts',(-0.0822265696984143,0.282475540951127,
-0.949081102554771));
#84559=CARTESIAN_POINT('Ctrl Pts',(-0.0662821177937581,0.287116854607618,
-0.949977552237761));
#84560=CARTESIAN_POINT('Ctrl Pts',(-0.0499276489994926,0.290408605631773,
-0.950874001920751));
#84561=CARTESIAN_POINT('Ctrl Pts',(-0.0334132751689965,0.292296412982577,
-0.951770451603741));
#84562=CARTESIAN_POINT('Ctrl Pts',(-0.016903251219302,0.294183723085526,
-0.952666665162171));
#84563=CARTESIAN_POINT('Ctrl Pts',(-0.000234193245550827,0.294667744720733,
-0.9535628787206));
#84564=CARTESIAN_POINT('Ctrl Pts',(0.0163382230062328,0.293745982898488,
-0.954459092279029));
#84565=CARTESIAN_POINT('Ctrl Pts',(0.0329501819331874,0.292822021703033,
-0.955357444251139));
#84566=CARTESIAN_POINT('Ctrl Pts',(0.0494642468985899,0.290485648558417,
-0.956255796223248));
#84567=CARTESIAN_POINT('Ctrl Pts',(0.0656290149933198,0.286786457823598,
-0.957154148195358));
#84568=CARTESIAN_POINT('Ctrl Pts',(0.0800026741511515,0.283497149466652,
-0.95795295984395));
#84569=CARTESIAN_POINT('Ctrl Pts',(0.0940999003317329,0.279131174082159,
-0.958751771492543));
#84570=CARTESIAN_POINT('Ctrl Pts',(0.107755391117469,0.273756124470524,
-0.959550583141136));
#84571=CARTESIAN_POINT('Ctrl Pts',(0.123112345746703,0.267711347734855,
-0.960448926118127));
#84572=CARTESIAN_POINT('Ctrl Pts',(0.138007890201815,0.26035111008134,-0.961347269095119));
#84573=CARTESIAN_POINT('Ctrl Pts',(0.152205406482096,0.251768056428174,
-0.96224561207211));
#84574=CARTESIAN_POINT('Ctrl Pts',(0.166375433877397,0.243201621074292,
-0.963142215699325));
#84575=CARTESIAN_POINT('Ctrl Pts',(0.179849412615261,0.23341741760681,-0.96403881932654));
#84576=CARTESIAN_POINT('Ctrl Pts',(0.192413763100579,0.222554675910156,
-0.964935422953755));
#84577=CARTESIAN_POINT('Ctrl Pts',(0.204975956323599,0.211693799314538,
-0.965831872636745));
#84578=CARTESIAN_POINT('Ctrl Pts',(0.216628200390941,0.199755228104271,
-0.966728322319735));
#84579=CARTESIAN_POINT('Ctrl Pts',(0.227188904550832,0.186919345304313,
-0.967624772002725));
#84580=CARTESIAN_POINT('Ctrl Pts',(0.237746827024616,0.17408684347179,-0.968520985561154));
#84581=CARTESIAN_POINT('Ctrl Pts',(0.247213286139144,0.160358117292406,
-0.969417199119583));
#84582=CARTESIAN_POINT('Ctrl Pts',(0.255447219515767,0.145946421818638,
-0.970313412678013));
#84583=CARTESIAN_POINT('Ctrl Pts',(0.263700799499615,0.131500339265514,
-0.971211764650122));
#84584=CARTESIAN_POINT('Ctrl Pts',(0.270715609235867,0.116368735731305,
-0.972110116622231));
#84585=CARTESIAN_POINT('Ctrl Pts',(0.276396631947984,0.100789591961723,
-0.97300846859434));
#84586=CARTESIAN_POINT('Ctrl Pts',(0.281448178846364,0.0869366680470235,
-0.973807280242934));
#84587=CARTESIAN_POINT('Ctrl Pts',(0.285445733982361,0.072730574988778,
-0.974606091891527));
#84588=CARTESIAN_POINT('Ctrl Pts',(0.288356186683529,0.0583468045511799,
-0.97540490354012));
#84589=CARTESIAN_POINT('Ctrl Pts',(0.291629279594187,0.0421708271752409,
-0.976303246517112));
#84590=CARTESIAN_POINT('Ctrl Pts',(0.293547398864424,0.0256671560261943,
-0.977201589494104));
#84591=CARTESIAN_POINT('Ctrl Pts',(0.294059699922176,0.00908476095888113,
-0.978099932471096));
#84592=CARTESIAN_POINT('Ctrl Pts',(0.294571009075106,-0.00746552767927422,
-0.978996536098311));
#84593=CARTESIAN_POINT('Ctrl Pts',(0.293681813083,-0.0240934581280533,-0.979893139725527));
#84594=CARTESIAN_POINT('Ctrl Pts',(0.291392892362341,-0.0405440782446629,
-0.980789743352743));
#84595=CARTESIAN_POINT('Ctrl Pts',(0.289104364642687,-0.056991873837822,
-0.981686193035733));
#84596=CARTESIAN_POINT('Ctrl Pts',(0.285416645893085,-0.0732616312045314,
-0.982582642718723));
#84597=CARTESIAN_POINT('Ctrl Pts',(0.280382446964167,-0.0891028811789288,
-0.983479092401713));
#84598=CARTESIAN_POINT('Ctrl Pts',(0.275349574041641,-0.104939958573134,
-0.984375305960143));
#84599=CARTESIAN_POINT('Ctrl Pts',(0.268971175164861,-0.120348001876696,
-0.985271519518573));
#84600=CARTESIAN_POINT('Ctrl Pts',(0.261349582064675,-0.135092693935016,
-0.986167733077002));
#84601=CARTESIAN_POINT('Ctrl Pts',(0.253709803434047,-0.149872567620426,
-0.987066085049112));
#84602=CARTESIAN_POINT('Ctrl Pts',(0.244821294629877,-0.163985235418924,
-0.987964437021221));
#84603=CARTESIAN_POINT('Ctrl Pts',(0.234832169121801,-0.177221591081758,
-0.988862788993331));
#84604=CARTESIAN_POINT('Ctrl Pts',(0.225949871244333,-0.188991315439945,
-0.989661600641922));
#84605=CARTESIAN_POINT('Ctrl Pts',(0.216198248486144,-0.20006829068708,
-0.990460412290513));
#84606=CARTESIAN_POINT('Ctrl Pts',(0.20570660980217,-0.210329338618506,
-0.991259223939104));
#84607=CARTESIAN_POINT('Ctrl Pts',(0.19390772085819,-0.22186890537624,-0.992157566916095));
#84608=CARTESIAN_POINT('Ctrl Pts',(0.181097297278634,-0.232449235741734,
-0.993055909893087));
#84609=CARTESIAN_POINT('Ctrl Pts',(0.167456685694875,-0.241892328146404,
-0.993954252870079));
#84610=CARTESIAN_POINT('Ctrl Pts',(0.153842484730798,-0.251317137065721,
-0.994850856497294));
#84611=CARTESIAN_POINT('Ctrl Pts',(0.139401891896317,-0.259608579588606,
-0.995747460124509));
#84612=CARTESIAN_POINT('Ctrl Pts',(0.124349335150208,-0.266628735975141,
-0.996644063751725));
#84613=CARTESIAN_POINT('Ctrl Pts',(0.109299362884145,-0.273647687021319,
-0.997540513434715));
#84614=CARTESIAN_POINT('Ctrl Pts',(0.0936383277748143,-0.279395404277063,
-0.998436963117705));
#84615=CARTESIAN_POINT('Ctrl Pts',(0.077605120709974,-0.283779994431585,
-0.999333412800695));
#84616=CARTESIAN_POINT('Ctrl Pts',(0.0615761367867639,-0.288163429686457,
-1.00022962635912));
#84617=CARTESIAN_POINT('Ctrl Pts',(0.0451759416647873,-0.291184252527466,
-1.00112583991755));
#84618=CARTESIAN_POINT('Ctrl Pts',(0.0286568389950925,-0.292800999962106,
-1.00202205347598));
#84619=CARTESIAN_POINT('Ctrl Pts',(0.0120983208592947,-0.294421605042951,
-1.00292040544809));
#84620=CARTESIAN_POINT('Ctrl Pts',(-0.0045788782537557,-0.29463139278357,
-1.0038187574202));
#84621=CARTESIAN_POINT('Ctrl Pts',(-0.0211187325561017,-0.293441031785304,
-1.00471710939231));
#84622=CARTESIAN_POINT('Ctrl Pts',(-0.0358259171484693,-0.292382566661426,
-1.0055159210409));
#84623=CARTESIAN_POINT('Ctrl Pts',(-0.0504241228796736,-0.290217868882573,
-1.0063147326895));
#84624=CARTESIAN_POINT('Ctrl Pts',(-0.0647396718010162,-0.286988527462505,
-1.00711354433809));
#84625=CARTESIAN_POINT('Ctrl Pts',(-0.0808389273112742,-0.283356812539297,
-1.00801188731508));
#84626=CARTESIAN_POINT('Ctrl Pts',(-0.0966828133703411,-0.278354651258673,
-1.00891023029207));
#84627=CARTESIAN_POINT('Ctrl Pts',(-0.112023349778221,-0.272037514149182,
-1.00980857326906));
#84628=CARTESIAN_POINT('Ctrl Pts',(-0.127334184213414,-0.26573260812659,
-1.01070517689628));
#84629=CARTESIAN_POINT('Ctrl Pts',(-0.142142855419589,-0.258118017026034,
-1.01160178052349));
#84630=CARTESIAN_POINT('Ctrl Pts',(-0.15621704662262,-0.249298765228603,
-1.01249838415071));
#84631=CARTESIAN_POINT('Ctrl Pts',(-0.170288821328098,-0.240481027670966,
-1.0133948338337));
#84632=CARTESIAN_POINT('Ctrl Pts',(-0.183625670208904,-0.230459414214168,
-1.01429128351669));
#84633=CARTESIAN_POINT('Ctrl Pts',(-0.196020614124134,-0.219384499995778,
-1.01518773319967));
#84634=CARTESIAN_POINT('Ctrl Pts',(-0.208412293215094,-0.208312502906257,
-1.0160839467581));
#84635=CARTESIAN_POINT('Ctrl Pts',(-0.219861977160234,-0.196188291252235,
-1.01698016031653));
#84636=CARTESIAN_POINT('Ctrl Pts',(-0.230197727149494,-0.183201109208452,
-1.01787637387496));
#84637=CARTESIAN_POINT('Ctrl Pts',(-0.24055813879329,-0.170182939050861,
-1.01877472584707));
#84638=CARTESIAN_POINT('Ctrl Pts',(-0.249798834234182,-0.156298324222916,
-1.01967307781918));
#84639=CARTESIAN_POINT('Ctrl Pts',(-0.257789610195065,-0.141767968439547,
-1.02057142979129));
#84640=CARTESIAN_POINT('Ctrl Pts',(-0.264894982161803,-0.128847623387292,
-1.02137024143988));
#84641=CARTESIAN_POINT('Ctrl Pts',(-0.271012562110784,-0.115417480327191,
-1.02216905308848));
#84642=CARTESIAN_POINT('Ctrl Pts',(-0.27608285972775,-0.101645927437097,
-1.02296786473708));
#84643=CARTESIAN_POINT('Ctrl Pts',(-0.282617632419822,-0.083896679848063,
-1.0239974004649));
#84644=CARTESIAN_POINT('Ctrl Pts',(-0.287447179404754,-0.0654875880066178,
-1.02502693619272));
#84645=CARTESIAN_POINT('Ctrl Pts',(-0.290464678823977,-0.0467323266667069,
-1.02605647192054));
#84646=CARTESIAN_POINT('Ctrl Pts',(-0.2929324383204,-0.031393972669156,
-1.02689844277663));
#84647=CARTESIAN_POINT('Ctrl Pts',(-0.294189007618607,-0.0158245914797193,
-1.02774041363272));
#84648=CARTESIAN_POINT('Ctrl Pts',(-0.294199928089091,-0.000205699718015333,
-1.0285823844888));
#84649=CARTESIAN_POINT('',(-0.293916367631718,0.000220716887012043,-1.12858238829104));
#84650=CARTESIAN_POINT('Ctrl Pts',(-0.293881989377092,-0.000205406963665611,
-1.02858238829104));
#84651=CARTESIAN_POINT('Ctrl Pts',(-0.293473254748503,0.0630439083385033,
-1.03199565390605));
#84652=CARTESIAN_POINT('Ctrl Pts',(-0.242431600377607,0.22482394576972,
-1.04069369298737));
#84653=CARTESIAN_POINT('Ctrl Pts',(0.0238745824446583,0.346742558480913,
-1.05467650553506));
#84654=CARTESIAN_POINT('Ctrl Pts',(0.304028168071522,0.16842586074448,-1.07053082593402));
#84655=CARTESIAN_POINT('Ctrl Pts',(0.30662388542524,-0.163652651781727,
-1.08638514633302));
#84656=CARTESIAN_POINT('Ctrl Pts',(0.0292920140283848,-0.346326977672701,
-1.10223946673199));
#84657=CARTESIAN_POINT('Ctrl Pts',(-0.240478109422872,-0.227887870294271,
-1.11630521405135));
#84658=CARTESIAN_POINT('Ctrl Pts',(-0.29346304387379,-0.0645463479691509,
-1.12508618790436));
#84659=CARTESIAN_POINT('Ctrl Pts',(-0.293916367631718,0.000220716887012043,
-1.12858238829104));
#84660=CARTESIAN_POINT('',(-0.294666739399022,5.55183184013965E-5,-1.22858238829104));
#84661=CARTESIAN_POINT('Ctrl Pts',(-0.293916367631718,0.000220716887012043,
-1.12858238829104));
#84662=CARTESIAN_POINT('Ctrl Pts',(-0.294148277299391,0.0333540089861818,
-1.13037096137068));
#84663=CARTESIAN_POINT('Ctrl Pts',(-0.273700019748768,0.164109867608507,
-1.13744430791668));
#84664=CARTESIAN_POINT('Ctrl Pts',(-0.0817731457554239,0.337806971788931,
-1.14980242792894));
#84665=CARTESIAN_POINT('Ctrl Pts',(0.239104754541022,0.252248516133763,
-1.16565674832794));
#84666=CARTESIAN_POINT('Ctrl Pts',(0.341695624457678,-0.063596366052773,
-1.18151106872693));
#84667=CARTESIAN_POINT('Ctrl Pts',(0.132340697599494,-0.321381918213206,
-1.19736538912591));
#84668=CARTESIAN_POINT('Ctrl Pts',(-0.194419760005066,-0.286134902300222,
-1.21305582898062));
#84669=CARTESIAN_POINT('Ctrl Pts',(-0.294421732944348,-0.0941869120255346,
-1.22346149536899));
#84670=CARTESIAN_POINT('Ctrl Pts',(-0.294666739399022,5.55183184013965E-5,
-1.22858238829104));
#84671=CARTESIAN_POINT('',(-0.294199884378713,-0.000260828587339853,-1.32858238829104));
#84672=CARTESIAN_POINT('Ctrl Pts',(-0.294666739399022,5.55183184013965E-5,
-1.22858238829104));
#84673=CARTESIAN_POINT('Ctrl Pts',(-0.294674580178307,0.00307149639374388,
-1.22874626883532));
#84674=CARTESIAN_POINT('Ctrl Pts',(-0.293267859366203,0.103338389888432,
-1.23419492284593));
#84675=CARTESIAN_POINT('Ctrl Pts',(-0.179811334202771,0.297436181275677,
-1.24492835032287));
#84676=CARTESIAN_POINT('Ctrl Pts',(0.151931039768365,0.312597754286858,
-1.26078267072184));
#84677=CARTESIAN_POINT('Ctrl Pts',(0.344970294287786,0.0423779900056762,
-1.27663699112084));
#84678=CARTESIAN_POINT('Ctrl Pts',(0.223074190979041,-0.266530119498471,
-1.29249131151981));
#84679=CARTESIAN_POINT('Ctrl Pts',(-0.102474082261184,-0.332113617376057,
-1.30834563191881));
#84680=CARTESIAN_POINT('Ctrl Pts',(-0.278513916599102,-0.151810516675863,
-1.3203759701921));
#84681=CARTESIAN_POINT('Ctrl Pts',(-0.294307334922772,-0.0272861447661987,
-1.32712153499908));
#84682=CARTESIAN_POINT('Ctrl Pts',(-0.294074822703788,-0.000261863787000156,
-1.32858232633972));
#84683=CARTESIAN_POINT('',(-0.294199971607144,0.000129253068963336,-1.42858238829403));
#84684=CARTESIAN_POINT('Ctrl Pts',(-0.294199884378713,-0.000260828587339853,
-1.32858238829104));
#84685=CARTESIAN_POINT('Ctrl Pts',(-0.294214457430896,0.0161767494828003,
-1.32947054750874));
#84686=CARTESIAN_POINT('Ctrl Pts',(-0.292847107883467,0.0326438671053959,
-1.33035870672644));
#84687=CARTESIAN_POINT('Ctrl Pts',(-0.290109413072103,0.0488893490134608,
-1.33124686594414));
#84688=CARTESIAN_POINT('Ctrl Pts',(-0.287371187498568,0.065137980464425,
-1.33213519735098));
#84689=CARTESIAN_POINT('Ctrl Pts',(-0.283262188325697,0.081164091081889,
-1.33302352875782));
#84690=CARTESIAN_POINT('Ctrl Pts',(-0.277845619751207,0.0967235833965424,
-1.33391186016466));
#84691=CARTESIAN_POINT('Ctrl Pts',(-0.272428273701776,0.112285309065243,
-1.33480031907942));
#84692=CARTESIAN_POINT('Ctrl Pts',(-0.265703282052838,0.127379533890134,
-1.33568877799418));
#84693=CARTESIAN_POINT('Ctrl Pts',(-0.257782474987569,0.141780942264056,
-1.33657723690894));
#84694=CARTESIAN_POINT('Ctrl Pts',(-0.249844243100468,0.156214032002386,
-1.33746765032634));
#84695=CARTESIAN_POINT('Ctrl Pts',(-0.240705391305208,0.169950591334069,
-1.33835806374374));
#84696=CARTESIAN_POINT('Ctrl Pts',(-0.230521576920559,0.182793442371598,
-1.33924847716113));
#84697=CARTESIAN_POINT('Ctrl Pts',(-0.22744956856644,0.18666756499283,-1.33951707567968));
#84698=CARTESIAN_POINT('Ctrl Pts',(-0.224282741142796,0.190460603695425,
-1.33978567419823));
#84699=CARTESIAN_POINT('Ctrl Pts',(-0.221026025179474,0.194167804214197,
-1.34005427271677));
#84700=CARTESIAN_POINT('Ctrl Pts',(-0.210133752067151,0.206566748729891,
-1.34095261584971));
#84701=CARTESIAN_POINT('Ctrl Pts',(-0.198160287921806,0.218085713957663,
-1.34185095898264));
#84702=CARTESIAN_POINT('Ctrl Pts',(-0.18527299639449,0.228533491652771,
-1.34274930211558));
#84703=CARTESIAN_POINT('Ctrl Pts',(-0.172410657020504,0.238961040539487,
-1.34364590589191));
#84704=CARTESIAN_POINT('Ctrl Pts',(-0.158638568371357,0.248320975255663,
-1.34454250966825));
#84705=CARTESIAN_POINT('Ctrl Pts',(-0.144160112338002,0.256459552387301,
-1.34543911344458));
#84706=CARTESIAN_POINT('Ctrl Pts',(-0.129684142413037,0.264596732036718,
-1.3463355632643));
#84707=CARTESIAN_POINT('Ctrl Pts',(-0.114502707569499,0.271512538177124,
-1.34723201308401));
#84708=CARTESIAN_POINT('Ctrl Pts',(-0.0988470638600188,0.277097271668729,
-1.34812846290372));
#84709=CARTESIAN_POINT('Ctrl Pts',(-0.0831955439561307,0.282680534102635,
-1.34902467659231));
#84710=CARTESIAN_POINT('Ctrl Pts',(-0.0670708121268936,0.286933164451199,
-1.3499208902809));
#84711=CARTESIAN_POINT('Ctrl Pts',(-0.0507213131812425,0.289794734923135,
-1.35081710396949));
#84712=CARTESIAN_POINT('Ctrl Pts',(-0.0343328037034058,0.292663133212082,
-1.35171545605834));
#84713=CARTESIAN_POINT('Ctrl Pts',(-0.0177192430968529,0.294133731906785,
-1.3526138081472));
#84714=CARTESIAN_POINT('Ctrl Pts',(-0.00113673073858106,0.294197803940186,
-1.35351216023605));
#84715=CARTESIAN_POINT('Ctrl Pts',(0.0136083706295909,0.294254776527147,
-1.35431097119596));
#84716=CARTESIAN_POINT('Ctrl Pts',(0.0283284775460612,0.293200444401833,
-1.35510978215586));
#84717=CARTESIAN_POINT('Ctrl Pts',(0.0428472643703829,0.291063140806208,
-1.35590859311576));
#84718=CARTESIAN_POINT('Ctrl Pts',(0.0591751221422548,0.288659524750202,
-1.35680693757785));
#84719=CARTESIAN_POINT('Ctrl Pts',(0.0753519966548785,0.284870068190489,
-1.35770528203994));
#84720=CARTESIAN_POINT('Ctrl Pts',(0.0911264218009641,0.279731326900926,
-1.35860362650203));
#84721=CARTESIAN_POINT('Ctrl Pts',(0.106870305115145,0.274602535043512,
-1.35950023162431));
#84722=CARTESIAN_POINT('Ctrl Pts',(0.122212521910924,0.268129823766632,
-1.3603968367466));
#84723=CARTESIAN_POINT('Ctrl Pts',(0.136913476641977,0.260400345456389,
-1.36129344186888));
#84724=CARTESIAN_POINT('Ctrl Pts',(0.151611907154874,0.252672194331343,
-1.36218989304015));
#84725=CARTESIAN_POINT('Ctrl Pts',(0.165668571712451,0.243688025021323,
-1.36308634421142));
#84726=CARTESIAN_POINT('Ctrl Pts',(0.178865694570038,0.233582326613076,
-1.36398279538269));
#84727=CARTESIAN_POINT('Ctrl Pts',(0.192059341298967,0.223479290050765,
-1.36487901042828));
#84728=CARTESIAN_POINT('Ctrl Pts',(0.204393274255127,0.212255800656612,
-1.36577522547386));
#84729=CARTESIAN_POINT('Ctrl Pts',(0.215681732862412,0.200087556108488,
-1.36667144051945));
#84730=CARTESIAN_POINT('Ctrl Pts',(0.226997125875596,0.187890277974012,
-1.36756979394555));
#84731=CARTESIAN_POINT('Ctrl Pts',(0.237261541710229,0.17474434307023,-1.36846814737164));
#84732=CARTESIAN_POINT('Ctrl Pts',(0.246328456267685,0.160859975235542,
-1.36936650079773));
#84733=CARTESIAN_POINT('Ctrl Pts',(0.25439063933822,0.148514175063657,-1.37016530503674));
#84734=CARTESIAN_POINT('Ctrl Pts',(0.261506436947392,0.135585335079062,
-1.37096410927574));
#84735=CARTESIAN_POINT('Ctrl Pts',(0.267603794682592,0.122236856436498,
-1.37176291351475));
#84736=CARTESIAN_POINT('Ctrl Pts',(0.274460914295383,0.107225089261934,
-1.37266125283679));
#84737=CARTESIAN_POINT('Ctrl Pts',(0.280072727254961,0.0915868095519443,
-1.37355959215882));
#84738=CARTESIAN_POINT('Ctrl Pts',(0.284333237639734,0.075552961380124,
-1.37445793148086));
#84739=CARTESIAN_POINT('Ctrl Pts',(0.288585498914575,0.0595501576053983,
-1.37535453145734));
#84740=CARTESIAN_POINT('Ctrl Pts',(0.291491386675606,0.0431540444954077,
-1.37625113143382));
#84741=CARTESIAN_POINT('Ctrl Pts',(0.292993827122456,0.0266131033165356,
-1.3771477314103));
#84742=CARTESIAN_POINT('Ctrl Pts',(0.294496009703126,0.0100750010849986,
-1.37804417750193));
#84743=CARTESIAN_POINT('Ctrl Pts',(0.294595099449247,-0.00660709924303613,
-1.37894062359357));
#84744=CARTESIAN_POINT('Ctrl Pts',(0.293285616170215,-0.0231773024240751,
-1.37983706968521));
#84745=CARTESIAN_POINT('Ctrl Pts',(0.291976477771621,-0.039743141487598,
-1.38073327967858));
#84746=CARTESIAN_POINT('Ctrl Pts',(0.289259576137544,-0.0561963539634961,
-1.38162948967196));
#84747=CARTESIAN_POINT('Ctrl Pts',(0.285181422377442,-0.0722855195096436,
-1.38252569966534));
#84748=CARTESIAN_POINT('Ctrl Pts',(0.281093537348228,-0.0884130769382262,
-1.38342404819031));
#84749=CARTESIAN_POINT('Ctrl Pts',(0.275638133828674,-0.10417408897145,
-1.38432239671527));
#84750=CARTESIAN_POINT('Ctrl Pts',(0.268912030090887,-0.11933130382426,
-1.38522074524024));
#84751=CARTESIAN_POINT('Ctrl Pts',(0.262931043507767,-0.132809403806991,
-1.38601957479807));
#84752=CARTESIAN_POINT('Ctrl Pts',(0.255946204099478,-0.145809991572696,
-1.3868184043559));
#84753=CARTESIAN_POINT('Ctrl Pts',(0.248055515898018,-0.158183757170477,
-1.38761723391373));
#84754=CARTESIAN_POINT('Ctrl Pts',(0.239181831423695,-0.172099006242618,
-1.3885155790598));
#84755=CARTESIAN_POINT('Ctrl Pts',(0.229105382710018,-0.185309478845056,
-1.38941392420587));
#84756=CARTESIAN_POINT('Ctrl Pts',(0.217962411488752,-0.197600676056556,
-1.39031226935195));
#84757=CARTESIAN_POINT('Ctrl Pts',(0.206841015525056,-0.209868074790934,
-1.39120887510306));
#84758=CARTESIAN_POINT('Ctrl Pts',(0.194657672567564,-0.221219107756348,
-1.39210548085418));
#84759=CARTESIAN_POINT('Ctrl Pts',(0.181589935508457,-0.231470808790298,
-1.3930020866053));
#84760=CARTESIAN_POINT('Ctrl Pts',(0.168524443573054,-0.241720748514168,
-1.39389853831362));
#84761=CARTESIAN_POINT('Ctrl Pts',(0.154575447180179,-0.250871203132498,
-1.39479499002194));
#84762=CARTESIAN_POINT('Ctrl Pts',(0.139954765137329,-0.25877848387251,
-1.39569144173025));
#84763=CARTESIAN_POINT('Ctrl Pts',(0.125337934993483,-0.266683681395972,
-1.39658765726344));
#84764=CARTESIAN_POINT('Ctrl Pts',(0.110050471734688,-0.273345988513023,
-1.39748387279663));
#84765=CARTESIAN_POINT('Ctrl Pts',(0.0943286970484332,-0.278667789514944,
-1.39838008832982));
#84766=CARTESIAN_POINT('Ctrl Pts',(0.0785694116177297,-0.284002287856787,
-1.3992784421529));
#84767=CARTESIAN_POINT('Ctrl Pts',(0.06237450618845,-0.28798966286102,-1.40017679597598));
#84768=CARTESIAN_POINT('Ctrl Pts',(0.0459957532466042,-0.29058222706022,
-1.40107514979906));
#84769=CARTESIAN_POINT('Ctrl Pts',(0.0314320344127203,-0.292887492680259,
-1.40187395130361));
#84770=CARTESIAN_POINT('Ctrl Pts',(0.0167235182312306,-0.294090670138664,
-1.40267275280817));
#84771=CARTESIAN_POINT('Ctrl Pts',(0.00204878209681707,-0.294192866147226,
-1.40347155431272));
#84772=CARTESIAN_POINT('Ctrl Pts',(-0.0144547871297883,-0.294307798292277,
-1.4043699061337));
#84773=CARTESIAN_POINT('Ctrl Pts',(-0.0310205105826716,-0.29303005215292,
-1.40526825795467));
#84774=CARTESIAN_POINT('Ctrl Pts',(-0.0473942850564051,-0.290357403459929,
-1.40616660977565));
#84775=CARTESIAN_POINT('Ctrl Pts',(-0.0637363587694816,-0.28768992919979,
-1.40706322232532));
#84776=CARTESIAN_POINT('Ctrl Pts',(-0.079886438858722,-0.283632974159542,
-1.407959834875));
#84777=CARTESIAN_POINT('Ctrl Pts',(-0.0955944370975883,-0.278236129206822,
-1.40885644742467));
#84778=CARTESIAN_POINT('Ctrl Pts',(-0.11129973813358,-0.272840210940335,
-1.409752906018));
#84779=CARTESIAN_POINT('Ctrl Pts',(-0.126562345130107,-0.266105066013107,
-1.41064936461133));
#84780=CARTESIAN_POINT('Ctrl Pts',(-0.141146514708509,-0.258130396090117,
-1.41154582320467));
#84781=CARTESIAN_POINT('Ctrl Pts',(-0.155726843005352,-0.250157826591999,
-1.4124420456824));
#84782=CARTESIAN_POINT('Ctrl Pts',(-0.16962839967055,-0.24094676949677,
-1.41333826816014));
#84783=CARTESIAN_POINT('Ctrl Pts',(-0.182640796697551,-0.23064253593317,
-1.41423449063788));
#84784=CARTESIAN_POINT('Ctrl Pts',(-0.195684239174444,-0.220313718154525,
-1.41513285135579));
#84785=CARTESIAN_POINT('Ctrl Pts',(-0.207833678909567,-0.208887028931223,
-1.4160312120737));
#84786=CARTESIAN_POINT('Ctrl Pts',(-0.218912239215287,-0.196547886078048,
-1.4169295727916));
#84787=CARTESIAN_POINT('Ctrl Pts',(-0.22876261624213,-0.185576676287448,
-1.4177283400983));
#84788=CARTESIAN_POINT('Ctrl Pts',(-0.237766686379653,-0.173884970186014,
-1.418527107405));
#84789=CARTESIAN_POINT('Ctrl Pts',(-0.245828328475075,-0.16162324374653,
-1.4193258747117));
#84790=CARTESIAN_POINT('Ctrl Pts',(-0.255067937885253,-0.147569833578445,
-1.42024135791427));
#84791=CARTESIAN_POINT('Ctrl Pts',(-0.263125967190795,-0.132680482413092,
-1.42115684111684));
#84792=CARTESIAN_POINT('Ctrl Pts',(-0.269858553853055,-0.11717508656851,
-1.42207232431942));
#84793=CARTESIAN_POINT('Ctrl Pts',(-0.276575724393973,-0.101705194620988,
-1.42298571126971));
#84794=CARTESIAN_POINT('Ctrl Pts',(-0.281973120566162,-0.0856227113463165,
-1.42389909822));
#84795=CARTESIAN_POINT('Ctrl Pts',(-0.285952486678191,-0.0691723598163232,
-1.4248124851703));
#84796=CARTESIAN_POINT('Ctrl Pts',(-0.289925530565836,-0.0527481438090875,
-1.42572442097559));
#84797=CARTESIAN_POINT('Ctrl Pts',(-0.292484803514074,-0.0359579352967791,
-1.42663635678088));
#84798=CARTESIAN_POINT('Ctrl Pts',(-0.293581844870242,-0.0190614889918173,
-1.42754829258617));
#84799=CARTESIAN_POINT('Ctrl Pts',(-0.293996510664294,-0.0126748762316724,
-1.42789299115446));
#84800=CARTESIAN_POINT('Ctrl Pts',(-0.294202784441153,-0.00627319483703169,
-1.42823768972275));
#84801=CARTESIAN_POINT('Ctrl Pts',(-0.294199971607168,0.000129253013507976,
-1.42858238829104));
#84802=CARTESIAN_POINT('Ctrl Pts',(-0.294199971607144,0.000129253068963212,
-1.42858238829403));
#84803=CARTESIAN_POINT('Ctrl Pts',(-0.294191975027856,0.0183307040540321,
-1.4295623281923));
#84804=CARTESIAN_POINT('Ctrl Pts',(-0.29249067779368,0.036476686751396,
-1.43054226809058));
#84805=CARTESIAN_POINT('Ctrl Pts',(-0.289151433169477,0.054268671404759,
-1.43152220798886));
#84806=CARTESIAN_POINT('Ctrl Pts',(-0.285788906561617,0.0721847058785258,
-1.43250898025411));
#84807=CARTESIAN_POINT('Ctrl Pts',(-0.280765736918653,0.0897412935870321,
-1.43349575251937));
#84808=CARTESIAN_POINT('Ctrl Pts',(-0.27418768992192,0.106652476273555,
-1.43448252478462));
#84809=CARTESIAN_POINT('Ctrl Pts',(-0.272637413883995,0.110638005915544,
-1.43471508155998));
#84810=CARTESIAN_POINT('Ctrl Pts',(-0.271000981417167,0.114587788409907,
-1.43494763833534));
#84811=CARTESIAN_POINT('Ctrl Pts',(-0.269280148701361,0.118498276423637,
-1.4351801951107));
#84812=CARTESIAN_POINT('Ctrl Pts',(-0.262632583131113,0.133604466144566,
-1.43607856041884));
#84813=CARTESIAN_POINT('Ctrl Pts',(-0.254688782871077,0.148197549509576,
-1.43697692572698));
#84814=CARTESIAN_POINT('Ctrl Pts',(-0.245550685018537,0.162044750260313,
-1.43787529103512));
#84815=CARTESIAN_POINT('Ctrl Pts',(-0.236430282646639,0.175865136582404,
-1.43877191670267));
#84816=CARTESIAN_POINT('Ctrl Pts',(-0.226120549143635,0.188941818496891,
-1.43966854237023));
#84817=CARTESIAN_POINT('Ctrl Pts',(-0.214769058735139,0.201066882927106,
-1.44056516803778));
#84818=CARTESIAN_POINT('Ctrl Pts',(-0.203419526870608,0.213189855343769,
-1.44146163900487));
#84819=CARTESIAN_POINT('Ctrl Pts',(-0.191029095476835,0.224360924630009,
-1.44235810997196));
#84820=CARTESIAN_POINT('Ctrl Pts',(-0.177785194385758,0.234405769249006,
-1.44325458093905));
#84821=CARTESIAN_POINT('Ctrl Pts',(-0.164544787233774,0.244447963887831,
-1.4441508154037));
#84822=CARTESIAN_POINT('Ctrl Pts',(-0.150451994427785,0.253364054318814,
-1.44504704986835));
#84823=CARTESIAN_POINT('Ctrl Pts',(-0.135725489750741,0.261021515266312,
-1.445943284333));
#84824=CARTESIAN_POINT('Ctrl Pts',(-0.120963864993721,0.268697237888713,
-1.44684165615657));
#84825=CARTESIAN_POINT('Ctrl Pts',(-0.105566227049724,0.275107993319137,
-1.44774002798013));
#84826=CARTESIAN_POINT('Ctrl Pts',(-0.0897741356302365,0.280168243332188,
-1.4486383998037));
#84827=CARTESIAN_POINT('Ctrl Pts',(-0.0757340402459295,0.284667102347404,
-1.44943710503902));
#84828=CARTESIAN_POINT('Ctrl Pts',(-0.0613828225292932,0.288099109861824,
-1.45023581027434));
#84829=CARTESIAN_POINT('Ctrl Pts',(-0.0468970705487783,0.290438125551627,
-1.45103451550967));
#84830=CARTESIAN_POINT('Ctrl Pts',(-0.0306033336238293,0.293069076734849,
-1.4519329081511));
#84831=CARTESIAN_POINT('Ctrl Pts',(-0.0140357636801972,0.294332984452315,
-1.45283130079253));
#84832=CARTESIAN_POINT('Ctrl Pts',(0.00255482522783669,0.294188906772596,
-1.45372969343397));
#84833=CARTESIAN_POINT('Ctrl Pts',(0.0191133046459322,0.294045107941375,
-1.45462634732281));
#84834=CARTESIAN_POINT('Ctrl Pts',(0.0356939321908188,0.292498673935604,
-1.45552300121165));
#84835=CARTESIAN_POINT('Ctrl Pts',(0.0520419624030031,0.289560484440202,
-1.45641965510049));
#84836=CARTESIAN_POINT('Ctrl Pts',(0.0683871888520291,0.286622798857954,
-1.45731615520903));
#84837=CARTESIAN_POINT('Ctrl Pts',(0.0844991117914871,0.282293919412258,
-1.45821265531756));
#84838=CARTESIAN_POINT('Ctrl Pts',(0.100129522321303,0.276636437874167,
-1.45910915542609));
#84839=CARTESIAN_POINT('Ctrl Pts',(0.115755819145252,0.270980445306244,
-1.46000541958831));
#84840=CARTESIAN_POINT('Ctrl Pts',(0.130900114959361,0.263996824445283,
-1.46090168375053));
#84841=CARTESIAN_POINT('Ctrl Pts',(0.145332304362076,0.25579710965687,-1.46179794791275));
#84842=CARTESIAN_POINT('Ctrl Pts',(0.159798915277226,0.24757783812785,-1.462696349711));
#84843=CARTESIAN_POINT('Ctrl Pts',(0.173549350228455,0.238137095384846,
-1.46359475150924));
#84844=CARTESIAN_POINT('Ctrl Pts',(0.186380506412919,0.227631164011573,
-1.46449315330749));
#84845=CARTESIAN_POINT('Ctrl Pts',(0.197785714225321,0.218292774792987,
-1.46529171417455));
#84846=CARTESIAN_POINT('Ctrl Pts',(0.208464774368804,0.208113689555956,
-1.4660902750416));
#84847=CARTESIAN_POINT('Ctrl Pts',(0.218299831790271,0.197227846513467,
-1.46688883590866));
#84848=CARTESIAN_POINT('Ctrl Pts',(0.229361529350384,0.184984308091408,
-1.4677869942433));
#84849=CARTESIAN_POINT('Ctrl Pts',(0.239425231386049,0.171768251619834,
-1.46868515257794));
#84850=CARTESIAN_POINT('Ctrl Pts',(0.248320266062037,0.157767821379643,
-1.46958331091258));
#84851=CARTESIAN_POINT('Ctrl Pts',(0.257198073101548,0.143794506752994,
-1.47047972972108));
#84852=CARTESIAN_POINT('Ctrl Pts',(0.264911230496258,0.129040458772193,
-1.47137614852958));
#84853=CARTESIAN_POINT('Ctrl Pts',(0.271330418485106,0.113725300635774,
-1.47227256733809));
#84854=CARTESIAN_POINT('Ctrl Pts',(0.277748521405541,0.0984127312994287,
-1.4731688346203));
#84855=CARTESIAN_POINT('Ctrl Pts',(0.282872735543824,0.0825399473615452,
-1.47406510190251));
#84856=CARTESIAN_POINT('Ctrl Pts',(0.286620695905337,0.0663492025478846,
-1.47496136918473));
#84857=CARTESIAN_POINT('Ctrl Pts',(0.290367673058947,0.0501627050759085,
-1.47585740134784));
#84858=CARTESIAN_POINT('Ctrl Pts',(0.292738945429468,0.0336591860535186,
-1.47675343351095));
#84859=CARTESIAN_POINT('Ctrl Pts',(0.293703069443292,0.0170923081995552,
-1.47764946567406));
#84860=CARTESIAN_POINT('Ctrl Pts',(0.294669500245366,0.000485792001759425,
-1.47854764170708));
#84861=CARTESIAN_POINT('Ctrl Pts',(0.294222039052706,-0.0161835908076354,
-1.4794458177401));
#84862=CARTESIAN_POINT('Ctrl Pts',(0.292381480914927,-0.0326605207857176,
-1.48034399377313));
#84863=CARTESIAN_POINT('Ctrl Pts',(0.290742678881914,-0.0473313023229251,
-1.48114371461797));
#84864=CARTESIAN_POINT('Ctrl Pts',(0.288000288634847,-0.0618491557389784,
-1.48194343546281));
#84865=CARTESIAN_POINT('Ctrl Pts',(0.284202955405829,-0.0760415684911374,
-1.48274315630765));
#84866=CARTESIAN_POINT('Ctrl Pts',(0.279936370795273,-0.0919877934292838,
-1.48364170179827));
#84867=CARTESIAN_POINT('Ctrl Pts',(0.274309990599236,-0.107624415566617,
-1.4845402472889));
#84868=CARTESIAN_POINT('Ctrl Pts',(0.26738910759261,-0.122705766534535,
-1.48543879277952));
#84869=CARTESIAN_POINT('Ctrl Pts',(0.260481635580393,-0.137757893498329,
-1.48633559710669));
#84870=CARTESIAN_POINT('Ctrl Pts',(0.252284906269277,-0.15225614735143,
-1.48723240143386));
#84871=CARTESIAN_POINT('Ctrl Pts',(0.242913105765234,-0.16597247677699,
-1.48812920576104));
#84872=CARTESIAN_POINT('Ctrl Pts',(0.233542972951434,-0.179686365413423,
-1.48902585050395));
#84873=CARTESIAN_POINT('Ctrl Pts',(0.222998585385343,-0.192617925420461,
-1.48992249524687));
#84874=CARTESIAN_POINT('Ctrl Pts',(0.211438639738649,-0.204566227969012,
-1.49081913998978));
#84875=CARTESIAN_POINT('Ctrl Pts',(0.199881773859228,-0.216511347285368,
-1.4917155458512));
#84876=CARTESIAN_POINT('Ctrl Pts',(0.18731044474944,-0.227473168339034,
-1.49261195171261));
#84877=CARTESIAN_POINT('Ctrl Pts',(0.173920604502344,-0.237287301239529,
-1.49350835757403));
#84878=CARTESIAN_POINT('Ctrl Pts',(0.160498949731181,-0.247124752713033,
-1.49440689331342));
#84879=CARTESIAN_POINT('Ctrl Pts',(0.146255555677053,-0.255808621693674,
-1.49530542905282));
#84880=CARTESIAN_POINT('Ctrl Pts',(0.131416162592098,-0.263217461824947,
-1.49620396479221));
#84881=CARTESIAN_POINT('Ctrl Pts',(0.118239812598643,-0.269795997082846,
-1.49700180209702));
#84882=CARTESIAN_POINT('Ctrl Pts',(0.104594314999241,-0.275369792109794,
-1.49779963940182));
#84883=CARTESIAN_POINT('Ctrl Pts',(0.0906495987568348,-0.279886209458817,
-1.49859747670663));
#84884=CARTESIAN_POINT('Ctrl Pts',(0.0749437793531616,-0.284973013234692,
-1.49949607431199));
#84885=CARTESIAN_POINT('Ctrl Pts',(0.0587587944839904,-0.288749790801653,
-1.50039467191734));
#84886=CARTESIAN_POINT('Ctrl Pts',(0.0423364127233751,-0.291137885129565,
-1.5012932695227));
#84887=CARTESIAN_POINT('Ctrl Pts',(0.0259457377144457,-0.293521368755147,
-1.50219013220242));
#84888=CARTESIAN_POINT('Ctrl Pts',(0.00931933957586975,-0.294521314058951,
-1.50308699488214));
#84889=CARTESIAN_POINT('Ctrl Pts',(-0.00728924515587781,-0.294109685160243,
-1.50398385756186));
#84890=CARTESIAN_POINT('Ctrl Pts',(-0.0238950319068033,-0.293698125606984,
-1.50488056915077));
#84891=CARTESIAN_POINT('Ctrl Pts',(-0.0404822220529669,-0.291875431161071,
-1.50577728073968));
#84892=CARTESIAN_POINT('Ctrl Pts',(-0.0567958683189227,-0.2886656705289,
-1.50667399232858));
#84893=CARTESIAN_POINT('Ctrl Pts',(-0.0731052556088385,-0.28545674786351,
-1.50757046981451));
#84894=CARTESIAN_POINT('Ctrl Pts',(-0.0891404670749405,-0.280861641434708,
-1.50846694730044));
#84895=CARTESIAN_POINT('Ctrl Pts',(-0.104656992795962,-0.274955548878189,
-1.50936342478637));
#84896=CARTESIAN_POINT('Ctrl Pts',(-0.120210491283834,-0.269035383288374,
-1.51026203839824));
#84897=CARTESIAN_POINT('Ctrl Pts',(-0.135242103164361,-0.261798299921929,
-1.5111606520101));
#84898=CARTESIAN_POINT('Ctrl Pts',(-0.14952718619918,-0.25336783652894,
-1.51205926562197));
#84899=CARTESIAN_POINT('Ctrl Pts',(-0.162205052954496,-0.245885885509028,
-1.51285677611652));
#84900=CARTESIAN_POINT('Ctrl Pts',(-0.174294954879084,-0.237464895427554,
-1.51365428661107));
#84901=CARTESIAN_POINT('Ctrl Pts',(-0.18566054981683,-0.228218755236533,
-1.51445179710562));
#84902=CARTESIAN_POINT('Ctrl Pts',(-0.198280146566755,-0.217952459337103,
-1.51533729943965));
#84903=CARTESIAN_POINT('Ctrl Pts',(-0.210091389466563,-0.206598751621239,
-1.51622280177368));
#84904=CARTESIAN_POINT('Ctrl Pts',(-0.220899703879849,-0.194311504615128,
-1.51710830410771));
#84905=CARTESIAN_POINT('Ctrl Pts',(-0.231686991578213,-0.182048161469517,
-1.51799208376748));
#84906=CARTESIAN_POINT('Ctrl Pts',(-0.241474635807838,-0.16885543968172,
-1.51887586342724));
#84907=CARTESIAN_POINT('Ctrl Pts',(-0.250103755820896,-0.154924986119999,
-1.519759643087));
#84908=CARTESIAN_POINT('Ctrl Pts',(-0.258730243958732,-0.14099878133631,
-1.52064315319462));
#84909=CARTESIAN_POINT('Ctrl Pts',(-0.266198441486775,-0.126335957832702,
-1.52152666330224));
#84910=CARTESIAN_POINT('Ctrl Pts',(-0.272392376581496,-0.111157695101528,
-1.52241017340986));
#84911=CARTESIAN_POINT('Ctrl Pts',(-0.278585354724032,-0.0959817773855132,
-1.5232935470167));
#84912=CARTESIAN_POINT('Ctrl Pts',(-0.283504171834539,-0.0802913404046116,
-1.52417692062355));
#84913=CARTESIAN_POINT('Ctrl Pts',(-0.287081432566884,-0.0643264414945037,
-1.5250602942304));
#84914=CARTESIAN_POINT('Ctrl Pts',(-0.290665314592038,-0.0483319925240926,
-1.52594530290825));
#84915=CARTESIAN_POINT('Ctrl Pts',(-0.292902560389337,-0.03206287409932,
-1.52683031158611));
#84916=CARTESIAN_POINT('Ctrl Pts',(-0.293777160082763,-0.0157676952566583,
-1.52771532026396));
#84917=CARTESIAN_POINT('Ctrl Pts',(-0.294062783432995,-0.010446079426391,
-1.52800434293965));
#84918=CARTESIAN_POINT('Ctrl Pts',(-0.294203493231576,-0.00512168939691457,
-1.52829336561535));
#84919=CARTESIAN_POINT('Ctrl Pts',(-0.294199934127337,0.000196874250640231,
-1.52858238829104));
#84920=CARTESIAN_POINT('Origin',(0.,0.,-1.7456589891905));
#84921=CARTESIAN_POINT('',(0.223369910286723,0.0797362138773924,-0.0399999999999999));
#84922=CARTESIAN_POINT('Ctrl Pts',(0.223369910286723,0.0797362138773924,
-0.0399999999999999));
#84923=CARTESIAN_POINT('Ctrl Pts',(0.227755575186804,0.0674503837928969,
-0.040928151436346));
#84924=CARTESIAN_POINT('Ctrl Pts',(0.231120659856154,0.0548222395137741,
-0.0418874595346435));
#84925=CARTESIAN_POINT('Ctrl Pts',(0.235703470079078,0.0293394869896825,
-0.0437732825007175));
#84926=CARTESIAN_POINT('Ctrl Pts',(0.236946521790301,0.0165336719173053,
-0.0446967234098427));
#84927=CARTESIAN_POINT('Ctrl Pts',(0.237212224835647,-0.000548839537223723,
-0.0458846925810193));
#84928=CARTESIAN_POINT('Ctrl Pts',(0.237164551851847,-0.00478749684408978,
-0.0461760565250585));
#84929=CARTESIAN_POINT('Ctrl Pts',(0.236928918585958,-0.0109768834788314,
-0.046596819997762));
#84930=CARTESIAN_POINT('Ctrl Pts',(0.236830362302173,-0.0129299774393764,
-0.0467289136837998));
#84931=CARTESIAN_POINT('Ctrl Pts',(0.236612945991118,-0.0163881962245446,
-0.0469616636857334));
#84932=CARTESIAN_POINT('Ctrl Pts',(0.236503850297288,-0.0178938022358611,
-0.0470626128115884));
#84933=CARTESIAN_POINT('Ctrl Pts',(0.236243868106829,-0.0210618483813991,
-0.0472742652514253));
#84934=CARTESIAN_POINT('Ctrl Pts',(0.23608979020853,-0.0227239492479335,
-0.0473848652555413));
#84935=CARTESIAN_POINT('Ctrl Pts',(0.235631922462022,-0.0271538172966524,
-0.0476785522005319));
#84936=CARTESIAN_POINT('Ctrl Pts',(0.235296915096025,-0.0299181459330282,
-0.0478606820781113));
#84937=CARTESIAN_POINT('Ctrl Pts',(0.233057158499585,-0.0460201208094515,
-0.0489161062639835));
#84938=CARTESIAN_POINT('Ctrl Pts',(0.230067346158123,-0.0591825102383886,
-0.049755013879734));
#84939=CARTESIAN_POINT('Ctrl Pts',(0.222861512307011,-0.0817917434546498,
-0.0512194598399837));
#84940=CARTESIAN_POINT('Ctrl Pts',(0.21911721236422,-0.0913497372539561,
-0.0518470789759478));
#84941=CARTESIAN_POINT('Ctrl Pts',(0.212726646050054,-0.10498791702506,
-0.0527912725392269));
#84942=CARTESIAN_POINT('Ctrl Pts',(0.210555217960102,-0.109277552227489,
-0.0530958286049878));
#84943=CARTESIAN_POINT('Ctrl Pts',(0.206765840337732,-0.116230602600322,
-0.0536068528397998));
#84944=CARTESIAN_POINT('Ctrl Pts',(0.205223021235037,-0.118933490270836,
-0.0538100018954434));
#84945=CARTESIAN_POINT('Ctrl Pts',(0.203031938095021,-0.122602456126231,
-0.0540931017233831));
#84946=CARTESIAN_POINT('Ctrl Pts',(0.20242901099198,-0.123595410554864,
-0.0541704725068926));
#84947=CARTESIAN_POINT('Ctrl Pts',(0.201811785312619,-0.124595281265935,
-0.0542491903685042));
#84948=CARTESIAN_POINT('Ctrl Pts',(0.201804740776483,-0.124606690851416,
-0.0542500887297526));
#84949=CARTESIAN_POINT('Ctrl Pts',(0.201790589978157,-0.124629605648643,
-0.0542518931965488));
#84950=CARTESIAN_POINT('Ctrl Pts',(0.201783483699253,-0.124641110850562,
-0.0542527993031468));
#84951=CARTESIAN_POINT('Ctrl Pts',(0.201769201986442,-0.12466422879518,
-0.0542546202047113));
#84952=CARTESIAN_POINT('Ctrl Pts',(0.201762026534311,-0.124675841525576,
-0.0542555350007778));
#84953=CARTESIAN_POINT('Ctrl Pts',(0.201747598688302,-0.124699187001194,
-0.054257374270399));
#84954=CARTESIAN_POINT('Ctrl Pts',(0.201740346273374,-0.124710919733412,
-0.0542582987452612));
#84955=CARTESIAN_POINT('Ctrl Pts',(0.201725756314585,-0.124734518313683,
-0.0542601584120372));
#84956=CARTESIAN_POINT('Ctrl Pts',(0.201718418747594,-0.124746384146427,
-0.0542610936053595));
#84957=CARTESIAN_POINT('Ctrl Pts',(0.201703649851505,-0.124770262727592,
-0.0542629758048169));
#84958=CARTESIAN_POINT('Ctrl Pts',(0.201696218495876,-0.124782275460077,
-0.0542639228126168));
#84959=CARTESIAN_POINT('Ctrl Pts',(0.201243071185299,-0.125514638557729,
-0.0543216649507409));
#84960=CARTESIAN_POINT('Ctrl Pts',(0.200793507002238,-0.12623258571485,
-0.0543786991883708));
#84961=CARTESIAN_POINT('Ctrl Pts',(0.199847898651101,-0.127724874967505,
-0.0544981783427748));
#84962=CARTESIAN_POINT('Ctrl Pts',(0.19935118134348,-0.128498765387827,
-0.0545606656932554));
#84963=CARTESIAN_POINT('Ctrl Pts',(0.198013518471803,-0.130556433814375,
-0.0547281802793283));
#84964=CARTESIAN_POINT('Ctrl Pts',(0.197164607935789,-0.131834945972515,
-0.054833698192417));
#84965=CARTESIAN_POINT('Ctrl Pts',(0.193008892955007,-0.137963794258743,
-0.0553461529099942));
#84966=CARTESIAN_POINT('Ctrl Pts',(0.189535438439584,-0.142698095821386,
-0.05576220297476));
#84967=CARTESIAN_POINT('Ctrl Pts',(0.177918393812321,-0.157358800030003,
-0.0571051638411923));
#84968=CARTESIAN_POINT('Ctrl Pts',(0.169143058456079,-0.166755416962442,
-0.0580489718136488));
#84969=CARTESIAN_POINT('Ctrl Pts',(0.151594553358339,-0.182728602446552,
-0.0597692792142245));
#84970=CARTESIAN_POINT('Ctrl Pts',(0.143042067791329,-0.189498474350884,
-0.0605477119705698));
#84971=CARTESIAN_POINT('Ctrl Pts',(0.130695912675107,-0.197957377281211,
-0.0615872527892901));
#84972=CARTESIAN_POINT('Ctrl Pts',(0.127279627262982,-0.200171038878033,
-0.0618668771674415));
#84973=CARTESIAN_POINT('Ctrl Pts',(0.122177258488858,-0.20329376025142,
-0.0622731376752819));
#84974=CARTESIAN_POINT('Ctrl Pts',(0.120534598112089,-0.204271991413951,
-0.0624022531823423));
#84975=CARTESIAN_POINT('Ctrl Pts',(0.117591734899885,-0.205976653643895,
-0.0626306639199171));
#84976=CARTESIAN_POINT('Ctrl Pts',(0.116296197972131,-0.206710891036716,
-0.0627302345586643));
#84977=CARTESIAN_POINT('Ctrl Pts',(0.113542477274176,-0.208237461003023,
-0.0629398516207759));
#84978=CARTESIAN_POINT('Ctrl Pts',(0.112082714370279,-0.209026791786239,
-0.0630497878355391));
#84979=CARTESIAN_POINT('Ctrl Pts',(0.108141162077503,-0.211104924661254,
-0.0633435605812183));
#84980=CARTESIAN_POINT('Ctrl Pts',(0.105644617103683,-0.212365289296648,
-0.0635264032803257));
#84981=CARTESIAN_POINT('Ctrl Pts',(0.0900633192796194,-0.219888614679257,
-0.0646489582964317));
#84982=CARTESIAN_POINT('Ctrl Pts',(0.0764485973721632,-0.22498465108704,
-0.06554716703907));
#84983=CARTESIAN_POINT('Ctrl Pts',(0.0506837805438242,-0.232017117908173,
-0.0671866412882708));
#84984=CARTESIAN_POINT('Ctrl Pts',(0.0386861121709244,-0.234316312254402,
-0.0679284520800586));
#84985=CARTESIAN_POINT('Ctrl Pts',(0.0228676245380731,-0.236099348823575,
-0.068933787660448));
#84986=CARTESIAN_POINT('Ctrl Pts',(0.0191603640519138,-0.236429076493693,
-0.0691713979761933));
#84987=CARTESIAN_POINT('Ctrl Pts',(0.0128708064886722,-0.236839583852149,
-0.0695801684717117));
#84988=CARTESIAN_POINT('Ctrl Pts',(0.0102920760984747,-0.236965647261717,
-0.0697493700725626));
#84989=CARTESIAN_POINT('Ctrl Pts',(0.00658976627498104,-0.237086094478279,
-0.0699952507444404));
#84990=CARTESIAN_POINT('Ctrl Pts',(0.00546738311595209,-0.23711463221513,
-0.070070180856495));
#84991=CARTESIAN_POINT('Ctrl Pts',(0.00351078517608979,-0.237150481635207,
-0.0702015475009433));
#84992=CARTESIAN_POINT('Ctrl Pts',(0.00267666438307106,-0.237161362786392,
-0.0702577877255202));
#84993=CARTESIAN_POINT('Ctrl Pts',(0.000882804323840761,-0.237175298701457,
-0.0703792716987969));
#84994=CARTESIAN_POINT('Ctrl Pts',(-7.68863340875269E-5,-0.237176929030061,
-0.0704445873827406));
#84995=CARTESIAN_POINT('Ctrl Pts',(-0.0027429472510075,-0.23716527728665,
-0.0706268865926895));
#84996=CARTESIAN_POINT('Ctrl Pts',(-0.0044491645413205,-0.237139404200317,
-0.0707445205617118));
#84997=CARTESIAN_POINT('Ctrl Pts',(-0.0161885180090893,-0.236834655441247,
-0.0715598674649074));
#84998=CARTESIAN_POINT('Ctrl Pts',(-0.0261944222053511,-0.235937554081915,
-0.0722845079809336));
#84999=CARTESIAN_POINT('Ctrl Pts',(-0.0383371644445804,-0.234066893115663,
-0.0731794300146716));
#85000=CARTESIAN_POINT('Ctrl Pts',(-0.0405571327612126,-0.233692463477712,
-0.0733437078865619));
#85001=CARTESIAN_POINT('Ctrl Pts',(-0.0523670548376334,-0.231527198235096,
-0.0742203929345932));
#85002=CARTESIAN_POINT('Ctrl Pts',(-0.0618455126808292,-0.229177450263697,
-0.0749331806921317));
#85003=CARTESIAN_POINT('Ctrl Pts',(-0.0806233994391151,-0.223272061809617,
-0.0763472186036685));
#85004=CARTESIAN_POINT('Ctrl Pts',(-0.0898987652493098,-0.219701628220547,
-0.0770466322226461));
#85005=CARTESIAN_POINT('Ctrl Pts',(-0.101257323179697,-0.214488986516255,
-0.0779027805130789));
#85006=CARTESIAN_POINT('Ctrl Pts',(-0.103573042032291,-0.213380403749465,
-0.0780773488717331));
#85007=CARTESIAN_POINT('Ctrl Pts',(-0.107299926305311,-0.211521295718243,
-0.0783584354956205));
#85008=CARTESIAN_POINT('Ctrl Pts',(-0.108722253252174,-0.210793748941424,
-0.078465743405674));
#85009=CARTESIAN_POINT('Ctrl Pts',(-0.111449490585185,-0.209363768099226,
-0.0786716095187473));
#85010=CARTESIAN_POINT('Ctrl Pts',(-0.112755377140241,-0.208663368710152,
-0.0787702335327048));
#85011=CARTESIAN_POINT('Ctrl Pts',(-0.115754579455062,-0.207018397876951,
-0.0789969047242206));
#85012=CARTESIAN_POINT('Ctrl Pts',(-0.117443063077325,-0.206065200924031,
-0.0791246369939908));
#85013=CARTESIAN_POINT('Ctrl Pts',(-0.122947178955313,-0.20286833966744,
-0.0795416118550793));
#85014=CARTESIAN_POINT('Ctrl Pts',(-0.126711846404028,-0.200538485245224,
-0.0798277403004468));
#85015=CARTESIAN_POINT('Ctrl Pts',(-0.145622837675745,-0.188089655647993,
-0.0812745292420112));
#85016=CARTESIAN_POINT('Ctrl Pts',(-0.159631916097633,-0.176355953255343,
-0.0823726212208167));
#85017=CARTESIAN_POINT('Ctrl Pts',(-0.177278096616715,-0.157733356860707,
-0.0839520793447804));
#85018=CARTESIAN_POINT('Ctrl Pts',(-0.182138231918799,-0.152095312609701,
-0.0844139482852281));
#85019=CARTESIAN_POINT('Ctrl Pts',(-0.189286628847751,-0.142967872773016,
-0.0851534698077213));
#85020=CARTESIAN_POINT('Ctrl Pts',(-0.191761668395135,-0.139630576981363,
-0.0854223063960954));
#85021=CARTESIAN_POINT('Ctrl Pts',(-0.194914621004483,-0.135137168462202,
-0.0857847843149075));
#85022=CARTESIAN_POINT('Ctrl Pts',(-0.19567236056301,-0.134037647268601,
-0.0858735208550365));
#85023=CARTESIAN_POINT('Ctrl Pts',(-0.196907283132061,-0.132212919195767,
-0.0860209554798516));
#85024=CARTESIAN_POINT('Ctrl Pts',(-0.197389856318338,-0.131491363752863,
-0.0860792994661674));
#85025=CARTESIAN_POINT('Ctrl Pts',(-0.198296430181172,-0.130119594743281,
-0.0861903331526911));
#85026=CARTESIAN_POINT('Ctrl Pts',(-0.198721217770172,-0.129469922076962,
-0.0862429651524551));
#85027=CARTESIAN_POINT('Ctrl Pts',(-0.199839652964633,-0.127740909111082,
-0.086383135483864));
#85028=CARTESIAN_POINT('Ctrl Pts',(-0.200527732722454,-0.126658023751571,
-0.0864710247082619));
#85029=CARTESIAN_POINT('Ctrl Pts',(-0.203002791940602,-0.122692103540876,
-0.0867931198186491));
#85030=CARTESIAN_POINT('Ctrl Pts',(-0.204736565585314,-0.119776548835057,
-0.0870303112116316));
#85031=CARTESIAN_POINT('Ctrl Pts',(-0.213696265236722,-0.103946498853728,
-0.0883163554729566));
#85032=CARTESIAN_POINT('Ctrl Pts',(-0.219763748477631,-0.0904147503945695,
-0.0894070699715227));
#85033=CARTESIAN_POINT('Ctrl Pts',(-0.228423049350878,-0.0649682780140882,
-0.0913620129888713));
#85034=CARTESIAN_POINT('Ctrl Pts',(-0.23143616194505,-0.0532479326507539,
-0.0922287017789436));
#85035=CARTESIAN_POINT('Ctrl Pts',(-0.234261466371192,-0.0372897763053309,
-0.0933548781232203));
#85036=CARTESIAN_POINT('Ctrl Pts',(-0.234874029562119,-0.0332137915015895,
-0.0936380657761215));
#85037=CARTESIAN_POINT('Ctrl Pts',(-0.235615636658183,-0.0272200597254118,
-0.0940482315604449));
#85038=CARTESIAN_POINT('Ctrl Pts',(-0.235828076924721,-0.0253136010403289,
-0.0941777761363258));
#85039=CARTESIAN_POINT('Ctrl Pts',(-0.236164071525444,-0.0219253723326297,
-0.0944064383914506));
#85040=CARTESIAN_POINT('Ctrl Pts',(-0.236296862671317,-0.0204446446661825,
-0.0945058385743478));
#85041=CARTESIAN_POINT('Ctrl Pts',(-0.236547571661388,-0.0173189593859044,
-0.0947145890644771));
#85042=CARTESIAN_POINT('Ctrl Pts',(-0.236662273466589,-0.0156738176972949,
-0.0948238343004504));
#85043=CARTESIAN_POINT('Ctrl Pts',(-0.236923075804442,-0.0112719521688186,
-0.095114553972766));
#85044=CARTESIAN_POINT('Ctrl Pts',(-0.237038225682992,-0.00851359785458927,
-0.0952950661872727));
#85045=CARTESIAN_POINT('Ctrl Pts',(-0.237406034895552,0.0066433410101141,
-0.096278896824417));
#85046=CARTESIAN_POINT('Ctrl Pts',(-0.236734189313708,0.0190457176630952,
-0.0970529493503612));
#85047=CARTESIAN_POINT('Ctrl Pts',(-0.232800798207848,0.0485518444689856,
-0.0988874096047161));
#85048=CARTESIAN_POINT('Ctrl Pts',(-0.228623424655103,0.0654574093770121,
-0.0999317714500581));
#85049=CARTESIAN_POINT('Ctrl Pts',(-0.221655485484241,0.0844332701974654,
-0.101238640282909));
#85050=CARTESIAN_POINT('Ctrl Pts',(-0.220623138636862,0.0870951221952471,
-0.101425287275785));
#85051=CARTESIAN_POINT('Ctrl Pts',(-0.219100372267507,0.0908205726181262,
-0.101692106218462));
#85052=CARTESIAN_POINT('Ctrl Pts',(-0.218649692287981,0.0919002799766883,
-0.101770106907023));
#85053=CARTESIAN_POINT('Ctrl Pts',(-0.217860194909153,0.0937530182021312,
-0.101905186248613));
#85054=CARTESIAN_POINT('Ctrl Pts',(-0.217525199342231,0.0945276709645965,
-0.101962039591995));
#85055=CARTESIAN_POINT('Ctrl Pts',(-0.216806517994463,0.0961655170133428,
-0.102083067720244));
#85056=CARTESIAN_POINT('Ctrl Pts',(-0.216421804597607,0.0970282192153031,
-0.102147299890636));
#85057=CARTESIAN_POINT('Ctrl Pts',(-0.215345578569769,0.0994033605387357,
-0.102325431172351));
#85058=CARTESIAN_POINT('Ctrl Pts',(-0.214643311330578,0.100910826018539,
-0.102439941787794));
#85059=CARTESIAN_POINT('Ctrl Pts',(-0.210622799138623,0.109309254525945,
-0.10308558382786));
#85060=CARTESIAN_POINT('Ctrl Pts',(-0.206988889152257,0.116043320881076,
-0.103632301245098));
#85061=CARTESIAN_POINT('Ctrl Pts',(-0.191690828878982,0.141380468971707,
-0.105774192769637));
#85062=CARTESIAN_POINT('Ctrl Pts',(-0.177788199330129,0.158510317670842,
-0.107395176475848));
#85063=CARTESIAN_POINT('Ctrl Pts',(-0.158770679954309,0.176238984353413,
-0.109200792951285));
#85064=CARTESIAN_POINT('Ctrl Pts',(-0.155744950341185,0.178918479550083,
-0.109478360597535));
#85065=CARTESIAN_POINT('Ctrl Pts',(-0.151196967155293,0.182743187188463,
-0.109881851380408));
#85066=CARTESIAN_POINT('Ctrl Pts',(-0.149727174977946,0.183949364715039,
-0.110010231779461));
#85067=CARTESIAN_POINT('Ctrl Pts',(-0.147086283895167,0.186063971681287,
-0.110237406491457));
#85068=CARTESIAN_POINT('Ctrl Pts',(-0.145920891178292,0.186979330827736,
-0.110336474111621));
#85069=CARTESIAN_POINT('Ctrl Pts',(-0.143438167322815,0.188892039134169,
-0.110545086270585));
#85070=CARTESIAN_POINT('Ctrl Pts',(-0.142118834418132,0.18988666996184,
-0.110654520695018));
#85071=CARTESIAN_POINT('Ctrl Pts',(-0.138547331954141,0.192521110336148,
-0.110947061476491));
#85072=CARTESIAN_POINT('Ctrl Pts',(-0.136276443313954,0.194135193035347,
-0.111129177257946));
#85073=CARTESIAN_POINT('Ctrl Pts',(-0.12244291154887,0.203605290862651,
-0.112216623359398));
#85074=CARTESIAN_POINT('Ctrl Pts',(-0.110232151627088,0.21046692268304,
-0.113083636319488));
#85075=CARTESIAN_POINT('Ctrl Pts',(-0.088131630129975,0.220431632362591,
-0.114572690029515));
#85076=CARTESIAN_POINT('Ctrl Pts',(-0.0785130769470917,0.224037876441566,
-0.11519760097848));
#85077=CARTESIAN_POINT('Ctrl Pts',(-0.061436611666013,0.22920510102654,
-0.116310526852575));
#85078=CARTESIAN_POINT('Ctrl Pts',(-0.0540812627729639,0.231051136994762,
-0.116791140588702));
#85079=CARTESIAN_POINT('Ctrl Pts',(-0.0450823060151138,0.232856449867392,
-0.117394376773371));
#85080=CARTESIAN_POINT('Ctrl Pts',(-0.0435104905522345,0.233155264635116,
-0.117500298996737));
#85081=CARTESIAN_POINT('Ctrl Pts',(-0.0419358257166351,0.233438144154857,
-0.117607078812657));
#85082=CARTESIAN_POINT('',(0.150502666328434,-0.183305559252938,-0.04));
#85083=CARTESIAN_POINT('Origin',(0.,0.,-0.04));
#85084=CARTESIAN_POINT('',(-0.237174908959558,-0.00020781006993565,-0.0759410108041934));
#85085=CARTESIAN_POINT('Ctrl Pts',(-0.237174908959558,-0.00020781006993565,
-0.0759410108041934));
#85086=CARTESIAN_POINT('Ctrl Pts',(-0.237158965686875,-0.0184039650893944,
-0.0747207381634765));
#85087=CARTESIAN_POINT('Ctrl Pts',(-0.235045118479419,-0.0365055894439177,
-0.073500465522759));
#85088=CARTESIAN_POINT('Ctrl Pts',(-0.230920381200416,-0.0541087624258259,
-0.0722801928820409));
#85089=CARTESIAN_POINT('Ctrl Pts',(-0.230276398834125,-0.0568570909190921,
-0.0720896755206831));
#85090=CARTESIAN_POINT('Ctrl Pts',(-0.229583492057616,-0.0595933149141058,
-0.0718991581593253));
#85091=CARTESIAN_POINT('Ctrl Pts',(-0.228842093394929,-0.0623159443130459,
-0.0717086407979675));
#85092=CARTESIAN_POINT('Ctrl Pts',(-0.225192493135875,-0.0757183274838922,
-0.0707708022957423));
#85093=CARTESIAN_POINT('Ctrl Pts',(-0.220347559650889,-0.0888495540733388,
-0.0698329637935173));
#85094=CARTESIAN_POINT('Ctrl Pts',(-0.214367883493431,-0.101480989113956,
-0.0688951252912922));
#85095=CARTESIAN_POINT('Ctrl Pts',(-0.208400359824408,-0.114086753304811,
-0.0679591927570915));
#85096=CARTESIAN_POINT('Ctrl Pts',(-0.201302959780381,-0.126193945435919,
-0.0670232602228907));
#85097=CARTESIAN_POINT('Ctrl Pts',(-0.193185046329708,-0.137591854771962,
-0.06608732768869));
#85098=CARTESIAN_POINT('Ctrl Pts',(-0.185067115835033,-0.148989788038536,
-0.0651513931894479));
#85099=CARTESIAN_POINT('Ctrl Pts',(-0.175929117518454,-0.159677709738982,
-0.0642154586902058));
#85100=CARTESIAN_POINT('Ctrl Pts',(-0.165924297051288,-0.169473031108303,
-0.0632795241909636));
#85101=CARTESIAN_POINT('Ctrl Pts',(-0.155920418675126,-0.179267430113833,
-0.0623436778227854));
#85102=CARTESIAN_POINT('Ctrl Pts',(-0.145050507587878,-0.188168815215712,
-0.0614078314546073));
#85103=CARTESIAN_POINT('Ctrl Pts',(-0.133503529137789,-0.196032620583299,
-0.060471985086429));
#85104=CARTESIAN_POINT('Ctrl Pts',(-0.121925774218444,-0.20391738556081,
-0.0595336443819963));
#85105=CARTESIAN_POINT('Ctrl Pts',(-0.109668087105897,-0.210758613379555,
-0.0585953036775631));
#85106=CARTESIAN_POINT('Ctrl Pts',(-0.0969465426444049,-0.216456343160224,
-0.0576569629731303));
#85107=CARTESIAN_POINT('Ctrl Pts',(-0.0888001065838006,-0.220104971790916,
-0.0570560821150817));
#85108=CARTESIAN_POINT('Ctrl Pts',(-0.0804639467507705,-0.223285648539055,
-0.0564552012570333));
#85109=CARTESIAN_POINT('Ctrl Pts',(-0.0719980238660825,-0.225982886928146,
-0.0558543203989847));
#85110=CARTESIAN_POINT('Ctrl Pts',(-0.0582706547715472,-0.230356419194777,
-0.0548800009499861));
#85111=CARTESIAN_POINT('Ctrl Pts',(-0.0441059425071512,-0.233486976078622,
-0.0539056815009878));
#85112=CARTESIAN_POINT('Ctrl Pts',(-0.0297453723807863,-0.235302344754421,
-0.0529313620519891));
#85113=CARTESIAN_POINT('Ctrl Pts',(-0.0154188776396131,-0.237113405844493,
-0.0519593545105423));
#85114=CARTESIAN_POINT('Ctrl Pts',(-0.000898203897908545,-0.237615317219415,
-0.0509873469690956));
#85115=CARTESIAN_POINT('Ctrl Pts',(0.0135648054651533,-0.236786774710271,
-0.0500153394276488));
#85116=CARTESIAN_POINT('Ctrl Pts',(0.02800928492293,-0.235959293723928,
-0.0490445772153881));
#85117=CARTESIAN_POINT('Ctrl Pts',(0.0423954714960833,-0.23380474552208,
-0.0480738150031273));
#85118=CARTESIAN_POINT('Ctrl Pts',(0.0564719007170983,-0.230353869197802,
-0.0471030527908667));
#85119=CARTESIAN_POINT('Ctrl Pts',(0.070536700396345,-0.226905843888489,
-0.0461330925944807));
#85120=CARTESIAN_POINT('Ctrl Pts',(0.0842914947997221,-0.222163793119845,
-0.0451631323980948));
#85121=CARTESIAN_POINT('Ctrl Pts',(0.0974964044458938,-0.216209231405883,
-0.0441931722017088));
#85122=CARTESIAN_POINT('Ctrl Pts',(0.110710507203386,-0.210250524192242,
-0.0432225367298155));
#85123=CARTESIAN_POINT('Ctrl Pts',(0.123373253112856,-0.20307794391354,
-0.0422519012579224));
#85124=CARTESIAN_POINT('Ctrl Pts',(0.13526628678023,-0.194820461670966,
-0.0412812657860291));
#85125=CARTESIAN_POINT('Ctrl Pts',(0.140499331718777,-0.191187093023135,
-0.0408541771906861));
#85126=CARTESIAN_POINT('Ctrl Pts',(0.145583704196375,-0.187344263367862,
-0.040427088595343));
#85127=CARTESIAN_POINT('Ctrl Pts',(0.150502666328434,-0.183305559252938,
-0.04));
#85128=CARTESIAN_POINT('Ctrl Pts',(-0.237174909590924,-0.000207088234899032,
-0.0759292533346744));
#85129=CARTESIAN_POINT('Ctrl Pts',(-0.237183607200531,0.00975414772469391,
-0.0765408113412823));
#85130=CARTESIAN_POINT('Ctrl Pts',(-0.236564747866873,0.0197057060827421,
-0.077155976177345));
#85131=CARTESIAN_POINT('Ctrl Pts',(-0.234739333942387,0.0342235074390107,
-0.0780837272251957));
#85132=CARTESIAN_POINT('Ctrl Pts',(-0.234019769798396,0.0388400093584547,
-0.0783832186704287));
#85133=CARTESIAN_POINT('Ctrl Pts',(-0.232806910733985,0.0453512298203194,
-0.0788136472548088));
#85134=CARTESIAN_POINT('Ctrl Pts',(-0.232425745196628,0.0472658898231393,
-0.0789412059275054));
#85135=CARTESIAN_POINT('Ctrl Pts',(-0.231713367225553,0.050627042651014,
-0.0791669932979334));
#85136=CARTESIAN_POINT('Ctrl Pts',(-0.23139213085097,0.0520755567847521,
-0.0792649100086293));
#85137=CARTESIAN_POINT('Ctrl Pts',(-0.23071500242883,0.0549988144949174,
-0.0794638062127938));
#85138=CARTESIAN_POINT('Ctrl Pts',(-0.230358509626961,0.056473345965148,
-0.0795648003562512));
#85139=CARTESIAN_POINT('Ctrl Pts',(-0.22958603411431,0.0595393928033083,
-0.0797762429485215));
#85140=CARTESIAN_POINT('Ctrl Pts',(-0.229167591361299,0.0611301987051148,
-0.0798867644607751));
#85141=CARTESIAN_POINT('Ctrl Pts',(-0.228027033146246,0.0652899164515071,
-0.080177964494201));
#85142=CARTESIAN_POINT('Ctrl Pts',(-0.22727806844499,0.0678511580749889,
-0.0803594829370441));
#85143=CARTESIAN_POINT('Ctrl Pts',(-0.223510081125561,0.0799734192171112,
-0.0812295129399832));
#85144=CARTESIAN_POINT('Ctrl Pts',(-0.219930375181725,0.0893481279248556,
-0.081935521199564));
#85145=CARTESIAN_POINT('Ctrl Pts',(-0.209494610383567,0.112215753794183,
-0.0837381847953898));
#85146=CARTESIAN_POINT('Ctrl Pts',(-0.201921125851801,0.125332348903381,
-0.0848487718477774));
#85147=CARTESIAN_POINT('Ctrl Pts',(-0.190029821487688,0.142019658077279,
-0.0863179540386775));
#85148=CARTESIAN_POINT('Ctrl Pts',(-0.186759756228465,0.146293262151402,
-0.08669947422341));
#85149=CARTESIAN_POINT('Ctrl Pts',(-0.18216687636809,0.151890323565048,
-0.0872027328516464));
#85150=CARTESIAN_POINT('Ctrl Pts',(-0.180969887668527,0.153314518254734,
-0.0873311131371838));
#85151=CARTESIAN_POINT('Ctrl Pts',(-0.179078607620505,0.15551177391918,
-0.0875294977947869));
#85152=CARTESIAN_POINT('Ctrl Pts',(-0.178395812982089,0.156294572983944,
-0.087600239082649));
#85153=CARTESIAN_POINT('Ctrl Pts',(-0.177146057088149,0.157708512009016,
-0.087728094087927));
#85154=CARTESIAN_POINT('Ctrl Pts',(-0.176580824444461,0.158341127997742,
-0.0877853242169888));
#85155=CARTESIAN_POINT('Ctrl Pts',(-0.175288096954773,0.159772434170472,
-0.0879148630181392));
#85156=CARTESIAN_POINT('Ctrl Pts',(-0.174558526178157,0.160569202230658,
-0.0879870193070934));
#85157=CARTESIAN_POINT('Ctrl Pts',(-0.172253464739296,0.163052292630772,
-0.0882121401610231));
#85158=CARTESIAN_POINT('Ctrl Pts',(-0.170658738016339,0.164720679762996,
-0.0883637636735546));
#85159=CARTESIAN_POINT('Ctrl Pts',(-0.161337112849328,0.174192145447494,
-0.0892285400570341));
#85160=CARTESIAN_POINT('Ctrl Pts',(-0.153099188227136,0.181475237755567,
-0.089909831712682));
#85161=CARTESIAN_POINT('Ctrl Pts',(-0.137081351256703,0.19376646526179,
-0.0911527640998902));
#85162=CARTESIAN_POINT('Ctrl Pts',(-0.129457388848606,0.198941001370079,
-0.0917148580242062));
#85163=CARTESIAN_POINT('Ctrl Pts',(-0.11244298369889,0.20909588064915,-0.0929427165481842));
#85164=CARTESIAN_POINT('Ctrl Pts',(-0.102980514660976,0.213914668181631,
-0.0936100598248527));
#85165=CARTESIAN_POINT('Ctrl Pts',(-0.0908108557209554,0.219117045955595,
-0.0944703612258928));
#85166=CARTESIAN_POINT('Ctrl Pts',(-0.0883767057591891,0.220110082306797,
-0.0946424899551439));
#85167=CARTESIAN_POINT('Ctrl Pts',(-0.0844129340528357,0.221650794365439,
-0.0949231338492768));
#85168=CARTESIAN_POINT('Ctrl Pts',(-0.0828932682452703,0.222223589966903,
-0.0950308107466323));
#85169=CARTESIAN_POINT('Ctrl Pts',(-0.0799597677835509,0.223295014301621,
-0.0952388816903031));
#85170=CARTESIAN_POINT('Ctrl Pts',(-0.0785468487422197,0.223795934395491,
-0.0953391942000627));
#85171=CARTESIAN_POINT('Ctrl Pts',(-0.0752836851071221,0.224918110707922,
-0.095571133716558));
#85172=CARTESIAN_POINT('Ctrl Pts',(-0.0734303522955524,0.225529981899466,
-0.0957030606453805));
#85173=CARTESIAN_POINT('Ctrl Pts',(-0.0673601683925233,0.227451278210229,
-0.0961359084387482));
#85174=CARTESIAN_POINT('Ctrl Pts',(-0.0631144862940898,0.22866576782424,
-0.0964398489030841));
#85175=CARTESIAN_POINT('Ctrl Pts',(-0.0532460002596512,0.231192907846172,
-0.0971494803606293));
#85176=CARTESIAN_POINT('Ctrl Pts',(-0.0476082272902688,0.232419130680886,
-0.09755724369748));
#85177=CARTESIAN_POINT('Ctrl Pts',(-0.0419357865133625,0.233438151197497,
-0.0979694843087454));
#85178=CARTESIAN_POINT('Origin',(3.51939854619125E-17,0.,-0.04));
#85179=CARTESIAN_POINT('',(-0.287858644329449,-0.0607539371959678,-0.04));
#85180=CARTESIAN_POINT('Origin',(0.,0.,-0.04));
#85181=CARTESIAN_POINT('Ctrl Pts',(-0.287858644329448,-0.0607539371959718,
-0.0400000000000039));
#85182=CARTESIAN_POINT('Ctrl Pts',(-0.286189983298407,-0.0661913078499225,
-0.0400000000000039));
#85183=CARTESIAN_POINT('Ctrl Pts',(-0.284353083067471,-0.0715709236410684,
-0.040000000000004));
#85184=CARTESIAN_POINT('Ctrl Pts',(-0.282345486243454,-0.076885442432171,
-0.0400000000000038));
#85185=CARTESIAN_POINT('Ctrl Pts',(-0.278227505697077,-0.0877865779257651,
-0.0400000000000036));
#85186=CARTESIAN_POINT('Ctrl Pts',(-0.27339181851782,-0.0984142681665029,
-0.0400000000000037));
#85187=CARTESIAN_POINT('Ctrl Pts',(-0.267892007126804,-0.108722285391854,
-0.0400000000000033));
#85188=CARTESIAN_POINT('Ctrl Pts',(-0.26474927804854,-0.114612542924374,
-0.040000000000003));
#85189=CARTESIAN_POINT('Ctrl Pts',(-0.261388562009413,-0.120399838370053,
-0.0400000000000031));
#85190=CARTESIAN_POINT('Ctrl Pts',(-0.25782193291234,-0.126069559657423,
-0.0400000000000028));
#85191=CARTESIAN_POINT('Ctrl Pts',(-0.252889452406428,-0.133910517873923,
-0.0400000000000024));
#85192=CARTESIAN_POINT('Ctrl Pts',(-0.247573067082612,-0.141511317453255,
-0.0400000000000019));
#85193=CARTESIAN_POINT('Ctrl Pts',(-0.241904248797415,-0.148843967831607,
-0.0400000000000018));
#85194=CARTESIAN_POINT('Ctrl Pts',(-0.236180254585571,-0.156247988601291,
-0.0400000000000017));
#85195=CARTESIAN_POINT('Ctrl Pts',(-0.230095622069276,-0.16338063206386,
-0.0400000000000015));
#85196=CARTESIAN_POINT('Ctrl Pts',(-0.223676361292404,-0.170215298935253,
-0.0400000000000015));
#85197=CARTESIAN_POINT('Ctrl Pts',(-0.219180917476327,-0.17500165393623,
-0.0400000000000015));
#85198=CARTESIAN_POINT('Ctrl Pts',(-0.214519683660013,-0.17964329080041,
-0.0400000000000022));
#85199=CARTESIAN_POINT('Ctrl Pts',(-0.209706358590513,-0.184124977275315,
-0.0400000000000017));
#85200=CARTESIAN_POINT('Ctrl Pts',(-0.205260944507215,-0.18826410186898,
-0.0400000000000013));
#85201=CARTESIAN_POINT('Ctrl Pts',(-0.200692159066689,-0.192260891598814,
-0.0400000000000011));
#85202=CARTESIAN_POINT('Ctrl Pts',(-0.196012274283808,-0.196105089280495,
-0.0400000000000009));
#85203=CARTESIAN_POINT('Ctrl Pts',(-0.183147436316345,-0.206672652924502,
-0.0400000000000005));
#85204=CARTESIAN_POINT('Ctrl Pts',(-0.169432018761062,-0.216101860642565,
-0.0400000000000016));
#85205=CARTESIAN_POINT('Ctrl Pts',(-0.155013008598473,-0.224234519276562,
-0.0400000000000007));
#85206=CARTESIAN_POINT('Ctrl Pts',(-0.145592444993356,-0.229547937262704,
-0.0400000000000001));
#85207=CARTESIAN_POINT('Ctrl Pts',(-0.13587108744713,-0.234307045047568,
-0.0400000000000003));
#85208=CARTESIAN_POINT('Ctrl Pts',(-0.125887328485882,-0.238455560328839,
-0.0400000000000003));
#85209=CARTESIAN_POINT('Ctrl Pts',(-0.120905607334647,-0.240525596915574,
-0.0400000000000003));
#85210=CARTESIAN_POINT('Ctrl Pts',(-0.11585960953477,-0.242442558405335,
-0.04));
#85211=CARTESIAN_POINT('Ctrl Pts',(-0.110772660029015,-0.244193536666844,
-0.04));
#85212=CARTESIAN_POINT('Ctrl Pts',(-0.100827431588364,-0.247616782520891,
-0.0399999999999998));
#85213=CARTESIAN_POINT('Ctrl Pts',(-0.0907100227550067,-0.250413295320921,
-0.0400000000000001));
#85214=CARTESIAN_POINT('Ctrl Pts',(-0.0804585625301252,-0.252538295668516,
-0.0400000000000002));
#85215=CARTESIAN_POINT('Ctrl Pts',(-0.0655592239457918,-0.255626743458011,
-0.0400000000000004));
#85216=CARTESIAN_POINT('Ctrl Pts',(-0.0503757632529026,-0.257298270450147,
-0.0400000000000008));
#85217=CARTESIAN_POINT('Ctrl Pts',(-0.035087887712621,-0.257593498543919,
-0.0400000000000002));
#85218=CARTESIAN_POINT('Ctrl Pts',(-0.0266776628482832,-0.257755910557829,
-0.0399999999999999));
#85219=CARTESIAN_POINT('Ctrl Pts',(-0.0182246094922889,-0.257499357140891,
-0.0400000000000009));
#85220=CARTESIAN_POINT('Ctrl Pts',(-0.00982040497162541,-0.256833045226985,
-0.0400000000000007));
#85221=CARTESIAN_POINT('Ctrl Pts',(0.00491692967266122,-0.255664622727442,
-0.0400000000000002));
#85222=CARTESIAN_POINT('Ctrl Pts',(0.0195312833862859,-0.253242426124699,
-0.0400000000000002));
#85223=CARTESIAN_POINT('Ctrl Pts',(0.0338566095938309,-0.249610755855218,
-0.0400000000000004));
#85224=CARTESIAN_POINT('Ctrl Pts',(0.0444101672705453,-0.246935281587024,
-0.0400000000000006));
#85225=CARTESIAN_POINT('Ctrl Pts',(0.0548058406093567,-0.24360288402174,
-0.04));
#85226=CARTESIAN_POINT('Ctrl Pts',(0.0649723996581922,-0.23961836524148,
-0.04));
#85227=CARTESIAN_POINT('Ctrl Pts',(0.0711875157987854,-0.237182511884928,
-0.04));
#85228=CARTESIAN_POINT('Ctrl Pts',(0.0773193102033957,-0.234500720362044,
-0.0400000000000002));
#85229=CARTESIAN_POINT('Ctrl Pts',(0.0833170489198445,-0.231590456312328,
-0.0400000000000002));
#85230=CARTESIAN_POINT('Ctrl Pts',(0.0966561951856547,-0.225117943976167,
-0.0400000000000002));
#85231=CARTESIAN_POINT('Ctrl Pts',(0.109365981463997,-0.217507780687347,
-0.0399999999999999));
#85232=CARTESIAN_POINT('Ctrl Pts',(0.121261887594827,-0.208786977554813,
-0.0400000000000002));
#85233=CARTESIAN_POINT('Ctrl Pts',(0.130897115114624,-0.201723461634865,
-0.0400000000000004));
#85234=CARTESIAN_POINT('Ctrl Pts',(0.139998199893573,-0.193930449475644,
-0.0400000000000004));
#85235=CARTESIAN_POINT('Ctrl Pts',(0.148446367846058,-0.18540786851733,
-0.0400000000000005));
#85236=CARTESIAN_POINT('Ctrl Pts',(0.149136190345306,-0.184711969935559,
-0.0400000000000004));
#85237=CARTESIAN_POINT('Ctrl Pts',(0.149821647047686,-0.184011201202051,
-0.0400000000000001));
#85238=CARTESIAN_POINT('Ctrl Pts',(0.150502666328434,-0.183305559252938,
-0.04));
#85239=CARTESIAN_POINT('',(0.222488700208077,0.082706301833401,-0.0398895408386927));
#85240=CARTESIAN_POINT('Ctrl Pts',(0.223369910286723,0.0797362138773923,
-0.0399999999999998));
#85241=CARTESIAN_POINT('Ctrl Pts',(0.223023510600583,0.0807066044070377,
-0.0399631802795641));
#85242=CARTESIAN_POINT('Ctrl Pts',(0.222670787293575,0.0816747375972639,
-0.0399263605591283));
#85243=CARTESIAN_POINT('Ctrl Pts',(0.222311770321392,0.0826405312275324,
-0.0398895408386926));
#85244=CARTESIAN_POINT('Ctrl Pts',(0.222665717629832,0.0827839932162159,
-0.0400000000000001));
#85245=CARTESIAN_POINT('Ctrl Pts',(0.221253480978161,0.0887066597966071,
-0.0399999999999969));
#85246=CARTESIAN_POINT('Ctrl Pts',(0.219601459374371,0.0945593417108579,
-0.0399999999999963));
#85247=CARTESIAN_POINT('Ctrl Pts',(0.217708690025739,0.100327411027147,
-0.0399999999999962));
#85248=CARTESIAN_POINT('Ctrl Pts',(0.213879851975831,0.1119955011136,-0.0399999999999962));
#85249=CARTESIAN_POINT('Ctrl Pts',(0.209067649811371,0.123317664354657,
-0.0399999999999959));
#85250=CARTESIAN_POINT('Ctrl Pts',(0.203378325968185,0.134233488491038,
-0.0399999999999964));
#85251=CARTESIAN_POINT('Ctrl Pts',(0.199898449286141,0.140910155688135,
-0.0399999999999962));
#85252=CARTESIAN_POINT('Ctrl Pts',(0.196088082415695,0.147435983260384,
-0.0399999999999961));
#85253=CARTESIAN_POINT('Ctrl Pts',(0.191987668267784,0.153768999827833,
-0.0399999999999963));
#85254=CARTESIAN_POINT('Ctrl Pts',(0.185593130911648,0.163645248800932,
-0.0399999999999965));
#85255=CARTESIAN_POINT('Ctrl Pts',(0.178486227796011,0.173069463514982,
-0.0399999999999978));
#85256=CARTESIAN_POINT('Ctrl Pts',(0.170751201853388,0.181989599778708,
-0.0399999999999976));
#85257=CARTESIAN_POINT('Ctrl Pts',(0.16732716542848,0.18593824477469,-0.0399999999999976));
#85258=CARTESIAN_POINT('Ctrl Pts',(0.163779810148522,0.189788049195326,
-0.0399999999999972));
#85259=CARTESIAN_POINT('Ctrl Pts',(0.16011541559148,0.193534072345585,-0.0399999999999973));
#85260=CARTESIAN_POINT('Ctrl Pts',(0.156842239619411,0.196880162068013,
-0.0399999999999974));
#85261=CARTESIAN_POINT('Ctrl Pts',(0.153481935750538,0.200136982106501,
-0.0399999999999977));
#85262=CARTESIAN_POINT('Ctrl Pts',(0.150041516968305,0.203300204333427,
-0.0399999999999972));
#85263=CARTESIAN_POINT('Ctrl Pts',(0.1381660476245,0.214218860160297,-0.0399999999999957));
#85264=CARTESIAN_POINT('Ctrl Pts',(0.125334099709751,0.224030039279681,
-0.0399999999999991));
#85265=CARTESIAN_POINT('Ctrl Pts',(0.111739635875884,0.232604600158049,
-0.0399999999999995));
#85266=CARTESIAN_POINT('Ctrl Pts',(0.102821755693203,0.238229456530972,
-0.0399999999999998));
#85267=CARTESIAN_POINT('Ctrl Pts',(0.0935746853790765,0.243321776325075,
-0.0399999999999999));
#85268=CARTESIAN_POINT('Ctrl Pts',(0.0840435370389822,0.247837152868998,
-0.0399999999999999));
#85269=CARTESIAN_POINT('Ctrl Pts',(0.0785373322670779,0.250445714501441,
-0.0399999999999998));
#85270=CARTESIAN_POINT('Ctrl Pts',(0.0729353892307488,0.252861193764587,
-0.0400000000000001));
#85271=CARTESIAN_POINT('Ctrl Pts',(0.0672734922871532,0.255064885842267,
-0.0400000000000003));
#85272=CARTESIAN_POINT('Ctrl Pts',(0.0576677102794855,0.258803594957093,
-0.0400000000000006));
#85273=CARTESIAN_POINT('Ctrl Pts',(0.0478720024143959,0.261941980498935,
-0.0400000000000014));
#85274=CARTESIAN_POINT('Ctrl Pts',(0.0379326081771775,0.264446101529577,
-0.0400000000000018));
#85275=CARTESIAN_POINT('Ctrl Pts',(0.0266860283143166,0.267279553597704,
-0.0400000000000022));
#85276=CARTESIAN_POINT('Ctrl Pts',(0.015255426554341,0.269301474714493,
-0.0400000000000019));
#85277=CARTESIAN_POINT('Ctrl Pts',(0.00371085635712924,0.270547759765321,
-0.0400000000000023));
#85278=CARTESIAN_POINT('Ctrl Pts',(-0.00338729350177195,0.271314034984457,
-0.040000000000003));
#85279=CARTESIAN_POINT('Ctrl Pts',(-0.0105286670358888,0.271786812582468,
-0.0400000000000027));
#85280=CARTESIAN_POINT('Ctrl Pts',(-0.0176977769208803,0.271971820819257,
-0.0400000000000024));
#85281=CARTESIAN_POINT('Ctrl Pts',(-0.0232469593148744,0.272115024713018,
-0.0400000000000023));
#85282=CARTESIAN_POINT('Ctrl Pts',(-0.0288098460156715,0.272085302073594,
-0.040000000000003));
#85283=CARTESIAN_POINT('Ctrl Pts',(-0.0343596925541648,0.271886941169997,
-0.0400000000000031));
#85284=CARTESIAN_POINT('Ctrl Pts',(-0.0515871477842762,0.271271202777516,
-0.0400000000000034));
#85285=CARTESIAN_POINT('Ctrl Pts',(-0.0687382048994064,0.269036890911878,
-0.0400000000000034));
#85286=CARTESIAN_POINT('Ctrl Pts',(-0.0855957885720179,0.265293203132554,
-0.0400000000000028));
#85287=CARTESIAN_POINT('Ctrl Pts',(-0.094137880371246,0.263396197885558,
-0.0400000000000026));
#85288=CARTESIAN_POINT('Ctrl Pts',(-0.102604921020482,0.261110692191661,
-0.0400000000000023));
#85289=CARTESIAN_POINT('Ctrl Pts',(-0.110969298043269,0.258445247385233,
-0.0400000000000021));
#85290=CARTESIAN_POINT('Ctrl Pts',(-0.116744071982683,0.25660502172788,
-0.040000000000002));
#85291=CARTESIAN_POINT('Ctrl Pts',(-0.12247203470197,0.254582775191448,
-0.0400000000000022));
#85292=CARTESIAN_POINT('Ctrl Pts',(-0.128136696559136,0.252383171185569,
-0.0400000000000022));
#85293=CARTESIAN_POINT('Ctrl Pts',(-0.133443994806023,0.250322332466753,
-0.0400000000000022));
#85294=CARTESIAN_POINT('Ctrl Pts',(-0.138687644571475,0.248108961431596,
-0.0400000000000018));
#85295=CARTESIAN_POINT('Ctrl Pts',(-0.143855255028261,0.245748938027449,
-0.0400000000000017));
#85296=CARTESIAN_POINT('Ctrl Pts',(-0.159697617720826,0.238513805456196,
-0.0400000000000015));
#85297=CARTESIAN_POINT('Ctrl Pts',(-0.174844413355584,0.229896763780577,
-0.0400000000000008));
#85298=CARTESIAN_POINT('Ctrl Pts',(-0.189088023629515,0.219973317830906,
-0.0400000000000005));
#85299=CARTESIAN_POINT('Ctrl Pts',(-0.200581329367837,0.211965994119865,
-0.0400000000000002));
#85300=CARTESIAN_POINT('Ctrl Pts',(-0.211487041503738,0.203107005513314,
-0.0399999999999997));
#85301=CARTESIAN_POINT('Ctrl Pts',(-0.221686865784456,0.19341296114445,
-0.0399999999999998));
#85302=CARTESIAN_POINT('Ctrl Pts',(-0.103724760116696,0.212823727783082,
-1.59396608746666));
#85303=CARTESIAN_POINT('Ctrl Pts',(-0.174393327975359,0.178381702331853,
-1.58868131400033));
#85304=CARTESIAN_POINT('Ctrl Pts',(-0.277518531248041,0.0341781548206397,
-1.57811176706767));
#85305=CARTESIAN_POINT('Ctrl Pts',(-0.179349083795972,-0.214866166073336,
-1.56225744666869));
#85306=CARTESIAN_POINT('Ctrl Pts',(0.0827902547662305,-0.2670809958049,
-1.5464031262697));
#85307=CARTESIAN_POINT('Ctrl Pts',(0.269226441972677,-0.0758032933439426,
-1.53054880587072));
#85308=CARTESIAN_POINT('Ctrl Pts',(0.209939552040885,0.184851367163293,
-1.51469448547173));
#85309=CARTESIAN_POINT('Ctrl Pts',(-0.041041429718235,0.276658199552224,
-1.49884016507275));
#85310=CARTESIAN_POINT('Ctrl Pts',(-0.254537004881614,0.115941550403291,
-1.48298584467376));
#85311=CARTESIAN_POINT('Ctrl Pts',(-0.235665945800168,-0.150646965377197,
-1.46713152427478));
#85312=CARTESIAN_POINT('Ctrl Pts',(-0.00164253664402765,-0.279691657770853,
-1.45127720387579));
#85313=CARTESIAN_POINT('Ctrl Pts',(0.233877927031332,-0.15340291974329,
-1.43542288347681));
#85314=CARTESIAN_POINT('Ctrl Pts',(0.255884407477275,0.112936223822634,
-1.41956856307782));
#85315=CARTESIAN_POINT('Ctrl Pts',(0.0442844522027617,0.276170107760178,
-1.40371424267884));
#85316=CARTESIAN_POINT('Ctrl Pts',(-0.207743962043941,0.187279687461201,
-1.38785992227985));
#85317=CARTESIAN_POINT('Ctrl Pts',(-0.270115887608575,-0.0725853701266998,
-1.37200560188087));
#85318=CARTESIAN_POINT('Ctrl Pts',(-0.0858895457739192,-0.266184456976842,
-1.35615128148188));
#85319=CARTESIAN_POINT('Ctrl Pts',(0.176748293013421,-0.216774652656855,
-1.3402969610829));
#85320=CARTESIAN_POINT('Ctrl Pts',(0.278026506306114,0.030536329962957,
-1.32444264068391));
#85321=CARTESIAN_POINT('Ctrl Pts',(0.125484657012978,0.249969598727324,
-1.30858832028493));
#85322=CARTESIAN_POINT('Ctrl Pts',(-0.141616484291169,0.241196963701767,
-1.29273399988594));
#85323=CARTESIAN_POINT('Ctrl Pts',(-0.279431025008706,0.0122272374408218,
-1.27687967948696));
#85324=CARTESIAN_POINT('Ctrl Pts',(-0.162143281191983,-0.227905152839578,
-1.26102535908797));
#85325=CARTESIAN_POINT('Ctrl Pts',(0.103170691412443,-0.259975020756189,
-1.24517103868899));
#85326=CARTESIAN_POINT('Ctrl Pts',(0.274296559039192,-0.0547046662863507,
-1.22931671829));
#85327=CARTESIAN_POINT('Ctrl Pts',(0.195007576056607,0.200507476197715,
-1.21346239789102));
#85328=CARTESIAN_POINT('Ctrl Pts',(-0.0623105921992744,0.272669383914658,
-1.19760807749203));
#85329=CARTESIAN_POINT('Ctrl Pts',(-0.262743257945448,0.0959019457480826,
-1.18175375709305));
#85330=CARTESIAN_POINT('Ctrl Pts',(-0.22330848294228,-0.168417707595505,
-1.16589943669406));
#85331=CARTESIAN_POINT('Ctrl Pts',(0.0199923577595259,-0.278982989499441,
-1.15004511629507));
#85332=CARTESIAN_POINT('Ctrl Pts',(0.245041481085025,-0.134855016003514,
-1.13419079589609));
#85333=CARTESIAN_POINT('Ctrl Pts',(0.246383730268811,0.13238678276863,-1.1183364754971));
#85334=CARTESIAN_POINT('Ctrl Pts',(0.0227937194468614,0.278768092056046,
-1.10248215509812));
#85335=CARTESIAN_POINT('Ctrl Pts',(-0.22160546909146,0.170652333305773,
-1.08662783469914));
#85336=CARTESIAN_POINT('Ctrl Pts',(-0.263693332369467,-0.0932578643215929,
-1.07077351430015));
#85337=CARTESIAN_POINT('Ctrl Pts',(-0.0650463990182539,-0.272029720378002,
-1.05491919390117));
#85338=CARTESIAN_POINT('Ctrl Pts',(0.192983649933591,-0.202456201812523,
-1.03906487350218));
#85339=CARTESIAN_POINT('Ctrl Pts',(0.274832225875905,0.051946611190235,
-1.0232105531032));
#85340=CARTESIAN_POINT('Ctrl Pts',(0.10577692264544,0.25892555963007,-1.00735623270421));
#85341=CARTESIAN_POINT('Ctrl Pts',(-0.159845805071481,0.22952237667625,
-0.99150191230523));
#85342=CARTESIAN_POINT('Ctrl Pts',(-0.279539748657917,-0.00941975128844859,
-0.975647591906243));
#85343=CARTESIAN_POINT('Ctrl Pts',(-0.144032152112957,-0.239762261316874,
-0.959793271507259));
#85344=CARTESIAN_POINT('Ctrl Pts',(0.122967395841924,-0.251217480191813,
-0.943938951108274));
#85345=CARTESIAN_POINT('Ctrl Pts',(0.27770573960144,-0.0333275409606875,
-0.928084630709289));
#85346=CARTESIAN_POINT('Ctrl Pts',(0.178916873760631,0.214988267302641,
-0.912230310310303));
#85347=CARTESIAN_POINT('Ctrl Pts',(-0.0832114168254042,0.2670338235205,
-0.896375989911319));
#85348=CARTESIAN_POINT('Ctrl Pts',(-0.269373116497936,0.0752949327794278,
-0.880521669512333));
#85349=CARTESIAN_POINT('Ctrl Pts',(-0.209614747449241,-0.185183315786979,
-0.864667349113349));
#85350=CARTESIAN_POINT('Ctrl Pts',(0.0415082008413281,-0.276601287157137,
-0.848813028714363));
#85351=CARTESIAN_POINT('Ctrl Pts',(0.254736871721806,-0.115500341901908,
-0.832958708315379));
#85352=CARTESIAN_POINT('Ctrl Pts',(0.235407409800871,0.151044874805183,
-0.817104387916392));
#85353=CARTESIAN_POINT('Ctrl Pts',(0.00116635184411073,0.279695982126031,
-0.80125006751741));
#85354=CARTESIAN_POINT('Ctrl Pts',(-0.234139509198369,0.153002918359146,
-0.785395747118422));
#85355=CARTESIAN_POINT('Ctrl Pts',(-0.25569128467731,-0.113371820723387,
-0.769541426719439));
#85356=CARTESIAN_POINT('Ctrl Pts',(-0.0438136106375017,-0.276245489224665,
-0.753687106320452));
#85357=CARTESIAN_POINT('Ctrl Pts',(0.208063029442341,-0.186925061383818,
-0.737832785921468));
#85358=CARTESIAN_POINT('Ctrl Pts',(0.269991707513143,0.0730457436693384,
-0.721978465522483));
#85359=CARTESIAN_POINT('Ctrl Pts',(0.0854355836519637,0.266330553711205,
-0.706124145123497));
#85360=CARTESIAN_POINT('Ctrl Pts',(-0.177117650225534,0.216472956215444,
-0.690269824724514));
#85361=CARTESIAN_POINT('Ctrl Pts',(-0.277974032978924,-0.0310103173718541,
-0.674415504325526));
#85362=CARTESIAN_POINT('Ctrl Pts',(-0.125058271794479,-0.250183195778305,
-0.658561183926543));
#85363=CARTESIAN_POINT('Ctrl Pts',(0.142027526822356,-0.240955150222586,
-0.642706863527556));
#85364=CARTESIAN_POINT('Ctrl Pts',(0.279451466043086,-0.0117507838229697,
-0.626852543128573));
#85365=CARTESIAN_POINT('Ctrl Pts',(0.161754461395924,0.22818128103017,-0.610998222729586));
#85366=CARTESIAN_POINT('Ctrl Pts',(-0.103613805994735,0.259798733640734,
-0.595143902330603));
#85367=CARTESIAN_POINT('Ctrl Pts',(-0.274389433177387,0.0542369039931965,
-0.579289581931617));
#85368=CARTESIAN_POINT('Ctrl Pts',(-0.194665422011536,-0.200839678019582,
-0.563435261532631));
#85369=CARTESIAN_POINT('Ctrl Pts',(0.0627754102712604,-0.272562746279138,
-0.547580941133648));
#85370=CARTESIAN_POINT('Ctrl Pts',(0.262906391415409,-0.0954538220697194,
-0.531726620734661));
#85371=CARTESIAN_POINT('Ctrl Pts',(0.223021001639017,0.168798209768152,
-0.515872300335677));
#85372=CARTESIAN_POINT('Ctrl Pts',(-0.0204680021875169,0.278948496465033,
-0.500017979936691));
#85373=CARTESIAN_POINT('Ctrl Pts',(-0.245271056334415,0.134437017682742,
-0.484163659537707));
#85374=CARTESIAN_POINT('Ctrl Pts',(-0.246157649098411,-0.132806681217667,
-0.468309339138721));
#85375=CARTESIAN_POINT('Ctrl Pts',(-0.0223183792644695,-0.278806550749913,
-0.452455018739736));
#85376=CARTESIAN_POINT('Ctrl Pts',(0.221896113850858,-0.1702742419819,-0.436600698340751));
#85377=CARTESIAN_POINT('Ctrl Pts',(0.263533941788505,0.0937073329898119,
-0.420746377941766));
#85378=CARTESIAN_POINT('Ctrl Pts',(0.0645824867269263,0.272140230804651,
-0.404892057542781));
#85379=CARTESIAN_POINT('Ctrl Pts',(-0.193328563134106,0.202126865260915,
-0.389037737143796));
#85380=CARTESIAN_POINT('Ctrl Pts',(-0.274743255159592,-0.0524151320788667,
-0.373183416744811));
#85381=CARTESIAN_POINT('Ctrl Pts',(-0.105335295510445,-0.259105535627046,
-0.357329096345826));
#85382=CARTESIAN_POINT('Ctrl Pts',(0.160236917697637,-0.229249501915933,
-0.341474775946841));
#85383=CARTESIAN_POINT('Ctrl Pts',(0.279523275373005,0.00989636086202485,
-0.325620455547856));
#85384=CARTESIAN_POINT('Ctrl Pts',(0.143623153177434,0.240007490565944,
-0.30976613514887));
#85385=CARTESIAN_POINT('Ctrl Pts',(-0.123395571661222,0.251007454096603,
-0.293911814749885));
#85386=CARTESIAN_POINT('Ctrl Pts',(-0.277762118238676,0.032853993377835,
-0.2780574943509));
#85387=CARTESIAN_POINT('Ctrl Pts',(-0.178550133277567,-0.215293006392593,
-0.262203173951915));
#85388=CARTESIAN_POINT('Ctrl Pts',(0.0836667492467019,-0.266891570065015,
-0.24634885355293));
#85389=CARTESIAN_POINT('Ctrl Pts',(0.269500811469429,-0.074835511252918,
-0.230494533153945));
#85390=CARTESIAN_POINT('Ctrl Pts',(0.209299260770646,0.185540400134779,
-0.21464021275496));
#85391=CARTESIAN_POINT('Ctrl Pts',(-0.0419808241655782,0.276530198966801,
-0.198785892355975));
#85392=CARTESIAN_POINT('Ctrl Pts',(-0.254931386165377,0.11506567559891,
-0.18293157195699));
#85393=CARTESIAN_POINT('Ctrl Pts',(-0.235153442315408,-0.151445715536821,
-0.167077251558005));
#85394=CARTESIAN_POINT('Ctrl Pts',(-0.000681989459094153,-0.279698167413373,
-0.151222931159019));
#85395=CARTESIAN_POINT('Ctrl Pts',(0.234385766356705,-0.152602329150558,
-0.135368610760035));
#85396=CARTESIAN_POINT('Ctrl Pts',(0.255524894043667,0.113805412776539,
-0.119514290361049));
#85397=CARTESIAN_POINT('Ctrl Pts',(0.0432903726894156,0.276324012658087,
-0.103659969962065));
#85398=CARTESIAN_POINT('Ctrl Pts',(-0.208281425456119,0.186561872885006,
-0.0878056495630792));
#85399=CARTESIAN_POINT('Ctrl Pts',(-0.270060833707632,-0.0734895181549532,
-0.0719513291640941));
#85400=CARTESIAN_POINT('Ctrl Pts',(-0.0845542121726118,-0.266546212100623,
-0.0560944337615691));
#85401=CARTESIAN_POINT('Ctrl Pts',(0.0895616202659112,-0.232850436616742,
-0.0455223118253725));
#85402=CARTESIAN_POINT('Ctrl Pts',(0.150324724191651,-0.182907739666978,
-0.0402349633555041));
#85403=CARTESIAN_POINT('Ctrl Pts',(-0.112169338338267,0.230150416363986,
-1.58283766981155));
#85404=CARTESIAN_POINT('Ctrl Pts',(-0.188591269698735,0.192904350896613,
-1.57755289634522));
#85405=CARTESIAN_POINT('Ctrl Pts',(-0.300112239273236,0.0369607122498147,
-1.56698334941257));
#85406=CARTESIAN_POINT('Ctrl Pts',(-0.193950490108011,-0.232359136358677,
-1.55112902901358));
#85407=CARTESIAN_POINT('Ctrl Pts',(0.0895304851757355,-0.288824949302914,
-1.5352747086146));
#85408=CARTESIAN_POINT('Ctrl Pts',(0.291145063389551,-0.0819746919509459,
-1.51942038821561));
#85409=CARTESIAN_POINT('Ctrl Pts',(0.227031430267615,0.199900732692013,
-1.50356606781663));
#85410=CARTESIAN_POINT('Ctrl Pts',(-0.0443827492179445,0.299181865108354,
-1.48771174741764));
#85411=CARTESIAN_POINT('Ctrl Pts',(-0.275259710295338,0.125380738215436,
-1.47185742701866));
#85412=CARTESIAN_POINT('Ctrl Pts',(-0.254852295435795,-0.162911636623858,
-1.45600310661967));
#85413=CARTESIAN_POINT('Ctrl Pts',(-0.00177626102340334,-0.302462287264814,
-1.44014878622069));
#85414=CARTESIAN_POINT('Ctrl Pts',(0.252918708103212,-0.165891962414805,
-1.4242944658217));
#85415=CARTESIAN_POINT('Ctrl Pts',(0.276716809424425,0.122130737987296,
-1.40844014542272));
#85416=CARTESIAN_POINT('Ctrl Pts',(0.0478897969652389,0.298654036137713,
-1.39258582502373));
#85417=CARTESIAN_POINT('Ctrl Pts',(-0.224657089975649,0.202526750633954,
-1.37673150462475));
#85418=CARTESIAN_POINT('Ctrl Pts',(-0.292106921757353,-0.078494786885889,
-1.36087718422576));
#85419=CARTESIAN_POINT('Ctrl Pts',(-0.0928820997879023,-0.28785542026255,
-1.34502286382677));
#85420=CARTESIAN_POINT('Ctrl Pts',(0.191137960284783,-0.234422999192009,
-1.32916854342779));
#85421=CARTESIAN_POINT('Ctrl Pts',(0.30066157027282,0.0330223942997807,
-1.3133142230288));
#85422=CARTESIAN_POINT('Ctrl Pts',(0.135700780921689,0.270320456392293,
-1.29745990262982));
#85423=CARTESIAN_POINT('Ctrl Pts',(-0.153145953992668,0.260833611928227,
-1.28160558223083));
#85424=CARTESIAN_POINT('Ctrl Pts',(-0.30218043552135,0.0132226975690194,
-1.26575126183185));
#85425=CARTESIAN_POINT('Ctrl Pts',(-0.175343905802614,-0.246459670469582,
-1.24989694143286));
#85426=CARTESIAN_POINT('Ctrl Pts',(0.111570161055234,-0.281140453155943,
-1.23404262103388));
#85427=CARTESIAN_POINT('Ctrl Pts',(0.296627955574683,-0.059158355386433,
-1.21818830063489));
#85428=CARTESIAN_POINT('Ctrl Pts',(0.21088379238101,0.216831457712414,-1.20233398023591));
#85429=CARTESIAN_POINT('Ctrl Pts',(-0.0673835050627706,0.294868306703247,
-1.18647965983692));
#85430=CARTESIAN_POINT('Ctrl Pts',(-0.284134061755598,0.10370964259462,
-1.17062533943794));
#85431=CARTESIAN_POINT('Ctrl Pts',(-0.241488770364737,-0.182129154159352,
-1.15477101903895));
#85432=CARTESIAN_POINT('Ctrl Pts',(0.0216200021979781,-0.301695923948899,
-1.13891669863997));
#85433=CARTESIAN_POINT('Ctrl Pts',(0.264991124277493,-0.145834012049705,
-1.12306237824098));
#85434=CARTESIAN_POINT('Ctrl Pts',(0.266442650438278,0.143164831725639,
-1.107208057842));
#85435=CARTESIAN_POINT('Ctrl Pts',(0.0246494320714388,0.301463530988827,
-1.09135373744301));
#85436=CARTESIAN_POINT('Ctrl Pts',(-0.23964710848369,0.18454570819209,-1.07549941704403));
#85437=CARTESIAN_POINT('Ctrl Pts',(-0.285161484903114,-0.100850297691931,
-1.05964509664504));
#85438=CARTESIAN_POINT('Ctrl Pts',(-0.0703420430276832,-0.294176566027392,
-1.04379077624606));
#85439=CARTESIAN_POINT('Ctrl Pts',(0.208695091690748,-0.218938835570607,
-1.02793645584707));
#85440=CARTESIAN_POINT('Ctrl Pts',(0.297207232832846,0.0561757578380344,
-1.01208213544809));
#85441=CARTESIAN_POINT('Ctrl Pts',(0.1143885742541,0.280005551903859,-0.996227815049101));
#85442=CARTESIAN_POINT('Ctrl Pts',(-0.172859384498394,0.248208557885668,
-0.980373494650116));
#85443=CARTESIAN_POINT('Ctrl Pts',(-0.302298010724994,-0.0101866446174213,
-0.964519174251132));
#85444=CARTESIAN_POINT('Ctrl Pts',(-0.155758289378265,-0.259282105643277,
-0.948664853852145));
#85445=CARTESIAN_POINT('Ctrl Pts',(0.132978581133861,-0.27166993204342,
-0.932810533453161));
#85446=CARTESIAN_POINT('Ctrl Pts',(0.300314688882263,-0.0360408470821843,
-0.916956213054176));
#85447=CARTESIAN_POINT('Ctrl Pts',(0.193483092414029,0.232491178255772,
-0.901101892655191));
#85448=CARTESIAN_POINT('Ctrl Pts',(-0.0899859354410101,0.288773936565713,
-0.885247572256206));
#85449=CARTESIAN_POINT('Ctrl Pts',(-0.291303679176474,0.081424944059558,
-0.86939325185722));
#85450=CARTESIAN_POINT('Ctrl Pts',(-0.226680182252261,-0.200259706358852,
-0.853538931458236));
#85451=CARTESIAN_POINT('Ctrl Pts',(0.0448875217329529,-0.299120319285611,
-0.837684611059252));
#85452=CARTESIAN_POINT('Ctrl Pts',(0.275475848960733,-0.124903609460319,
-0.821830290660265));
#85453=CARTESIAN_POINT('Ctrl Pts',(0.25457271115963,0.163341941183787,-0.80597597026128));
#85454=CARTESIAN_POINT('Ctrl Pts',(0.00126130843278474,0.30246696368015,
-0.790121649862295));
#85455=CARTESIAN_POINT('Ctrl Pts',(-0.253201586545781,0.165459395585599,
-0.77426732946331));
#85456=CARTESIAN_POINT('Ctrl Pts',(-0.276507963854035,-0.122601798282684,
-0.758413009064326));
#85457=CARTESIAN_POINT('Ctrl Pts',(-0.0473806226198084,-0.298735554658316,
-0.74255868866534));
#85458=CARTESIAN_POINT('Ctrl Pts',(0.225002133713745,-0.202143253266375,
-0.726704368266355));
#85459=CARTESIAN_POINT('Ctrl Pts',(0.291972631746717,0.0789926409721084,
-0.71085004786737));
#85460=CARTESIAN_POINT('Ctrl Pts',(0.0923911790974798,0.288013411218696,
-0.694995727468384));
#85461=CARTESIAN_POINT('Ctrl Pts',(-0.191537388097839,0.234096740638372,
-0.679141407069401));
#85462=CARTESIAN_POINT('Ctrl Pts',(-0.300604824917278,-0.0335349706024578,
-0.663287086670414));
#85463=CARTESIAN_POINT('Ctrl Pts',(-0.135239682262291,-0.270551443090672,
-0.647432766271431));
#85464=CARTESIAN_POINT('Ctrl Pts',(0.153590460865475,-0.260572111608241,
-0.631578445872444));
#85465=CARTESIAN_POINT('Ctrl Pts',(0.302202540728427,-0.012707454275101,
-0.615724125473459));
#85466=CARTESIAN_POINT('Ctrl Pts',(0.174923430891825,0.246758279175934,
-0.599869805074475));
#85467=CARTESIAN_POINT('Ctrl Pts',(-0.112049351071656,0.280949813919219,
-0.584015484675488));
#85468=CARTESIAN_POINT('Ctrl Pts',(-0.296728390905827,0.0586525110069064,
-0.568161164276505));
#85469=CARTESIAN_POINT('Ctrl Pts',(-0.210513782435438,-0.217190705191142,
-0.552306843877518));
#85470=CARTESIAN_POINT('Ctrl Pts',(0.0678861655222763,-0.294752987342616,
-0.536452523478534));
#85471=CARTESIAN_POINT('Ctrl Pts',(0.284310476464735,-0.10322503567493,
-0.52059820307955));
#85472=CARTESIAN_POINT('Ctrl Pts',(0.241177884250994,0.182540634281302,
-0.504743882680563));
#85473=CARTESIAN_POINT('Ctrl Pts',(-0.0221343704231927,0.301658622721666,
-0.488889562281578));
#85474=CARTESIAN_POINT('Ctrl Pts',(-0.265239390012636,0.145381983093314,
-0.473035241882593));
#85475=CARTESIAN_POINT('Ctrl Pts',(-0.266198163246733,-0.143618915506068,
-0.457180921483609));
#85476=CARTESIAN_POINT('Ctrl Pts',(-0.0241353928614716,-0.301505120733064,
-0.441326601084624));
#85477=CARTESIAN_POINT('Ctrl Pts',(0.23996141560107,-0.184136835194144,
-0.425472280685638));
#85478=CARTESIAN_POINT('Ctrl Pts',(0.284989117804036,0.10133635910158,-0.409617960286653));
#85479=CARTESIAN_POINT('Ctrl Pts',(0.0698403620914573,0.294296073475977,
-0.393763639887668));
#85480=CARTESIAN_POINT('Ctrl Pts',(-0.209068085423801,0.218582686633334,
-0.377909319488683));
#85481=CARTESIAN_POINT('Ctrl Pts',(-0.297111018714161,-0.0566824225728229,
-0.362054999089698));
#85482=CARTESIAN_POINT('Ctrl Pts',(-0.113910992783014,-0.280200180346236,
-0.346200678690714));
#85483=CARTESIAN_POINT('Ctrl Pts',(0.173282338906218,-0.247913467482185,
-0.330346358291728));
#85484=CARTESIAN_POINT('Ctrl Pts',(0.302280196295086,0.010702056563939,
-0.314492037892742));
#85485=CARTESIAN_POINT('Ctrl Pts',(0.155315992477052,0.259547299822357,
-0.298637717493759));
#85486=CARTESIAN_POINT('Ctrl Pts',(-0.133441616172835,0.271442807024216,
-0.282783397094773));
#85487=CARTESIAN_POINT('Ctrl Pts',(-0.30037565749215,0.0355287464132556,
-0.266929076695788));
#85488=CARTESIAN_POINT('Ctrl Pts',(-0.193086494366649,-0.232820727170103,
-0.251074756296802));
#85489=CARTESIAN_POINT('Ctrl Pts',(0.0904783379914081,-0.288620101782581,
-0.235220435897817));
#85490=CARTESIAN_POINT('Ctrl Pts',(0.291441770220941,-0.0809281194962718,
-0.219366115498832));
#85491=CARTESIAN_POINT('Ctrl Pts',(0.226339010752297,0.200645862132831,
-0.203511795099848));
#85492=CARTESIAN_POINT('Ctrl Pts',(-0.0453986228963076,0.29904344356891,
-0.187657474700862));
#85493=CARTESIAN_POINT('Ctrl Pts',(-0.275686199473072,0.124433555525748,
-0.171803154301878));
#85494=CARTESIAN_POINT('Ctrl Pts',(-0.254298067335225,-0.163775415694561,
-0.155948833902892));
#85495=CARTESIAN_POINT('Ctrl Pts',(-0.000737512492624156,-0.302469326879015,
-0.140094513503908));
#85496=CARTESIAN_POINT('Ctrl Pts',(0.253467892319643,-0.165026193075203,
-0.124240193104921));
#85497=CARTESIAN_POINT('Ctrl Pts',(0.27632802680467,0.12307069050915,-0.108385872705936));
#85498=CARTESIAN_POINT('Ctrl Pts',(0.0468147861274968,0.298820470946009,
-0.0925315523069517));
#85499=CARTESIAN_POINT('Ctrl Pts',(-0.225238310074468,0.201750496382117,
-0.0766772319079666));
#85500=CARTESIAN_POINT('Ctrl Pts',(-0.292047385734954,-0.0794725446167814,
-0.0608229115089816));
#85501=CARTESIAN_POINT('Ctrl Pts',(-0.0914380522302025,-0.28824662707594,
-0.0449660161064564));
#85502=CARTESIAN_POINT('Ctrl Pts',(0.0968531300957259,-0.251807566271467,
-0.0343938941702599));
#85503=CARTESIAN_POINT('Ctrl Pts',(0.162563160710032,-0.197798868007127,
-0.0291065457003915));
#85504=CARTESIAN_POINT('Ctrl Pts',(-0.120613916559838,0.24747710494489,
-1.57170925215644));
#85505=CARTESIAN_POINT('Ctrl Pts',(-0.202789211422113,0.207426999461372,
-1.56642447869011));
#85506=CARTESIAN_POINT('Ctrl Pts',(-0.32270594729843,0.0397432696789904,
-1.55585493175745));
#85507=CARTESIAN_POINT('Ctrl Pts',(-0.20855189642005,-0.249852106644019,
-1.54000061135847));
#85508=CARTESIAN_POINT('Ctrl Pts',(0.0962707155852401,-0.310568902800926,
-1.52414629095948));
#85509=CARTESIAN_POINT('Ctrl Pts',(0.313063684806424,-0.0881460905579498,
-1.5082919705605));
#85510=CARTESIAN_POINT('Ctrl Pts',(0.244123308494345,0.214950098220732,
-1.49243765016151));
#85511=CARTESIAN_POINT('Ctrl Pts',(-0.0477240687176538,0.321705530664484,
-1.47658332976253));
#85512=CARTESIAN_POINT('Ctrl Pts',(-0.295982415709062,0.134819926027581,
-1.46072900936354));
#85513=CARTESIAN_POINT('Ctrl Pts',(-0.274038645071423,-0.175176307870519,
-1.44487468896456));
#85514=CARTESIAN_POINT('Ctrl Pts',(-0.00190998540277913,-0.325232916758775,
-1.42902036856557));
#85515=CARTESIAN_POINT('Ctrl Pts',(0.271959489175091,-0.178381005086319,
-1.41316604816659));
#85516=CARTESIAN_POINT('Ctrl Pts',(0.297549211371575,0.131325252151957,
-1.3973117277676));
#85517=CARTESIAN_POINT('Ctrl Pts',(0.0514951417277158,0.32113796451525,
-1.38145740736861));
#85518=CARTESIAN_POINT('Ctrl Pts',(-0.241570217907355,0.217773813806707,
-1.36560308696963));
#85519=CARTESIAN_POINT('Ctrl Pts',(-0.314097955906133,-0.0844042036450784,
-1.34974876657064));
#85520=CARTESIAN_POINT('Ctrl Pts',(-0.099874653801885,-0.309526383548257,
-1.33389444617166));
#85521=CARTESIAN_POINT('Ctrl Pts',(0.205527627556145,-0.252071345727164,
-1.31804012577267));
#85522=CARTESIAN_POINT('Ctrl Pts',(0.323296634239525,0.0355084586366044,
-1.30218580537369));
#85523=CARTESIAN_POINT('Ctrl Pts',(0.1459169048304,0.290671314057262,-1.2863314849747));
#85524=CARTESIAN_POINT('Ctrl Pts',(-0.164675423694167,0.280470260154686,
-1.27047716457572));
#85525=CARTESIAN_POINT('Ctrl Pts',(-0.324929846033993,0.0142181576972166,
-1.25462284417674));
#85526=CARTESIAN_POINT('Ctrl Pts',(-0.188544530413246,-0.265014188099586,
-1.23876852377775));
#85527=CARTESIAN_POINT('Ctrl Pts',(0.119969630698024,-0.302305885555697,
-1.22291420337877));
#85528=CARTESIAN_POINT('Ctrl Pts',(0.318959352110174,-0.0636120444865149,
-1.20705988297978));
#85529=CARTESIAN_POINT('Ctrl Pts',(0.226760008705413,0.233155439227114,
-1.19120556258079));
#85530=CARTESIAN_POINT('Ctrl Pts',(-0.0724564179262672,0.317067229491835,
-1.17535124218181));
#85531=CARTESIAN_POINT('Ctrl Pts',(-0.305524865565747,0.111517339441156,
-1.15949692178283));
#85532=CARTESIAN_POINT('Ctrl Pts',(-0.259669057787194,-0.1958406007232,
-1.14364260138384));
#85533=CARTESIAN_POINT('Ctrl Pts',(0.0232476466364306,-0.324408858398355,
-1.12778828098485));
#85534=CARTESIAN_POINT('Ctrl Pts',(0.28494076746996,-0.156813008095897,
-1.11193396058587));
#85535=CARTESIAN_POINT('Ctrl Pts',(0.286501570607746,0.15394288068265,-1.09607964018688));
#85536=CARTESIAN_POINT('Ctrl Pts',(0.0265051446960164,0.324158969921607,
-1.0802253197879));
#85537=CARTESIAN_POINT('Ctrl Pts',(-0.25768874787592,0.198439083078409,
-1.06437099938891));
#85538=CARTESIAN_POINT('Ctrl Pts',(-0.306629637436761,-0.108442731062269,
-1.04851667898993));
#85539=CARTESIAN_POINT('Ctrl Pts',(-0.0756376870371126,-0.316323411676782,
-1.03266235859094));
#85540=CARTESIAN_POINT('Ctrl Pts',(0.224406533447907,-0.235421469328689,
-1.01680803819196));
#85541=CARTESIAN_POINT('Ctrl Pts',(0.319582239789786,0.0604049044858338,
-1.00095371779297));
#85542=CARTESIAN_POINT('Ctrl Pts',(0.123000225862759,0.301085544177648,
-0.985099397393988));
#85543=CARTESIAN_POINT('Ctrl Pts',(-0.185872963925308,0.266894739095086,
-0.969245076995004));
#85544=CARTESIAN_POINT('Ctrl Pts',(-0.325056272792072,-0.0109535379463947,
-0.953390756596019));
#85545=CARTESIAN_POINT('Ctrl Pts',(-0.167484426643573,-0.27880194996968,
-0.937536436197032));
#85546=CARTESIAN_POINT('Ctrl Pts',(0.142989766425799,-0.292122383895027,
-0.92168211579805));
#85547=CARTESIAN_POINT('Ctrl Pts',(0.322923638163087,-0.038754153203681,
-0.905827795399063));
#85548=CARTESIAN_POINT('Ctrl Pts',(0.208049311067426,0.249994089208903,
-0.889973475000078));
#85549=CARTESIAN_POINT('Ctrl Pts',(-0.0967604540566158,0.310514049610926,
-0.874119154601094));
#85550=CARTESIAN_POINT('Ctrl Pts',(-0.313234241855012,0.0875549553396883,
-0.858264834202108));
#85551=CARTESIAN_POINT('Ctrl Pts',(-0.243745617055283,-0.215336096930725,
-0.842410513803123));
#85552=CARTESIAN_POINT('Ctrl Pts',(0.0482668426245778,-0.321639351414085,
-0.826556193404139));
#85553=CARTESIAN_POINT('Ctrl Pts',(0.296214826199661,-0.134306877018729,
-0.810701873005152));
#85554=CARTESIAN_POINT('Ctrl Pts',(0.273738012518388,0.175639007562391,
-0.794847552606168));
#85555=CARTESIAN_POINT('Ctrl Pts',(0.00135626502145843,0.325237945234271,
-0.778993232207183));
#85556=CARTESIAN_POINT('Ctrl Pts',(-0.272263663893192,0.177915872812052,
-0.763138911808198));
#85557=CARTESIAN_POINT('Ctrl Pts',(-0.29732464303076,-0.131831775841982,
-0.747284591409212));
#85558=CARTESIAN_POINT('Ctrl Pts',(-0.0509476346021148,-0.321225620091967,
-0.731430271010228));
#85559=CARTESIAN_POINT('Ctrl Pts',(0.241941237985149,-0.217361445148932,
-0.715575950611242));
#85560=CARTESIAN_POINT('Ctrl Pts',(0.313953555980292,0.0849395382748782,
-0.699721630212258));
#85561=CARTESIAN_POINT('Ctrl Pts',(0.0993467745429957,0.309696268726186,
-0.683867309813271));
#85562=CARTESIAN_POINT('Ctrl Pts',(-0.205957125970144,0.251720525061298,
-0.668012989414289));
#85563=CARTESIAN_POINT('Ctrl Pts',(-0.323235616855631,-0.036059623833061,
-0.652158669015301));
#85564=CARTESIAN_POINT('Ctrl Pts',(-0.145421092730103,-0.290919690403039,
-0.636304348616318));
#85565=CARTESIAN_POINT('Ctrl Pts',(0.165153394908594,-0.280189072993896,
-0.620450028217332));
#85566=CARTESIAN_POINT('Ctrl Pts',(0.324953615413767,-0.0136641247272328,
-0.604595707818346));
#85567=CARTESIAN_POINT('Ctrl Pts',(0.188092400387725,0.265335277321699,
-0.588741387419363));
#85568=CARTESIAN_POINT('Ctrl Pts',(-0.120484896148577,0.302100894197703,
-0.572887067020376));
#85569=CARTESIAN_POINT('Ctrl Pts',(-0.319067348634266,0.0630681180206169,
-0.557032746621392));
#85570=CARTESIAN_POINT('Ctrl Pts',(-0.226362142859338,-0.233541732362702,
-0.541178426222406));
#85571=CARTESIAN_POINT('Ctrl Pts',(0.0729969207732917,-0.316943228406093,
-0.525324105823422));
#85572=CARTESIAN_POINT('Ctrl Pts',(0.305714561514062,-0.11099624928014,
-0.509469785424436));
#85573=CARTESIAN_POINT('Ctrl Pts',(0.25933476686297,0.196283058794453,-0.493615465025452));
#85574=CARTESIAN_POINT('Ctrl Pts',(-0.0238007386588687,0.324368748978298,
-0.477761144626466));
#85575=CARTESIAN_POINT('Ctrl Pts',(-0.285207723690857,0.156326948503885,
-0.461906824227481));
#85576=CARTESIAN_POINT('Ctrl Pts',(-0.286238677395056,-0.154431149794468,
-0.446052503828496));
#85577=CARTESIAN_POINT('Ctrl Pts',(-0.0259524064584728,-0.324203690716216,
-0.430198183429511));
#85578=CARTESIAN_POINT('Ctrl Pts',(0.258026717351281,-0.197999428406388,
-0.414343863030526));
#85579=CARTESIAN_POINT('Ctrl Pts',(0.306444293819567,0.108965385213349,
-0.39848954263154));
#85580=CARTESIAN_POINT('Ctrl Pts',(0.0750982374559877,0.316451916147304,
-0.382635222232556));
#85581=CARTESIAN_POINT('Ctrl Pts',(-0.224807607713496,0.235038508005751,
-0.36678090183357));
#85582=CARTESIAN_POINT('Ctrl Pts',(-0.319478782268731,-0.0609497130667787,
-0.350926581434586));
#85583=CARTESIAN_POINT('Ctrl Pts',(-0.122486690055583,-0.301294825065426,
-0.3350722610356));
#85584=CARTESIAN_POINT('Ctrl Pts',(0.186327760114798,-0.266577433048437,
-0.319217940636616));
#85585=CARTESIAN_POINT('Ctrl Pts',(0.325037117217167,0.0115077522658523,
-0.30336362023763));
#85586=CARTESIAN_POINT('Ctrl Pts',(0.16700883177667,0.279087109078769,-0.287509299838645));
#85587=CARTESIAN_POINT('Ctrl Pts',(-0.143487660684447,0.291878159951829,
-0.27165497943966));
#85588=CARTESIAN_POINT('Ctrl Pts',(-0.322989196745625,0.0382034994486758,
-0.255800659040675));
#85589=CARTESIAN_POINT('Ctrl Pts',(-0.207622855455732,-0.250348447947614,
-0.23994633864169));
#85590=CARTESIAN_POINT('Ctrl Pts',(0.0972899267361147,-0.310348633500145,
-0.224092018242705));
#85591=CARTESIAN_POINT('Ctrl Pts',(0.313382728972451,-0.0870207277396255,
-0.20823769784372));
#85592=CARTESIAN_POINT('Ctrl Pts',(0.243378760733948,0.215751324130884,
-0.192383377444734));
#85593=CARTESIAN_POINT('Ctrl Pts',(-0.0488164216270374,0.321556688171018,
-0.17652905704575));
#85594=CARTESIAN_POINT('Ctrl Pts',(-0.296441012780766,0.133801435452586,
-0.160674736646764));
#85595=CARTESIAN_POINT('Ctrl Pts',(-0.273442692355043,-0.176105115852303,
-0.14482041624778));
#85596=CARTESIAN_POINT('Ctrl Pts',(-0.000793035526154019,-0.325240486344656,
-0.128966095848794));
#85597=CARTESIAN_POINT('Ctrl Pts',(0.272550018282581,-0.177450056999848,
-0.11311177544981));
#85598=CARTESIAN_POINT('Ctrl Pts',(0.297131159565674,0.132335968241762,
-0.0972574550508239));
#85599=CARTESIAN_POINT('Ctrl Pts',(0.0503391995655778,0.321316929233932,
-0.0814031346518392));
#85600=CARTESIAN_POINT('Ctrl Pts',(-0.242195194692815,0.216939119879229,
-0.0655488142528539));
#85601=CARTESIAN_POINT('Ctrl Pts',(-0.314033937762277,-0.0854555710786095,
-0.049694493853869));
#85602=CARTESIAN_POINT('Ctrl Pts',(-0.0983218922877928,-0.309947042051257,
-0.0338375984513437));
#85603=CARTESIAN_POINT('Ctrl Pts',(0.104144639925541,-0.270764695926192,
-0.0232654765151473));
#85604=CARTESIAN_POINT('Ctrl Pts',(0.174801597228414,-0.212689996347276,
-0.017978128045279));
#85605=CARTESIAN_POINT('Ctrl Pts',(-0.129058494781408,0.264803793525795,
-1.56058083450132));
#85606=CARTESIAN_POINT('Ctrl Pts',(-0.216987153145491,0.221949648026132,
-1.55529606103499));
#85607=CARTESIAN_POINT('Ctrl Pts',(-0.345299655323625,0.0425258271081653,
-1.54472651410234));
#85608=CARTESIAN_POINT('Ctrl Pts',(-0.223153302732089,-0.267345076929359,
-1.52887219370335));
#85609=CARTESIAN_POINT('Ctrl Pts',(0.103010945994745,-0.33231285629894,
-1.51301787330437));
#85610=CARTESIAN_POINT('Ctrl Pts',(0.334982306223297,-0.0943174891649531,
-1.49716355290538));
#85611=CARTESIAN_POINT('Ctrl Pts',(0.261215186721073,0.229999463749451,
-1.48130923250639));
#85612=CARTESIAN_POINT('Ctrl Pts',(-0.0510653882173629,0.344229196220614,
-1.46545491210741));
#85613=CARTESIAN_POINT('Ctrl Pts',(-0.316705121122787,0.144259113839725,
-1.44960059170842));
#85614=CARTESIAN_POINT('Ctrl Pts',(-0.29322499470705,-0.18744097911718,
-1.43374627130944));
#85615=CARTESIAN_POINT('Ctrl Pts',(-0.00204370978215536,-0.348003546252736,
-1.41789195091045));
#85616=CARTESIAN_POINT('Ctrl Pts',(0.29100027024697,-0.190870047757833,
-1.40203763051147));
#85617=CARTESIAN_POINT('Ctrl Pts',(0.318381613318725,0.140519766316618,
-1.38618331011248));
#85618=CARTESIAN_POINT('Ctrl Pts',(0.0551004864901935,0.343621892892786,
-1.3703289897135));
#85619=CARTESIAN_POINT('Ctrl Pts',(-0.258483345839064,0.233020876979461,
-1.35447466931451));
#85620=CARTESIAN_POINT('Ctrl Pts',(-0.336088990054911,-0.0903136204042676,
-1.33862034891553));
#85621=CARTESIAN_POINT('Ctrl Pts',(-0.106867207815869,-0.331197346833964,
-1.32276602851654));
#85622=CARTESIAN_POINT('Ctrl Pts',(0.219917294827507,-0.269719692262318,
-1.30691170811756));
#85623=CARTESIAN_POINT('Ctrl Pts',(0.345931698206229,0.0379945229734283,
-1.29105738771857));
#85624=CARTESIAN_POINT('Ctrl Pts',(0.156133028739111,0.31102217172223,-1.27520306731959));
#85625=CARTESIAN_POINT('Ctrl Pts',(-0.176204893395666,0.300106908381147,
-1.2593487469206));
#85626=CARTESIAN_POINT('Ctrl Pts',(-0.347679256546638,0.0152136178254138,
-1.24349442652162));
#85627=CARTESIAN_POINT('Ctrl Pts',(-0.201745155023878,-0.283568705729589,
-1.22764010612263));
#85628=CARTESIAN_POINT('Ctrl Pts',(0.128369100340815,-0.323471317955452,
-1.21178578572365));
#85629=CARTESIAN_POINT('Ctrl Pts',(0.341290748645665,-0.0680657335865966,
-1.19593146532466));
#85630=CARTESIAN_POINT('Ctrl Pts',(0.242636225029816,0.249479420741813,
-1.18007714492568));
#85631=CARTESIAN_POINT('Ctrl Pts',(-0.0775293307897633,0.339266152280424,
-1.16422282452669));
#85632=CARTESIAN_POINT('Ctrl Pts',(-0.326915669375897,0.119325036287693,
-1.14836850412771));
#85633=CARTESIAN_POINT('Ctrl Pts',(-0.277849345209651,-0.209552047287046,
-1.13251418372872));
#85634=CARTESIAN_POINT('Ctrl Pts',(0.0248752910748828,-0.347121792847813,
-1.11665986332974));
#85635=CARTESIAN_POINT('Ctrl Pts',(0.304890410662428,-0.167792004142087,
-1.10080554293075));
#85636=CARTESIAN_POINT('Ctrl Pts',(0.306560490777213,0.164720929639658,
-1.08495122253177));
#85637=CARTESIAN_POINT('Ctrl Pts',(0.0283608573205941,0.346854408854388,
-1.06909690213278));
#85638=CARTESIAN_POINT('Ctrl Pts',(-0.275730387268151,0.212332457964726,
-1.0532425817338));
#85639=CARTESIAN_POINT('Ctrl Pts',(-0.328097789970408,-0.116035164432605,
-1.03738826133481));
#85640=CARTESIAN_POINT('Ctrl Pts',(-0.0809333310465426,-0.338470257326172,
-1.02153394093583));
#85641=CARTESIAN_POINT('Ctrl Pts',(0.240117975205065,-0.251904103086773,
-1.00567962053684));
#85642=CARTESIAN_POINT('Ctrl Pts',(0.341957246746726,0.0646340511336335,
-0.989825300137861));
#85643=CARTESIAN_POINT('Ctrl Pts',(0.13161187747142,0.322165536451435,-0.973970979738877));
#85644=CARTESIAN_POINT('Ctrl Pts',(-0.198886543352222,0.285580920304504,
-0.958116659339892));
#85645=CARTESIAN_POINT('Ctrl Pts',(-0.34781453485915,-0.0117204312753678,
-0.942262338940907));
#85646=CARTESIAN_POINT('Ctrl Pts',(-0.179210563908882,-0.298321794296082,
-0.926408018541922));
#85647=CARTESIAN_POINT('Ctrl Pts',(0.153000951717736,-0.312574835746634,
-0.910553698142936));
#85648=CARTESIAN_POINT('Ctrl Pts',(0.34553258744391,-0.041467459325178,
-0.894699377743952));
#85649=CARTESIAN_POINT('Ctrl Pts',(0.222615529720825,0.267497000162033,
-0.878845057344966));
#85650=CARTESIAN_POINT('Ctrl Pts',(-0.103534972672222,0.332254162656138,
-0.86299073694598));
#85651=CARTESIAN_POINT('Ctrl Pts',(-0.33516480453355,0.0936849666198187,
-0.847136416546997));
#85652=CARTESIAN_POINT('Ctrl Pts',(-0.260811051858304,-0.230412487502598,
-0.83128209614801));
#85653=CARTESIAN_POINT('Ctrl Pts',(0.0516461635162027,-0.344158383542559,
-0.815427775749027));
#85654=CARTESIAN_POINT('Ctrl Pts',(0.316953803438588,-0.14371014457714,
-0.799573455350039));
#85655=CARTESIAN_POINT('Ctrl Pts',(0.292903313877147,0.187936073940996,
-0.783719134951057));
#85656=CARTESIAN_POINT('Ctrl Pts',(0.00145122161013225,0.348008926788391,
-0.767864814552071));
#85657=CARTESIAN_POINT('Ctrl Pts',(-0.291325741240603,0.190372350038505,
-0.752010494153085));
#85658=CARTESIAN_POINT('Ctrl Pts',(-0.318141322207485,-0.141061753401278,
-0.7361561737541));
#85659=CARTESIAN_POINT('Ctrl Pts',(-0.0545146465844214,-0.343715685525617,
-0.720301853355115));
#85660=CARTESIAN_POINT('Ctrl Pts',(0.258880342256552,-0.232579637031489,
-0.704447532956129));
#85661=CARTESIAN_POINT('Ctrl Pts',(0.335934480213866,0.0908864355776483,
-0.688593212557146));
#85662=CARTESIAN_POINT('Ctrl Pts',(0.106302369988512,0.331379126233676,
-0.672738892158159));
#85663=CARTESIAN_POINT('Ctrl Pts',(-0.220376863842449,0.269344309484226,
-0.656884571759176));
#85664=CARTESIAN_POINT('Ctrl Pts',(-0.345866408793984,-0.0385842770636646,
-0.641030251360189));
#85665=CARTESIAN_POINT('Ctrl Pts',(-0.155602503197914,-0.311287937715406,
-0.625175930961206));
#85666=CARTESIAN_POINT('Ctrl Pts',(0.176716328951713,-0.29980603437955,
-0.609321610562219));
#85667=CARTESIAN_POINT('Ctrl Pts',(0.347704690099108,-0.0146207951793645,
-0.593467290163235));
#85668=CARTESIAN_POINT('Ctrl Pts',(0.201261369883626,0.283912275467464,
-0.577612969764248));
#85669=CARTESIAN_POINT('Ctrl Pts',(-0.128920441225498,0.323251974476187,
-0.561758649365265));
#85670=CARTESIAN_POINT('Ctrl Pts',(-0.341406306362706,0.0674837250343271,
-0.545904328966279));
#85671=CARTESIAN_POINT('Ctrl Pts',(-0.242210503283238,-0.249892759534263,
-0.530050008567293));
#85672=CARTESIAN_POINT('Ctrl Pts',(0.0781076760243074,-0.339133469469571,
-0.51419568816831));
#85673=CARTESIAN_POINT('Ctrl Pts',(0.327118646563388,-0.11876746288535,
-0.498341367769324));
#85674=CARTESIAN_POINT('Ctrl Pts',(0.277491649474946,0.210025483307604,
-0.482487047370338));
#85675=CARTESIAN_POINT('Ctrl Pts',(-0.0254671068945446,0.347078875234931,
-0.466632726971353));
#85676=CARTESIAN_POINT('Ctrl Pts',(-0.305176057369077,0.167271913914455,
-0.450778406572368));
#85677=CARTESIAN_POINT('Ctrl Pts',(-0.306279191543379,-0.165243384082869,
-0.434924086173383));
#85678=CARTESIAN_POINT('Ctrl Pts',(-0.0277694200554746,-0.346902260699368,
-0.419069765774398));
#85679=CARTESIAN_POINT('Ctrl Pts',(0.276092019101493,-0.211862021618632,
-0.403215445375414));
#85680=CARTESIAN_POINT('Ctrl Pts',(0.327899469835099,0.116594411325117,
-0.387361124976428));
#85681=CARTESIAN_POINT('Ctrl Pts',(0.0803561128205185,0.338607758818632,
-0.371506804577444));
#85682=CARTESIAN_POINT('Ctrl Pts',(-0.240547130003191,0.251494329378168,
-0.355652484178459));
#85683=CARTESIAN_POINT('Ctrl Pts',(-0.3418465458233,-0.0652170035607345,
-0.339798163779473));
#85684=CARTESIAN_POINT('Ctrl Pts',(-0.131062387328152,-0.322389469784616,
-0.323943843380488));
#85685=CARTESIAN_POINT('Ctrl Pts',(0.199373181323377,-0.285241398614689,
-0.308089522981502));
#85686=CARTESIAN_POINT('Ctrl Pts',(0.347794038139249,0.0123134479677662,
-0.292235202582517));
#85687=CARTESIAN_POINT('Ctrl Pts',(0.178701671076287,0.29862691833518,-0.276380882183532));
#85688=CARTESIAN_POINT('Ctrl Pts',(-0.153533705196059,0.312313512879442,
-0.260526561784547));
#85689=CARTESIAN_POINT('Ctrl Pts',(-0.3456027359991,0.0408782524840959,
-0.244672241385563));
#85690=CARTESIAN_POINT('Ctrl Pts',(-0.222159216544815,-0.267876168725123,
-0.228817920986577));
#85691=CARTESIAN_POINT('Ctrl Pts',(0.104101515480821,-0.33207716521771,
-0.212963600587593));
#85692=CARTESIAN_POINT('Ctrl Pts',(0.335323687723963,-0.0931133359829788,
-0.197109280188608));
#85693=CARTESIAN_POINT('Ctrl Pts',(0.260418510715598,0.230856786128936,
-0.181254959789622));
#85694=CARTESIAN_POINT('Ctrl Pts',(-0.0522342203577671,0.344069932773126,
-0.165400639390636));
#85695=CARTESIAN_POINT('Ctrl Pts',(-0.317195826088459,0.143169315379424,
-0.149546318991652));
#85696=CARTESIAN_POINT('Ctrl Pts',(-0.292587317374861,-0.188434816010044,
-0.133691998592666));
#85697=CARTESIAN_POINT('Ctrl Pts',(-0.000848558559683781,-0.348011645810298,
-0.117837678193682));
#85698=CARTESIAN_POINT('Ctrl Pts',(0.291632144245519,-0.189873920924492,
-0.101983357794696));
#85699=CARTESIAN_POINT('Ctrl Pts',(0.317934292326678,0.141601245974372,
-0.0861290373957114));
#85700=CARTESIAN_POINT('Ctrl Pts',(0.053863613003659,0.343813387521854,
-0.0702747169967265));
#85701=CARTESIAN_POINT('Ctrl Pts',(-0.259152079311164,0.23212774337634,
-0.0544203965977413));
#85702=CARTESIAN_POINT('Ctrl Pts',(-0.336020489789599,-0.0914385975404377,
-0.0385660761987564));
#85703=CARTESIAN_POINT('Ctrl Pts',(-0.105205732345383,-0.331647457026574,
-0.0227091807962312));
#85704=CARTESIAN_POINT('Ctrl Pts',(0.111436149755356,-0.289721825580918,
-0.0121370588600346));
#85705=CARTESIAN_POINT('Ctrl Pts',(0.187040033746796,-0.227581124687426,
-0.00684971039016626));
#85706=CARTESIAN_POINT('Ctrl Pts',(-0.289031747819831,-0.055539659978255,
-0.04));
#85707=CARTESIAN_POINT('Ctrl Pts',(-0.288640713323037,-0.0572777523841593,
-0.04));
#85708=CARTESIAN_POINT('Ctrl Pts',(-0.288249678826243,-0.0590158447900636,
-0.04));
#85709=CARTESIAN_POINT('Ctrl Pts',(-0.287858644329449,-0.0607539371959678,
-0.04));
#85710=CARTESIAN_POINT('Ctrl Pts',(-0.13799857747695,-0.193363938662942,
-1.5608));
#85711=CARTESIAN_POINT('Ctrl Pts',(-0.143347841422346,-0.190455713481887,
-1.5608));
#85712=CARTESIAN_POINT('Ctrl Pts',(-0.148566997856137,-0.187334258556034,
-1.5608));
#85713=CARTESIAN_POINT('Ctrl Pts',(-0.15364167413773,-0.184002459902945,
-1.5608));
#85714=CARTESIAN_POINT('Ctrl Pts',(-0.163907115485033,-0.177262644049398,
-1.5608));
#85715=CARTESIAN_POINT('Ctrl Pts',(-0.173582104512979,-0.169663735623815,
-1.5608));
#85716=CARTESIAN_POINT('Ctrl Pts',(-0.182636032389057,-0.161324058116206,
-1.5608));
#85717=CARTESIAN_POINT('Ctrl Pts',(-0.188173868816878,-0.156223093040049,
-1.5608));
#85718=CARTESIAN_POINT('Ctrl Pts',(-0.193479882338644,-0.150842423408572,
-1.5608));
#85719=CARTESIAN_POINT('Ctrl Pts',(-0.198524103660284,-0.145232040158292,
-1.5608));
#85720=CARTESIAN_POINT('Ctrl Pts',(-0.206390733930232,-0.136482461603259,
-1.5608));
#85721=CARTESIAN_POINT('Ctrl Pts',(-0.213635127195895,-0.127163051947901,
-1.5608));
#85722=CARTESIAN_POINT('Ctrl Pts',(-0.220229011985289,-0.117368722208056,
-1.5608));
#85723=CARTESIAN_POINT('Ctrl Pts',(-0.223143397241071,-0.113039794558308,
-1.5608));
#85724=CARTESIAN_POINT('Ctrl Pts',(-0.225930582649798,-0.108617881329991,
-1.5608));
#85725=CARTESIAN_POINT('Ctrl Pts',(-0.228587451034113,-0.104110300495371,
-1.5608));
#85726=CARTESIAN_POINT('Ctrl Pts',(-0.230967501738554,-0.10007236206978,
-1.5608));
#85727=CARTESIAN_POINT('Ctrl Pts',(-0.233238383225063,-0.0959733682384296,
-1.5608));
#85728=CARTESIAN_POINT('Ctrl Pts',(-0.235397692200457,-0.0918213261469215,
-1.5608));
#85729=CARTESIAN_POINT('Ctrl Pts',(-0.242841770000136,-0.0775074300306483,
-1.5608));
#85730=CARTESIAN_POINT('Ctrl Pts',(-0.24896693470216,-0.0625588879644513,
-1.5608));
#85731=CARTESIAN_POINT('Ctrl Pts',(-0.253699085536977,-0.047196706931204,
-1.5608));
#85732=CARTESIAN_POINT('Ctrl Pts',(-0.256802926190838,-0.0371205779811004,
-1.5608));
#85733=CARTESIAN_POINT('Ctrl Pts',(-0.259306827718714,-0.0268655758638595,
-1.5608));
#85734=CARTESIAN_POINT('Ctrl Pts',(-0.261179689706241,-0.0164868296819522,
-1.5608));
#85735=CARTESIAN_POINT('Ctrl Pts',(-0.262261665440453,-0.0104908985374452,
-1.5608));
#85736=CARTESIAN_POINT('Ctrl Pts',(-0.263132275784059,-0.00445291160850025,
-1.5608));
#85737=CARTESIAN_POINT('Ctrl Pts',(-0.263782798320229,0.00158770973103373,
-1.5608));
#85738=CARTESIAN_POINT('Ctrl Pts',(-0.264886445795179,0.0118359580511637,
-1.5608));
#85739=CARTESIAN_POINT('Ctrl Pts',(-0.265361036560997,0.0221109639333779,
-1.5608));
#85740=CARTESIAN_POINT('Ctrl Pts',(-0.265185866874642,0.0323592383439703,
-1.5608));
#85741=CARTESIAN_POINT('Ctrl Pts',(-0.264987655497751,0.0439555631644492,
-1.5608));
#85742=CARTESIAN_POINT('Ctrl Pts',(-0.263958005355191,0.0555178554776766,
-1.5608));
#85743=CARTESIAN_POINT('Ctrl Pts',(-0.262149841841104,0.0669878505690906,
-1.5608));
#85744=CARTESIAN_POINT('Ctrl Pts',(-0.261038096613289,0.0740401509869451,
-1.5608));
#85745=CARTESIAN_POINT('Ctrl Pts',(-0.259631739078235,0.0810576215322809,
-1.5608));
#85746=CARTESIAN_POINT('Ctrl Pts',(-0.25794033900309,0.0880268053398159,
-1.5608));
#85747=CARTESIAN_POINT('Ctrl Pts',(-0.256631126704129,0.0934212364319209,
-1.5608));
#85748=CARTESIAN_POINT('Ctrl Pts',(-0.255151399390779,0.0987837905468475,
-1.5608));
#85749=CARTESIAN_POINT('Ctrl Pts',(-0.253512272984399,0.104089767724613,
-1.5608));
#85750=CARTESIAN_POINT('Ctrl Pts',(-0.248424210607189,0.120560213656933,
-1.5608));
#85751=CARTESIAN_POINT('Ctrl Pts',(-0.241793533995896,0.13653471216082,
-1.5608));
#85752=CARTESIAN_POINT('Ctrl Pts',(-0.233782283533326,0.151832188232471,
-1.5608));
#85753=CARTESIAN_POINT('Ctrl Pts',(-0.229722814977607,0.159583740051364,
-1.5608));
#85754=CARTESIAN_POINT('Ctrl Pts',(-0.225307871711475,0.167161501680917,
-1.5608));
#85755=CARTESIAN_POINT('Ctrl Pts',(-0.220552921268545,0.174541049986005,
-1.5608));
#85756=CARTESIAN_POINT('Ctrl Pts',(-0.217270098793488,0.179635897413433,
-1.5608));
#85757=CARTESIAN_POINT('Ctrl Pts',(-0.213823767062381,0.184638075610162,
-1.5608));
#85758=CARTESIAN_POINT('Ctrl Pts',(-0.210222729269013,0.189532882285389,
-1.5608));
#85759=CARTESIAN_POINT('Ctrl Pts',(-0.206848865553593,0.194118896535493,
-1.5608));
#85760=CARTESIAN_POINT('Ctrl Pts',(-0.203344351977369,0.198603678931769,
-1.5608));
#85761=CARTESIAN_POINT('Ctrl Pts',(-0.199718097012662,0.202976801403612,
-1.5608));
#85762=CARTESIAN_POINT('Ctrl Pts',(-0.188601077808648,0.216383494251783,
-1.5608));
#85763=CARTESIAN_POINT('Ctrl Pts',(-0.176331421703839,0.228758241429328,
-1.5608));
#85764=CARTESIAN_POINT('Ctrl Pts',(-0.163036176043001,0.239920308741562,
-1.5608));
#85765=CARTESIAN_POINT('Ctrl Pts',(-0.15230812646604,0.248927078120766,
-1.5608));
#85766=CARTESIAN_POINT('Ctrl Pts',(-0.140911166079345,0.257144449634528,
-1.5608));
#85767=CARTESIAN_POINT('Ctrl Pts',(-0.128892185405328,0.264462557919714,
-1.5608));
#85768=CARTESIAN_POINT('Origin',(-3.51939854619125E-17,0.,-1.5608));
#85769=CARTESIAN_POINT('',(-0.2942,-3.60291088309151E-17,-1.5608));
#85770=CARTESIAN_POINT('Origin',(0.,0.,-1.5608));
#85771=CARTESIAN_POINT('',(0.133736061201431,0.262046381265468,-1.5608));
#85772=CARTESIAN_POINT('Origin',(0.,0.,-1.5608));
#85773=CARTESIAN_POINT('Ctrl Pts',(0.13373606120143,0.262046381265467,-1.5608));
#85774=CARTESIAN_POINT('Ctrl Pts',(0.138550012611077,0.259017157142651,
-1.5608));
#85775=CARTESIAN_POINT('Ctrl Pts',(0.143264321808573,0.255840579156758,
-1.5608));
#85776=CARTESIAN_POINT('Ctrl Pts',(0.147871259490879,0.252516190150327,
-1.5608));
#85777=CARTESIAN_POINT('Ctrl Pts',(0.157320856382195,0.245697314318481,
-1.5608));
#85778=CARTESIAN_POINT('Ctrl Pts',(0.166319266874593,0.238256907737579,
-1.5608));
#85779=CARTESIAN_POINT('Ctrl Pts',(0.174835840546171,0.230258755145514,
-1.5608));
#85780=CARTESIAN_POINT('Ctrl Pts',(0.179702443415592,0.225688392244233,
-1.5608));
#85781=CARTESIAN_POINT('Ctrl Pts',(0.184412787467239,0.220934445028738,
-1.5608));
#85782=CARTESIAN_POINT('Ctrl Pts',(0.18895591579128,0.216012380917119,-1.5608));
#85783=CARTESIAN_POINT('Ctrl Pts',(0.19523865863058,0.209205603550034,-1.5608));
#85784=CARTESIAN_POINT('Ctrl Pts',(0.201189436575403,0.202090872429547,
-1.5608));
#85785=CARTESIAN_POINT('Ctrl Pts',(0.20678943857,0.194705868097706,-1.5608));
#85786=CARTESIAN_POINT('Ctrl Pts',(0.212443879605949,0.187249072263542,
-1.5608));
#85787=CARTESIAN_POINT('Ctrl Pts',(0.21774229688384,0.179514930803699,-1.5608));
#85788=CARTESIAN_POINT('Ctrl Pts',(0.222665799064572,0.171535487495526,
-1.5608));
#85789=CARTESIAN_POINT('Ctrl Pts',(0.226114144708047,0.165946807413943,
-1.5608));
#85790=CARTESIAN_POINT('Ctrl Pts',(0.229379510809365,0.160235806619833,
-1.5608));
#85791=CARTESIAN_POINT('Ctrl Pts',(0.232450764193899,0.154419684787329,
-1.5608));
#85792=CARTESIAN_POINT('Ctrl Pts',(0.23528691598115,0.149048781685295,-1.5608));
#85793=CARTESIAN_POINT('Ctrl Pts',(0.237953497096427,0.14359591196093,-1.5608));
#85794=CARTESIAN_POINT('Ctrl Pts',(0.240443806796245,0.138075597522685,
-1.5608));
#85795=CARTESIAN_POINT('Ctrl Pts',(0.247289923459264,0.122899687207787,
-1.5608));
#85796=CARTESIAN_POINT('Ctrl Pts',(0.25281522573498,0.107199566527781,-1.5608));
#85797=CARTESIAN_POINT('Ctrl Pts',(0.256905339126335,0.0911583963714125,
-1.5608));
#85798=CARTESIAN_POINT('Ctrl Pts',(0.259577627326119,0.0806778483723795,
-1.5608));
#85799=CARTESIAN_POINT('Ctrl Pts',(0.261636317517558,0.0700514990909618,
-1.5608));
#85800=CARTESIAN_POINT('Ctrl Pts',(0.263037088781112,0.0593310937249914,
-1.5608));
#85801=CARTESIAN_POINT('Ctrl Pts',(0.263736056624588,0.0539817416824344,
-1.5608));
#85802=CARTESIAN_POINT('Ctrl Pts',(0.26427047436316,0.0486102636085355,
-1.5608));
#85803=CARTESIAN_POINT('Ctrl Pts',(0.264633964208612,0.043242546357013,
-1.5608));
#85804=CARTESIAN_POINT('Ctrl Pts',(0.265344592360124,0.0327485778568958,
-1.5608));
#85805=CARTESIAN_POINT('Ctrl Pts',(0.265405260271088,0.0222518652651568,
-1.5608));
#85806=CARTESIAN_POINT('Ctrl Pts',(0.264782683669769,0.0118008989594462,
-1.5608));
#85807=CARTESIAN_POINT('Ctrl Pts',(0.263877775160184,-0.00338947010257891,
-1.5608));
#85808=CARTESIAN_POINT('Ctrl Pts',(0.261530657070704,-0.0184845232811562,
-1.5608));
#85809=CARTESIAN_POINT('Ctrl Pts',(0.257827438680858,-0.0333213284021663,
-1.5608));
#85810=CARTESIAN_POINT('Ctrl Pts',(0.255791351029307,-0.0414788369569387,
-1.5608));
#85811=CARTESIAN_POINT('Ctrl Pts',(0.253340030824081,-0.0495684731839285,
-1.5608));
#85812=CARTESIAN_POINT('Ctrl Pts',(0.250506238567754,-0.0575042321542823,
-1.5608));
#85813=CARTESIAN_POINT('Ctrl Pts',(0.245534376020338,-0.0714274485516459,
-1.5608));
#85814=CARTESIAN_POINT('Ctrl Pts',(0.239384092384913,-0.0849048911441926,
-1.5608));
#85815=CARTESIAN_POINT('Ctrl Pts',(0.232141482928074,-0.0977877984656227,
-1.5608));
#85816=CARTESIAN_POINT('Ctrl Pts',(0.226804087220809,-0.107281776381215,
-1.5608));
#85817=CARTESIAN_POINT('Ctrl Pts',(0.220873249583642,-0.116451756653311,
-1.5608));
#85818=CARTESIAN_POINT('Ctrl Pts',(0.214372210700434,-0.125230152591395,
-1.5608));
#85819=CARTESIAN_POINT('Ctrl Pts',(0.210401710388729,-0.130591545506374,
-1.5608));
#85820=CARTESIAN_POINT('Ctrl Pts',(0.206215774074286,-0.135808510284193,
-1.5608));
#85821=CARTESIAN_POINT('Ctrl Pts',(0.201844453986288,-0.140836689913866,
-1.5608));
#85822=CARTESIAN_POINT('Ctrl Pts',(0.192116839118631,-0.152026031791883,
-1.5608));
#85823=CARTESIAN_POINT('Ctrl Pts',(0.181455103880824,-0.162311068884459,
-1.5608));
#85824=CARTESIAN_POINT('Ctrl Pts',(0.169933457476246,-0.171520717268733,
-1.5608));
#85825=CARTESIAN_POINT('Ctrl Pts',(0.160599905043598,-0.178981346857809,
-1.5608));
#85826=CARTESIAN_POINT('Ctrl Pts',(0.150701251204416,-0.185735832894192,
-1.5608));
#85827=CARTESIAN_POINT('Ctrl Pts',(0.140268421710186,-0.191669440498754,
-1.5608));
#85828=CARTESIAN_POINT('Ctrl Pts',(0.139416665144678,-0.1921538718064,-1.5608));
#85829=CARTESIAN_POINT('Ctrl Pts',(0.138561345670519,-0.192632817908258,
-1.5608));
#85830=CARTESIAN_POINT('Ctrl Pts',(0.137702479013106,-0.193106208855762,
-1.5608));
#85831=CARTESIAN_POINT('Ctrl Pts',(0.170904886030586,-0.239913673682597,
-1.59394040064334));
#85832=CARTESIAN_POINT('Ctrl Pts',(0.250610379973567,-0.183139249212075,
-1.58865305194158));
#85833=CARTESIAN_POINT('Ctrl Pts',(0.34758798138322,0.0150557195712735,
-1.57808092977351));
#85834=CARTESIAN_POINT('Ctrl Pts',(0.175911135758696,0.300519364992409,
-1.56222403413909));
#85835=CARTESIAN_POINT('Ctrl Pts',(-0.156485212151456,0.310711293896572,
-1.54636971374011));
#85836=CARTESIAN_POINT('Ctrl Pts',(-0.345940875846988,0.0376795876694137,
-1.53051539334112));
#85837=CARTESIAN_POINT('Ctrl Pts',(-0.219616959829241,-0.269976713895109,
-1.51466107294214));
#85838=CARTESIAN_POINT('Ctrl Pts',(0.107224807406404,-0.331044119307512,
-1.49880675254315));
#85839=CARTESIAN_POINT('Ctrl Pts',(0.33616586372552,-0.089951456236232,
-1.48295243214416));
#85840=CARTESIAN_POINT('Ctrl Pts',(0.258215431334032,0.233293241644007,
-1.46709811174518));
#85841=CARTESIAN_POINT('Ctrl Pts',(-0.0554719698132699,0.343539578459029,
-1.45124379134619));
#85842=CARTESIAN_POINT('Ctrl Pts',(-0.318515442143559,0.140165531986085,
-1.43538947094721));
#85843=CARTESIAN_POINT('Ctrl Pts',(-0.290775969960518,-0.19117511072713,
-1.41953515054822));
#85844=CARTESIAN_POINT('Ctrl Pts',(0.00242342836231637,-0.34798294308962,
-1.40368083014924));
#85845=CARTESIAN_POINT('Ctrl Pts',(0.29341015959215,-0.187106331189504,
-1.38782650975025));
#85846=CARTESIAN_POINT('Ctrl Pts',(0.31653269414384,0.144586806748901,-1.37197218935127));
#85847=CARTESIAN_POINT('Ctrl Pts',(0.0506814801073806,0.344281283774666,
-1.35611786895228));
#85848=CARTESIAN_POINT('Ctrl Pts',(-0.26143858271537,0.229669606964089,
-1.3402635485533));
#85849=CARTESIAN_POINT('Ctrl Pts',(-0.334882305766732,-0.0946155212339324,
-1.32440922815431));
#85850=CARTESIAN_POINT('Ctrl Pts',(-0.102600337987051,-0.332522806167084,
-1.30855490775533));
#85851=CARTESIAN_POINT('Ctrl Pts',(0.223349035049687,-0.266858504519963,
-1.29270058735634));
#85852=CARTESIAN_POINT('Ctrl Pts',(0.345395323465393,0.042430202855741,
-1.27684626695736));
#85853=CARTESIAN_POINT('Ctrl Pts',(0.152118230161139,0.312982898076324,
-1.26099194655837));
#85854=CARTESIAN_POINT('Ctrl Pts',(-0.180032875201427,0.297802644874621,
-1.24513762615939));
#85855=CARTESIAN_POINT('Ctrl Pts',(-0.347825719725829,0.0107480176866395,
-1.2292833057604));
#85856=CARTESIAN_POINT('Ctrl Pts',(-0.198076390550669,-0.286118846923063,
-1.21342898536142));
#85857=CARTESIAN_POINT('Ctrl Pts',(0.132503751226997,-0.321777884749036,
-1.19757466496243));
#85858=CARTESIAN_POINT('Ctrl Pts',(0.342116618997376,-0.0636747215274613,
-1.18172034456345));
#85859=CARTESIAN_POINT('Ctrl Pts',(0.239399349463731,0.252559305152815,
-1.16586602416446));
#85860=CARTESIAN_POINT('Ctrl Pts',(-0.081873896380812,0.338223175217988,
-1.15001170376548));
#85861=CARTESIAN_POINT('Ctrl Pts',(-0.3284016201621,0.11511136794454,-1.13415738336649));
#85862=CARTESIAN_POINT('Ctrl Pts',(-0.275120105184066,-0.213089602931875,
-1.1183030629675));
#85863=CARTESIAN_POINT('Ctrl Pts',(0.0293281039782686,-0.346753678385599,
-1.10244874256852));
#85864=CARTESIAN_POINT('Ctrl Pts',(0.307001668962005,-0.163854284076304,
-1.08659442216953));
#85865=CARTESIAN_POINT('Ctrl Pts',(0.304402753490565,0.168633373989131,
-1.07074010177055));
#85866=CARTESIAN_POINT('Ctrl Pts',(0.0239039977140675,0.347169771220429,
-1.05488578137156));
#85867=CARTESIAN_POINT('Ctrl Pts',(-0.27841754734824,0.20876283310098,-1.03903146097258));
#85868=CARTESIAN_POINT('Ctrl Pts',(-0.326562048809314,-0.120230942079134,
-1.02317714057359));
#85869=CARTESIAN_POINT('Ctrl Pts',(-0.0765767200594529,-0.33946171669388,
-1.00732282017461));
#85870=CARTESIAN_POINT('Ctrl Pts',(0.243318154618006,-0.248786106503311,
-0.991468499775624));
#85871=CARTESIAN_POINT('Ctrl Pts',(0.341079439712692,0.069014976353469,
-0.975614179376641));
#85872=CARTESIAN_POINT('Ctrl Pts',(0.127457464502766,0.323809891600497,
-0.959759858977655));
#85873=CARTESIAN_POINT('Ctrl Pts',(-0.20252485444545,0.28298751648729,-0.94390553857867));
#85874=CARTESIAN_POINT('Ctrl Pts',(-0.347615203584335,-0.0161839856901046,
-0.928051218179684));
#85875=CARTESIAN_POINT('Ctrl Pts',(-0.175355566706118,-0.300580565541041,
-0.9121968977807));
#85876=CARTESIAN_POINT('Ctrl Pts',(0.156992254084647,-0.310566713144241,
-0.896342577381714));
#85877=CARTESIAN_POINT('Ctrl Pts',(0.346016396495308,-0.0370257277065219,
-0.88048825698273));
#85878=CARTESIAN_POINT('Ctrl Pts',(0.219150159379363,0.270317329817745,
-0.864633936583744));
#85879=CARTESIAN_POINT('Ctrl Pts',(-0.107785865529432,0.33087831350493,
-0.84877961618476));
#85880=CARTESIAN_POINT('Ctrl Pts',(-0.336320432257163,0.0893689991112763,
-0.832925295785774));
#85881=CARTESIAN_POINT('Ctrl Pts',(-0.257816401784462,-0.233728376811007,
-0.81707097538679));
#85882=CARTESIAN_POINT('Ctrl Pts',(0.056057171382673,-0.343447004197692,
-0.801216654987804));
#85883=CARTESIAN_POINT('Ctrl Pts',(0.318754206898361,-0.13962093947683,
-0.785362334588819));
#85884=CARTESIAN_POINT('Ctrl Pts',(0.290449462114917,0.191669927513295,
-0.769508014189834));
#85885=CARTESIAN_POINT('Ctrl Pts',(-0.00301667892052102,0.347978664294359,
-0.753653693790849));
#85886=CARTESIAN_POINT('Ctrl Pts',(-0.293728789052321,0.186605599159438,
-0.737799373391864));
#85887=CARTESIAN_POINT('Ctrl Pts',(-0.316285691536655,-0.145126195033759,
-0.721945052992879));
#85888=CARTESIAN_POINT('Ctrl Pts',(-0.0500944070844066,-0.344367248057443,
-0.706090732593894));
#85889=CARTESIAN_POINT('Ctrl Pts',(0.261829800507703,-0.22922348640986,
-0.690236412194909));
#85890=CARTESIAN_POINT('Ctrl Pts',(0.334720494395002,0.0951863529491743,
-0.674382091795923));
#85891=CARTESIAN_POINT('Ctrl Pts',(0.102033229894396,0.332697266524855,
-0.658527771396939));
#85892=CARTESIAN_POINT('Ctrl Pts',(-0.223803712026459,0.266477296667027,
-0.642673450997953));
#85893=CARTESIAN_POINT('Ctrl Pts',(-0.345322476405579,-0.0430190474666505,
-0.626819130598969));
#85894=CARTESIAN_POINT('Ctrl Pts',(-0.151584364995733,-0.313241809860391,
-0.610964810199983));
#85895=CARTESIAN_POINT('Ctrl Pts',(0.180540375122247,-0.297495250561208,
-0.595110489800998));
#85896=CARTESIAN_POINT('Ctrl Pts',(0.347843539746289,-0.0101549501589795,
-0.579256169402013));
#85897=CARTESIAN_POINT('Ctrl Pts',(0.197588262343984,0.286456156749127,
-0.563401849003027));
#85898=CARTESIAN_POINT('Ctrl Pts',(-0.133052198574159,0.321551494492247,
-0.547547528604043));
#85899=CARTESIAN_POINT('Ctrl Pts',(-0.342224688814901,0.0630913109900864,
-0.531693208205058));
#85900=CARTESIAN_POINT('Ctrl Pts',(-0.238968381085131,-0.252967120384663,
-0.515838887806072));
#85901=CARTESIAN_POINT('Ctrl Pts',(0.0824504569657546,-0.338083086387494,
-0.499984567407088));
#85902=CARTESIAN_POINT('Ctrl Pts',(0.328597410795141,-0.114551267045994,
-0.484130247008102));
#85903=CARTESIAN_POINT('Ctrl Pts',(0.274756381763336,0.213558380362958,
-0.468275926609118));
#85904=CARTESIAN_POINT('Ctrl Pts',(-0.0299192856409278,0.346703169155593,
-0.452421606210132));
#85905=CARTESIAN_POINT('Ctrl Pts',(-0.30728059875184,0.163330599807569,
-0.436567285811148));
#85906=CARTESIAN_POINT('Ctrl Pts',(-0.304114786438363,-0.169152143727808,
-0.420712965412162));
#85907=CARTESIAN_POINT('Ctrl Pts',(-0.0233120294769848,-0.347210023571681,
-0.404858645013177));
#85908=CARTESIAN_POINT('Ctrl Pts',(0.278773089448442,-0.208287820207959,
-0.389004324614192));
#85909=CARTESIAN_POINT('Ctrl Pts',(0.326356576077487,0.120787564287852,
-0.373150004215206));
#85910=CARTESIAN_POINT('Ctrl Pts',(0.0759978194502111,0.339591788806732,
-0.357295683816222));
#85911=CARTESIAN_POINT('Ctrl Pts',(-0.243741991839324,0.248370880552563,
-0.341441363417237));
#85912=CARTESIAN_POINT('Ctrl Pts',(-0.340961264081266,-0.0695964249972271,
-0.325587043018251));
#85913=CARTESIAN_POINT('Ctrl Pts',(-0.126905188939026,-0.324026740554483,
-0.309732722619267));
#85914=CARTESIAN_POINT('Ctrl Pts',(0.203007088642323,-0.282641792479861,
-0.293878402220281));
#85915=CARTESIAN_POINT('Ctrl Pts',(0.34758705207047,0.0167766509282329,
-0.278024081821296));
#85916=CARTESIAN_POINT('Ctrl Pts',(0.174842913459877,0.300879123171855,
-0.262169761422311));
#85917=CARTESIAN_POINT('Ctrl Pts',(-0.157521740789639,0.310298569287209,
-0.246315441023326));
#85918=CARTESIAN_POINT('Ctrl Pts',(-0.346078659673261,0.0364357380205341,
-0.230461120624341));
#85919=CARTESIAN_POINT('Ctrl Pts',(-0.218689637670251,-0.270690653779669,
-0.214606800225356));
#85920=CARTESIAN_POINT('Ctrl Pts',(0.108351193813394,-0.330693940132053,
-0.198752479826371));
#85921=CARTESIAN_POINT('Ctrl Pts',(0.336469780852948,-0.0887956529090298,
-0.182898159427386));
#85922=CARTESIAN_POINT('Ctrl Pts',(0.257422366521119,0.23416803964345,-0.1670438390284));
#85923=CARTESIAN_POINT('Ctrl Pts',(-0.0566519505980647,0.343350125828982,
-0.151189518629416));
#85924=CARTESIAN_POINT('Ctrl Pts',(-0.318974075534328,0.139078781230093,
-0.13533519823043));
#85925=CARTESIAN_POINT('Ctrl Pts',(-0.290156119492426,-0.192167794938009,
-0.119480877831445));
#85926=CARTESIAN_POINT('Ctrl Pts',(0.00367478997105658,-0.347967436446841,
-0.10362655743246));
#85927=CARTESIAN_POINT('Ctrl Pts',(0.29392225292049,-0.1861151230156,-0.0877722370334754));
#85928=CARTESIAN_POINT('Ctrl Pts',(0.316279104812747,0.145685085984127,
-0.0719179166344901));
#85929=CARTESIAN_POINT('Ctrl Pts',(0.0490122977774616,0.344418191703448,
-0.0560635962355054));
#85930=CARTESIAN_POINT('Ctrl Pts',(-0.157657690967761,0.267353546877372,
-0.0454940493028484));
#85931=CARTESIAN_POINT('Ctrl Pts',(-0.221960000566811,0.193651260363756,
-0.04020927583652));
#85932=CARTESIAN_POINT('Ctrl Pts',(0.159724862551269,-0.224219327154077,
-1.58281527225733));
#85933=CARTESIAN_POINT('Ctrl Pts',(0.234216290855694,-0.171158894795468,
-1.57752792355557));
#85934=CARTESIAN_POINT('Ctrl Pts',(0.324849943382959,0.0140708249774791,
-1.56695580138749));
#85935=CARTESIAN_POINT('Ctrl Pts',(0.164403620240946,0.280860397746711,
-1.55109890575308));
#85936=CARTESIAN_POINT('Ctrl Pts',(-0.146248475293588,0.290385604902334,
-1.5352445853541));
#85937=CARTESIAN_POINT('Ctrl Pts',(-0.323310585957363,0.0352147156308222,
-1.51939026495511));
#85938=CARTESIAN_POINT('Ctrl Pts',(-0.205250356133029,-0.252315744274402,
-1.50353594455613));
#85939=CARTESIAN_POINT('Ctrl Pts',(0.100210520733791,-0.309388325184188,
-1.48768162415714));
#85940=CARTESIAN_POINT('Ctrl Pts',(0.314175022289166,-0.0840671341663506,
-1.47182730375816));
#85941=CARTESIAN_POINT('Ctrl Pts',(0.241323845305763,0.218031981537731,
-1.45597298335917));
#85942=CARTESIAN_POINT('Ctrl Pts',(-0.051843179909363,0.321066373377227,
-1.44011866296019));
#85943=CARTESIAN_POINT('Ctrl Pts',(-0.297679231989491,0.130996373777726,
-1.4242643425612));
#85944=CARTESIAN_POINT('Ctrl Pts',(-0.271754382884308,-0.178669077247151,
-1.40841002216222));
#85945=CARTESIAN_POINT('Ctrl Pts',(0.00226489582050245,-0.325219068021424,
-1.39255570176323));
#85946=CARTESIAN_POINT('Ctrl Pts',(0.274216252679952,-0.174866463597575,
-1.37670138136425));
#85947=CARTESIAN_POINT('Ctrl Pts',(0.295826188702755,0.135128423599089,
-1.36084706096526));
#85948=CARTESIAN_POINT('Ctrl Pts',(0.0473660679461038,0.321759558822918,
-1.34499274056628));
#85949=CARTESIAN_POINT('Ctrl Pts',(-0.244336148952099,0.214645392864761,
-1.32913842016729));
#85950=CARTESIAN_POINT('Ctrl Pts',(-0.312975430379855,-0.0884260917010995,
-1.3132840997683));
#85951=CARTESIAN_POINT('Ctrl Pts',(-0.0958885685676773,-0.310770281317141,
-1.29742977936932));
#85952=CARTESIAN_POINT('Ctrl Pts',(0.208738291530677,-0.249401517680771,
-1.28157545897033));
#85953=CARTESIAN_POINT('Ctrl Pts',(0.322800721779757,0.0396545615316289,
-1.26572113857135));
#85954=CARTESIAN_POINT('Ctrl Pts',(0.142167166593946,0.292508608368234,
-1.24986681817236));
#85955=CARTESIAN_POINT('Ctrl Pts',(-0.168255729336558,0.278321396332049,
-1.23401249777338));
#85956=CARTESIAN_POINT('Ctrl Pts',(-0.325072129681891,0.0100449184781619,
-1.21815817737439));
#85957=CARTESIAN_POINT('Ctrl Pts',(-0.185118898529878,-0.267401913190092,
-1.20230385697541));
#85958=CARTESIAN_POINT('Ctrl Pts',(0.123835800975708,-0.300728256560079,
-1.18644953657643));
#85959=CARTESIAN_POINT('Ctrl Pts',(0.319736499143041,-0.0595093351640252,
-1.17059521617744));
#85960=CARTESIAN_POINT('Ctrl Pts',(0.223738648297707,0.236037723897242,
-1.15474089577845));
#85961=CARTESIAN_POINT('Ctrl Pts',(-0.0765179811396485,0.316097751375452,
-1.13888657537947));
#85962=CARTESIAN_POINT('Ctrl Pts',(-0.306918689455241,0.107581168976872,
-1.12303225498049));
#85963=CARTESIAN_POINT('Ctrl Pts',(-0.257122672184753,-0.199149996994861,
-1.1071779345815));
#85964=CARTESIAN_POINT('Ctrl Pts',(0.0274095579454656,-0.324070217684555,
-1.09132361418251));
#85965=CARTESIAN_POINT('Ctrl Pts',(0.28691865116829,-0.153135487289929,
-1.07546929378353));
#85966=CARTESIAN_POINT('Ctrl Pts',(0.284489748015783,0.15760194519629,-1.05961497338455));
#85967=CARTESIAN_POINT('Ctrl Pts',(0.0223402784904676,0.324459091124019,
-1.04376065298556));
#85968=CARTESIAN_POINT('Ctrl Pts',(-0.260204406760496,0.195106269910267,
-1.02790633258657));
#85969=CARTESIAN_POINT('Ctrl Pts',(-0.305199456680208,-0.112365837771089,
-1.01205201218759));
#85970=CARTESIAN_POINT('Ctrl Pts',(-0.0715673282970608,-0.317255271628942,
-0.996197691788603));
#85971=CARTESIAN_POINT('Ctrl Pts',(0.227401098384244,-0.232511355227108,
-0.980343371389616));
#85972=CARTESIAN_POINT('Ctrl Pts',(0.318767168642697,0.0645002484602125,
-0.964489050990633));
#85973=CARTESIAN_POINT('Ctrl Pts',(0.119119625375682,0.302627336349962,
-0.948634730591646));
#85974=CARTESIAN_POINT('Ctrl Pts',(-0.189276358861536,0.26447542387154,
-0.932780410192662));
#85975=CARTESIAN_POINT('Ctrl Pts',(-0.324875384799132,-0.015125283717291,
-0.916926089793677));
#85976=CARTESIAN_POINT('Ctrl Pts',(-0.163884394649323,-0.280917594761059,
-0.901071769394691));
#85977=CARTESIAN_POINT('Ctrl Pts',(0.146722348246946,-0.290250482137093,
-0.885217448995707));
#85978=CARTESIAN_POINT('Ctrl Pts',(0.323381166298586,-0.0346036289900233,
-0.869363128596721));
#85979=CARTESIAN_POINT('Ctrl Pts',(0.204814092200339,0.252634078247699,
-0.853508808197737));
#85980=CARTESIAN_POINT('Ctrl Pts',(-0.100734876319318,0.309233365840177,
-0.837654487798751));
#85981=CARTESIAN_POINT('Ctrl Pts',(-0.31431947946675,0.083522779429712,
-0.821800167399766));
#85982=CARTESIAN_POINT('Ctrl Pts',(-0.240950918928764,-0.218438651623968,
-0.805945847000781));
#85983=CARTESIAN_POINT('Ctrl Pts',(0.0523900995581144,-0.320979855013057,
-0.790091526601796));
#85984=CARTESIAN_POINT('Ctrl Pts',(0.297902377556176,-0.130487406680836,
-0.774237206202811));
#85985=CARTESIAN_POINT('Ctrl Pts',(0.271449234085044,0.17913152478153,-0.758382885803825));
#85986=CARTESIAN_POINT('Ctrl Pts',(-0.0028193379202488,0.325215069130574,
-0.742528565404841));
#85987=CARTESIAN_POINT('Ctrl Pts',(-0.274514038471294,0.174398487774677,
-0.726674245005856));
#85988=CARTESIAN_POINT('Ctrl Pts',(-0.295595344176312,-0.135632526914457,
-0.710819924606871));
#85989=CARTESIAN_POINT('Ctrl Pts',(-0.0468173992679871,-0.321839899611118,
-0.694965604207886));
#85990=CARTESIAN_POINT('Ctrl Pts',(0.244701774590776,-0.214228456018421,
-0.6791112838089));
#85991=CARTESIAN_POINT('Ctrl Pts',(0.312824204164448,0.0889595815232725,
-0.663256963409916));
#85992=CARTESIAN_POINT('Ctrl Pts',(0.0953585587812114,0.310933329064417,
-0.64740264301093));
#85993=CARTESIAN_POINT('Ctrl Pts',(-0.209163225067142,0.249045247164886,
-0.631548322611945));
#85994=CARTESIAN_POINT('Ctrl Pts',(-0.322732640129862,-0.04020488590635,
-0.615694002212961));
#85995=CARTESIAN_POINT('Ctrl Pts',(-0.14166822509411,-0.292750583013215,
-0.599839681813975));
#85996=CARTESIAN_POINT('Ctrl Pts',(0.168730030317533,-0.278034110721911,
-0.58398536141499));
#85997=CARTESIAN_POINT('Ctrl Pts',(0.325088783976481,-0.0094906474357171,
-0.568131041016005));
#85998=CARTESIAN_POINT('Ctrl Pts',(0.18466270203058,0.267717157340548,-0.55227672061702));
#85999=CARTESIAN_POINT('Ctrl Pts',(-0.124348370739959,0.300516675993317,
-0.536422400218035));
#86000=CARTESIAN_POINT('Ctrl Pts',(-0.319837499396171,0.0589640893840041,
-0.520568079819049));
#86001=CARTESIAN_POINT('Ctrl Pts',(-0.223335872422572,-0.236418861226701,
-0.504713759420064));
#86002=CARTESIAN_POINT('Ctrl Pts',(0.077056825068113,-0.315966826685613,
-0.488859439021079));
#86003=CARTESIAN_POINT('Ctrl Pts',(0.307101672122839,-0.107057707997419,
-0.473005118622095));
#86004=CARTESIAN_POINT('Ctrl Pts',(0.256782742328259,0.199588108581286,
-0.457150798223109));
#86005=CARTESIAN_POINT('Ctrl Pts',(-0.0279620664898624,0.324023012598688,
-0.441296477824125));
#86006=CARTESIAN_POINT('Ctrl Pts',(-0.287179334308354,0.152646060686708,
-0.425442157425139));
#86007=CARTESIAN_POINT('Ctrl Pts',(-0.284220618800695,-0.158086778761499,
-0.409587837026154));
#86008=CARTESIAN_POINT('Ctrl Pts',(-0.0217870348267034,-0.324496710301681,
-0.393733516627169));
#86009=CARTESIAN_POINT('Ctrl Pts',(0.260536690490967,-0.194662330764873,
-0.377879196228184));
#86010=CARTESIAN_POINT('Ctrl Pts',(0.305007425284199,0.112886047624917,
-0.362024875829198));
#86011=CARTESIAN_POINT('Ctrl Pts',(0.0710262974208254,0.317376834861157,
-0.346170555430214));
#86012=CARTESIAN_POINT('Ctrl Pts',(-0.227797209598448,0.232123291963083,
-0.330316235031228));
#86013=CARTESIAN_POINT('Ctrl Pts',(-0.318656723664062,-0.0650436606871058,
-0.314461914632243));
#86014=CARTESIAN_POINT('Ctrl Pts',(-0.11860347782392,-0.302829999773896,
-0.298607594233258));
#86015=CARTESIAN_POINT('Ctrl Pts',(0.189727046917343,-0.264152315967197,
-0.282753273834273));
#86016=CARTESIAN_POINT('Ctrl Pts',(0.324849074862728,0.0156791787866342,
-0.266898953435288));
#86017=CARTESIAN_POINT('Ctrl Pts',(0.163405277456162,0.281196621754686,
-0.251044633036303));
#86018=CARTESIAN_POINT('Ctrl Pts',(-0.147217197710538,0.289999879350344,
-0.235190312637318));
#86019=CARTESIAN_POINT('Ctrl Pts',(-0.323439356428613,0.0340522344471882,
-0.219335992238333));
#86020=CARTESIAN_POINT('Ctrl Pts',(-0.204383696274287,-0.252982980610236,
-0.203481671839348));
#86021=CARTESIAN_POINT('Ctrl Pts',(0.101263222726195,-0.30906105355394,
-0.187627351440363));
#86022=CARTESIAN_POINT('Ctrl Pts',(0.314459058179145,-0.0829869396098267,
-0.171773031041377));
#86023=CARTESIAN_POINT('Ctrl Pts',(0.240582660128564,0.218849553190984,
-0.155918710642392));
#86024=CARTESIAN_POINT('Ctrl Pts',(-0.0529459703154303,0.320889314101761,
-0.140064390243407));
#86025=CARTESIAN_POINT('Ctrl Pts',(-0.298107863124639,0.12998071460519,
-0.124210069844422));
#86026=CARTESIAN_POINT('Ctrl Pts',(-0.271175080951416,-0.179596823391934,
-0.108355749445437));
#86027=CARTESIAN_POINT('Ctrl Pts',(0.00343439755682056,-0.32520457577112,
-0.0925014290464522));
#86028=CARTESIAN_POINT('Ctrl Pts',(0.27469484658316,-0.173940096932386,
-0.0766471086474671));
#86029=CARTESIAN_POINT('Ctrl Pts',(0.295589188333754,0.136154857096479,
-0.0607927882484822));
#86030=CARTESIAN_POINT('Ctrl Pts',(0.0458060779164938,0.321887510694949,
-0.044938467849497));
#86031=CARTESIAN_POINT('Ctrl Pts',(-0.147344254484739,0.249864176030283,
-0.0343689209168401));
#86032=CARTESIAN_POINT('Ctrl Pts',(-0.207440123017129,0.180983245493314,
-0.0290841474505119));
#86033=CARTESIAN_POINT('Ctrl Pts',(0.148544839071951,-0.208524980625557,
-1.57169014387133));
#86034=CARTESIAN_POINT('Ctrl Pts',(0.21782220173782,-0.159178540378863,
-1.56640279516957));
#86035=CARTESIAN_POINT('Ctrl Pts',(0.3021119053827,0.0130859303836847,-1.55583067300148));
#86036=CARTESIAN_POINT('Ctrl Pts',(0.152896104723196,0.261201430501014,
-1.53997377736707));
#86037=CARTESIAN_POINT('Ctrl Pts',(-0.136011738435718,0.270059915908096,
-1.52411945696809));
#86038=CARTESIAN_POINT('Ctrl Pts',(-0.300680296067738,0.0327498435922312,
-1.5082651365691));
#86039=CARTESIAN_POINT('Ctrl Pts',(-0.190883752436815,-0.234654774653695,
-1.49241081617012));
#86040=CARTESIAN_POINT('Ctrl Pts',(0.0931962340611783,-0.287732531060864,
-1.47655649577114));
#86041=CARTESIAN_POINT('Ctrl Pts',(0.292184180852812,-0.0781828120964695,
-1.46070217537215));
#86042=CARTESIAN_POINT('Ctrl Pts',(0.224432259277494,0.202770721431455,
-1.44484785497317));
#86043=CARTESIAN_POINT('Ctrl Pts',(-0.0482143900054565,0.298593168295426,
-1.42899353457418));
#86044=CARTESIAN_POINT('Ctrl Pts',(-0.276843021835421,0.121827215569368,
-1.4131392141752));
#86045=CARTESIAN_POINT('Ctrl Pts',(-0.252732795808098,-0.166163043767173,
-1.39728489377621));
#86046=CARTESIAN_POINT('Ctrl Pts',(0.00210636327868856,-0.302455192953229,
-1.38143057337722));
#86047=CARTESIAN_POINT('Ctrl Pts',(0.255022345767755,-0.162626596005646,
-1.36557625297824));
#86048=CARTESIAN_POINT('Ctrl Pts',(0.27511968326167,0.125670040449278,-1.34972193257925));
#86049=CARTESIAN_POINT('Ctrl Pts',(0.0440506557848269,0.299237833871169,
-1.33386761218027));
#86050=CARTESIAN_POINT('Ctrl Pts',(-0.227233715188827,0.199621178765434,
-1.31801329178129));
#86051=CARTESIAN_POINT('Ctrl Pts',(-0.291068554992977,-0.0822366621682676,
-1.3021589713823));
#86052=CARTESIAN_POINT('Ctrl Pts',(-0.0891767991483039,-0.289017756467199,
-1.28630465098332));
#86053=CARTESIAN_POINT('Ctrl Pts',(0.194127548011667,-0.231944530841581,
-1.27045033058433));
#86054=CARTESIAN_POINT('Ctrl Pts',(0.300206120094121,0.0368789202075171,
-1.25459601018535));
#86055=CARTESIAN_POINT('Ctrl Pts',(0.132216103026753,0.272034318660143,
-1.23874168978636));
#86056=CARTESIAN_POINT('Ctrl Pts',(-0.15647858347169,0.258840147789478,
-1.22288736938738));
#86057=CARTESIAN_POINT('Ctrl Pts',(-0.302318539637954,0.00934181926968402,
-1.20703304898839));
#86058=CARTESIAN_POINT('Ctrl Pts',(-0.172161406509086,-0.248684979457122,
-1.19117872858941));
#86059=CARTESIAN_POINT('Ctrl Pts',(0.115167850724418,-0.279678628371122,
-1.17532440819042));
#86060=CARTESIAN_POINT('Ctrl Pts',(0.297356379288707,-0.0553439488005891,
-1.15947008779143));
#86061=CARTESIAN_POINT('Ctrl Pts',(0.208077947131682,0.21951614264167,-1.14361576739245));
#86062=CARTESIAN_POINT('Ctrl Pts',(-0.0711620658984849,0.293972327532916,
-1.12776144699346));
#86063=CARTESIAN_POINT('Ctrl Pts',(-0.285435758748384,0.100050970009206,
-1.11190712659448));
#86064=CARTESIAN_POINT('Ctrl Pts',(-0.23912523918544,-0.185210391057845,
-1.0960528061955));
#86065=CARTESIAN_POINT('Ctrl Pts',(0.0254910119126622,-0.301386756983511,
-1.08019848579651));
#86066=CARTESIAN_POINT('Ctrl Pts',(0.266835633374574,-0.142416690503555,
-1.06434416539752));
#86067=CARTESIAN_POINT('Ctrl Pts',(0.264576742541001,0.146570516403449,
-1.04848984499854));
#86068=CARTESIAN_POINT('Ctrl Pts',(0.0207765592668679,0.301748411027608,
-1.03263552459955));
#86069=CARTESIAN_POINT('Ctrl Pts',(-0.241991266172751,0.181449706719554,
-1.01678120420057));
#86070=CARTESIAN_POINT('Ctrl Pts',(-0.283836864551102,-0.104500733463044,
-1.00092688380158));
#86071=CARTESIAN_POINT('Ctrl Pts',(-0.0665579365346684,-0.295048826564006,
-0.985072563402594));
#86072=CARTESIAN_POINT('Ctrl Pts',(0.211484042150481,-0.216236603950906,
-0.969218243003609));
#86073=CARTESIAN_POINT('Ctrl Pts',(0.296454897572703,0.0599855205669558,
-0.953363922604623));
#86074=CARTESIAN_POINT('Ctrl Pts',(0.110781786248597,0.281444781099428,
-0.93750960220564));
#86075=CARTESIAN_POINT('Ctrl Pts',(-0.176027863277623,0.245963331255792,
-0.921655281806653));
#86076=CARTESIAN_POINT('Ctrl Pts',(-0.30213556601393,-0.014066581744478,
-0.905800961407669));
#86077=CARTESIAN_POINT('Ctrl Pts',(-0.152413222592527,-0.261254623981076,
-0.889946641008684));
#86078=CARTESIAN_POINT('Ctrl Pts',(0.136452442409244,-0.269934251129945,
-0.874092320609698));
#86079=CARTESIAN_POINT('Ctrl Pts',(0.300745936101864,-0.0321815302735241,
-0.858238000210714));
#86080=CARTESIAN_POINT('Ctrl Pts',(0.190478025021315,0.234950826677652,
-0.842383679811728));
#86081=CARTESIAN_POINT('Ctrl Pts',(-0.0936838871092037,0.287588418175423,
-0.826529359412743));
#86082=CARTESIAN_POINT('Ctrl Pts',(-0.292318526676337,0.0776765597481471,
-0.810675039013758));
#86083=CARTESIAN_POINT('Ctrl Pts',(-0.224085436073065,-0.203148926436928,
-0.794820718614773));
#86084=CARTESIAN_POINT('Ctrl Pts',(0.0487230277335556,-0.298512705828424,
-0.778966398215788));
#86085=CARTESIAN_POINT('Ctrl Pts',(0.277050548213993,-0.121353873884843,
-0.763112077816803));
#86086=CARTESIAN_POINT('Ctrl Pts',(0.252449006055172,0.166593122049766,
-0.747257757417818));
#86087=CARTESIAN_POINT('Ctrl Pts',(-0.00262199691997647,0.30245147396679,
-0.731403437018833));
#86088=CARTESIAN_POINT('Ctrl Pts',(-0.255299287890265,0.162191376389917,
-0.715549116619847));
#86089=CARTESIAN_POINT('Ctrl Pts',(-0.27490499681597,-0.126138858795157,
-0.699694796220863));
#86090=CARTESIAN_POINT('Ctrl Pts',(-0.0435403914515674,-0.299312551164792,
-0.683840475821877));
#86091=CARTESIAN_POINT('Ctrl Pts',(0.227573748673849,-0.199233425626985,
-0.667986155422893));
#86092=CARTESIAN_POINT('Ctrl Pts',(0.290927913933894,0.0827328100973711,
-0.652131835023907));
#86093=CARTESIAN_POINT('Ctrl Pts',(0.0886838876680271,0.289169391603979,
-0.636277514624922));
#86094=CARTESIAN_POINT('Ctrl Pts',(-0.194522738107825,0.231613197662744,
-0.620423194225936));
#86095=CARTESIAN_POINT('Ctrl Pts',(-0.300142803854146,-0.0373907243460496,
-0.604568873826953));
#86096=CARTESIAN_POINT('Ctrl Pts',(-0.131752085192487,-0.27225935616604,
-0.588714553427966));
#86097=CARTESIAN_POINT('Ctrl Pts',(0.15691968551282,-0.258572970882614,
-0.572860233028982));
#86098=CARTESIAN_POINT('Ctrl Pts',(0.302334028206672,-0.00882634471245425,
-0.557005912629997));
#86099=CARTESIAN_POINT('Ctrl Pts',(0.171737141717175,0.248978157931968,
-0.541151592231012));
#86100=CARTESIAN_POINT('Ctrl Pts',(-0.115644542905758,0.279481857494389,
-0.525297271832026));
#86101=CARTESIAN_POINT('Ctrl Pts',(-0.29745030997744,0.0548368677779214,
-0.509442951433041));
#86102=CARTESIAN_POINT('Ctrl Pts',(-0.207703363760013,-0.219870602068739,
-0.493588631034056));
#86103=CARTESIAN_POINT('Ctrl Pts',(0.0716631931704711,-0.293850566983732,
-0.477734310635071));
#86104=CARTESIAN_POINT('Ctrl Pts',(0.285605933450537,-0.0995641489488433,
-0.461879990236086));
#86105=CARTESIAN_POINT('Ctrl Pts',(0.238809102893179,0.185617836799614,
-0.446025669837101));
#86106=CARTESIAN_POINT('Ctrl Pts',(-0.0260048473387968,0.301342856041782,
-0.430171349438115));
#86107=CARTESIAN_POINT('Ctrl Pts',(-0.267078069864868,0.141961521565846,
-0.414317029039131));
#86108=CARTESIAN_POINT('Ctrl Pts',(-0.264326451163026,-0.147021413795191,
-0.398462708640145));
#86109=CARTESIAN_POINT('Ctrl Pts',(-0.0202620401764223,-0.301783397031682,
-0.382608388241161));
#86110=CARTESIAN_POINT('Ctrl Pts',(0.242300291533491,-0.181036841321789,
-0.366754067842175));
#86111=CARTESIAN_POINT('Ctrl Pts',(0.283658274490912,0.104984530961983,
-0.350899747443191));
#86112=CARTESIAN_POINT('Ctrl Pts',(0.0660547753914399,0.295161880915583,
-0.335045427044205));
#86113=CARTESIAN_POINT('Ctrl Pts',(-0.211852427357573,0.215875703373602,
-0.319191106645221));
#86114=CARTESIAN_POINT('Ctrl Pts',(-0.296352183246857,-0.0604908963769847,
-0.303336786246235));
#86115=CARTESIAN_POINT('Ctrl Pts',(-0.110301766708814,-0.281633258993308,
-0.28748246584725));
#86116=CARTESIAN_POINT('Ctrl Pts',(0.176447005192364,-0.245662839454535,
-0.271628145448265));
#86117=CARTESIAN_POINT('Ctrl Pts',(0.302111097654986,0.0145817066450353,
-0.25577382504928));
#86118=CARTESIAN_POINT('Ctrl Pts',(0.151967641452447,0.261514120337517,
-0.239919504650295));
#86119=CARTESIAN_POINT('Ctrl Pts',(-0.136912654631436,0.269701189413478,
-0.22406518425131));
#86120=CARTESIAN_POINT('Ctrl Pts',(-0.300800053183967,0.0316687308738422,
-0.208210863852325));
#86121=CARTESIAN_POINT('Ctrl Pts',(-0.190077754878324,-0.235275307440804,
-0.192356543453339));
#86122=CARTESIAN_POINT('Ctrl Pts',(0.0941752516389973,-0.287428166975827,
-0.176502223054355));
#86123=CARTESIAN_POINT('Ctrl Pts',(0.292448335505342,-0.0771782263106231,
-0.160647902655369));
#86124=CARTESIAN_POINT('Ctrl Pts',(0.223742953736009,0.203531066738519,
-0.144793582256384));
#86125=CARTESIAN_POINT('Ctrl Pts',(-0.0492399900327958,0.298428502374539,
-0.128939261857399));
#86126=CARTESIAN_POINT('Ctrl Pts',(-0.277241650714951,0.120882647980286,
-0.113084941458414));
#86127=CARTESIAN_POINT('Ctrl Pts',(-0.252194042410405,-0.167025851845859,
-0.0972306210594291));
#86128=CARTESIAN_POINT('Ctrl Pts',(0.00319400514258442,-0.3024417150954,
-0.081376300660444));
#86129=CARTESIAN_POINT('Ctrl Pts',(0.255467440245829,-0.161765070849173,
-0.0655219802614589));
#86130=CARTESIAN_POINT('Ctrl Pts',(0.274899271854761,0.126624628208832,
-0.0496676598624738));
#86131=CARTESIAN_POINT('Ctrl Pts',(0.0425998580555258,0.299356829686449,
-0.0338133394634889));
#86132=CARTESIAN_POINT('Ctrl Pts',(-0.137030818001717,0.232374805183194,
-0.023243792530832));
#86133=CARTESIAN_POINT('Ctrl Pts',(-0.192920245467447,0.168315230622872,
-0.0179590190645036));
#86134=CARTESIAN_POINT('Ctrl Pts',(0.137364815592633,-0.192830634097036,
-1.56056501548531));
#86135=CARTESIAN_POINT('Ctrl Pts',(0.201428112619947,-0.147198185962257,
-1.55527766678356));
#86136=CARTESIAN_POINT('Ctrl Pts',(0.27937386738244,0.0121010357898901,
-1.54470554461548));
#86137=CARTESIAN_POINT('Ctrl Pts',(0.141388589205448,0.241542463255316,
-1.52884864898106));
#86138=CARTESIAN_POINT('Ctrl Pts',(-0.125775001577849,0.249734226913857,
-1.51299432858207));
#86139=CARTESIAN_POINT('Ctrl Pts',(-0.278050006178113,0.0302849715536401,
-1.49714000818309));
#86140=CARTESIAN_POINT('Ctrl Pts',(-0.176517148740603,-0.216993805032989,
-1.48128568778411));
#86141=CARTESIAN_POINT('Ctrl Pts',(0.0861819473885653,-0.266076736937539,
-1.46543136738512));
#86142=CARTESIAN_POINT('Ctrl Pts',(0.270193339416458,-0.0722984900265885,
-1.44957704698614));
#86143=CARTESIAN_POINT('Ctrl Pts',(0.207540673249225,0.18750946132518,-1.43372272658715));
#86144=CARTESIAN_POINT('Ctrl Pts',(-0.0445856001015495,0.276119963213624,
-1.41786840618817));
#86145=CARTESIAN_POINT('Ctrl Pts',(-0.256006811681353,0.112658057361009,
-1.40201408578918));
#86146=CARTESIAN_POINT('Ctrl Pts',(-0.233711208731888,-0.153657010287193,
-1.3861597653902));
#86147=CARTESIAN_POINT('Ctrl Pts',(0.00194783073687467,-0.279691317885033,
-1.37030544499121));
#86148=CARTESIAN_POINT('Ctrl Pts',(0.235828438855558,-0.150386728413716,
-1.35445112459222));
#86149=CARTESIAN_POINT('Ctrl Pts',(0.254413177820586,0.116211657299466,
-1.33859680419324));
#86150=CARTESIAN_POINT('Ctrl Pts',(0.0407352436235497,0.276716108919421,
-1.32274248379426));
#86151=CARTESIAN_POINT('Ctrl Pts',(-0.210131281425556,0.184596964666106,
-1.30688816339527));
#86152=CARTESIAN_POINT('Ctrl Pts',(-0.269161679606099,-0.076047232635435,
-1.29103384299628));
#86153=CARTESIAN_POINT('Ctrl Pts',(-0.0824650297289307,-0.267265231617256,
-1.2751795225973));
#86154=CARTESIAN_POINT('Ctrl Pts',(0.179516804492658,-0.214487544002391,
-1.25932520219831));
#86155=CARTESIAN_POINT('Ctrl Pts',(0.277611518408485,0.0341032788834053,
-1.24347088179933));
#86156=CARTESIAN_POINT('Ctrl Pts',(0.122265039459559,0.251560028952052,
-1.22761656140035));
#86157=CARTESIAN_POINT('Ctrl Pts',(-0.144701437606821,0.239358899246907,
-1.21176224100136));
#86158=CARTESIAN_POINT('Ctrl Pts',(-0.279564949594017,0.00863872006120638,
-1.19590792060237));
#86159=CARTESIAN_POINT('Ctrl Pts',(-0.159203914488296,-0.229968045724152,
-1.18005360020339));
#86160=CARTESIAN_POINT('Ctrl Pts',(0.106499900473129,-0.258629000182165,
-1.1641992798044));
#86161=CARTESIAN_POINT('Ctrl Pts',(0.274976259434374,-0.0511785624371529,
-1.14834495940542));
#86162=CARTESIAN_POINT('Ctrl Pts',(0.192417245965658,0.202994561386096,
-1.13249063900643));
#86163=CARTESIAN_POINT('Ctrl Pts',(-0.0658061506573216,0.271846903690381,
-1.11663631860745));
#86164=CARTESIAN_POINT('Ctrl Pts',(-0.263952828041526,0.0925207710415389,
-1.10078199820846));
#86165=CARTESIAN_POINT('Ctrl Pts',(-0.221127806186127,-0.17127078512083,
-1.08492767780948));
#86166=CARTESIAN_POINT('Ctrl Pts',(0.0235724658798592,-0.278703296282466,
-1.06907335741049));
#86167=CARTESIAN_POINT('Ctrl Pts',(0.246752615580859,-0.13169789371718,
-1.05321903701151));
#86168=CARTESIAN_POINT('Ctrl Pts',(0.24466373706622,0.135539087610608,-1.03736471661252));
#86169=CARTESIAN_POINT('Ctrl Pts',(0.0192128400432681,0.279037730931197,
-1.02151039621354));
#86170=CARTESIAN_POINT('Ctrl Pts',(-0.223778125585007,0.167793143528841,
-1.00565607581455));
#86171=CARTESIAN_POINT('Ctrl Pts',(-0.262474272421997,-0.096635629154999,
-0.98980175541557));
#86172=CARTESIAN_POINT('Ctrl Pts',(-0.0615485447722762,-0.27284238149907,
-0.973947435016587));
#86173=CARTESIAN_POINT('Ctrl Pts',(0.195566985916719,-0.199961852674703,
-0.9580931146176));
#86174=CARTESIAN_POINT('Ctrl Pts',(0.274142626502709,0.0554707926736992,
-0.942238794218616));
#86175=CARTESIAN_POINT('Ctrl Pts',(0.102443947121514,0.260262225848894,
-0.926384473819631));
#86176=CARTESIAN_POINT('Ctrl Pts',(-0.162779367693708,0.227451238640043,
-0.910530153420645));
#86177=CARTESIAN_POINT('Ctrl Pts',(-0.279395747228729,-0.0130078797716646,
-0.894675833021661));
#86178=CARTESIAN_POINT('Ctrl Pts',(-0.14094205053573,-0.241591653201093,
-0.878821512622675));
#86179=CARTESIAN_POINT('Ctrl Pts',(0.126182536571542,-0.249618020122797,
-0.86296719222369));
#86180=CARTESIAN_POINT('Ctrl Pts',(0.278110705905143,-0.0297594315570249,
-0.847112871824706));
#86181=CARTESIAN_POINT('Ctrl Pts',(0.17614195784229,0.217267575107605,-0.83125855142572));
#86182=CARTESIAN_POINT('Ctrl Pts',(-0.0866328978990892,0.26594347051067,
-0.815404231026735));
#86183=CARTESIAN_POINT('Ctrl Pts',(-0.270317573885926,0.071830340066582,
-0.79954991062775));
#86184=CARTESIAN_POINT('Ctrl Pts',(-0.207219953217366,-0.187859201249889,
-0.783695590228765));
#86185=CARTESIAN_POINT('Ctrl Pts',(0.0450559559089969,-0.27604555664379,
-0.767841269829779));
#86186=CARTESIAN_POINT('Ctrl Pts',(0.256198718871808,-0.112220341088851,
-0.751986949430795));
#86187=CARTESIAN_POINT('Ctrl Pts',(0.233448778025299,0.154054719318002,
-0.736132629031809));
#86188=CARTESIAN_POINT('Ctrl Pts',(-0.00242465591970453,0.279687878803005,
-0.720278308632825));
#86189=CARTESIAN_POINT('Ctrl Pts',(-0.236084537309237,0.149984265005156,
-0.704423988233839));
#86190=CARTESIAN_POINT('Ctrl Pts',(-0.254214649455628,-0.116645190675855,
-0.688569667834855));
#86191=CARTESIAN_POINT('Ctrl Pts',(-0.0402633836351476,-0.276785202718466,
-0.672715347435869));
#86192=CARTESIAN_POINT('Ctrl Pts',(0.210445722756922,-0.184238395235546,
-0.656861027036884));
#86193=CARTESIAN_POINT('Ctrl Pts',(0.26903162370334,0.0765060386714696,
-0.641006706637899));
#86194=CARTESIAN_POINT('Ctrl Pts',(0.082009216554843,0.26740545414354,-0.625152386238914));
#86195=CARTESIAN_POINT('Ctrl Pts',(-0.179882251148508,0.214181148160604,
-0.609298065839929));
#86196=CARTESIAN_POINT('Ctrl Pts',(-0.277552967578429,-0.0345765627857494,
-0.593443745440943));
#86197=CARTESIAN_POINT('Ctrl Pts',(-0.121835945290864,-0.251768129318864,
-0.577589425041959));
#86198=CARTESIAN_POINT('Ctrl Pts',(0.145109340708106,-0.239111831043317,
-0.561735104642973));
#86199=CARTESIAN_POINT('Ctrl Pts',(0.279579272436864,-0.00816204198919175,
-0.545880784243989));
#86200=CARTESIAN_POINT('Ctrl Pts',(0.158811581403771,0.230239158523389,
-0.530026463845003));
#86201=CARTESIAN_POINT('Ctrl Pts',(-0.106940715071558,0.25844703899546,
-0.514172143446019));
#86202=CARTESIAN_POINT('Ctrl Pts',(-0.275063120558711,0.0507096461718393,
-0.498317823047033));
#86203=CARTESIAN_POINT('Ctrl Pts',(-0.192070855097454,-0.203322342910778,
-0.482463502648048));
#86204=CARTESIAN_POINT('Ctrl Pts',(0.0662695612728291,-0.27173430728185,
-0.466609182249063));
#86205=CARTESIAN_POINT('Ctrl Pts',(0.264110194778236,-0.092070589900268,
-0.450754861850078));
#86206=CARTESIAN_POINT('Ctrl Pts',(0.2208354634581,0.171647565017942,-0.434900541451093));
#86207=CARTESIAN_POINT('Ctrl Pts',(-0.0240476281877313,0.278662699484875,
-0.419046221052108));
#86208=CARTESIAN_POINT('Ctrl Pts',(-0.246976805421383,0.131276982444985,
-0.403191900653123));
#86209=CARTESIAN_POINT('Ctrl Pts',(-0.244432283525357,-0.135956048828884,
-0.387337580254138));
#86210=CARTESIAN_POINT('Ctrl Pts',(-0.0187370455261411,-0.279070083761682,
-0.371483259855153));
#86211=CARTESIAN_POINT('Ctrl Pts',(0.224063892576015,-0.167411351878704,
-0.355628939456167));
#86212=CARTESIAN_POINT('Ctrl Pts',(0.262309123697625,0.0970830142990478,
-0.339774619057182));
#86213=CARTESIAN_POINT('Ctrl Pts',(0.0610832533620543,0.272946926970009,
-0.323920298658198));
#86214=CARTESIAN_POINT('Ctrl Pts',(-0.195907645116697,0.199628114784122,
-0.308065978259212));
#86215=CARTESIAN_POINT('Ctrl Pts',(-0.274047642829653,-0.0559381320668637,
-0.292211657860227));
#86216=CARTESIAN_POINT('Ctrl Pts',(-0.102000055593709,-0.260436518212721,
-0.276357337461242));
#86217=CARTESIAN_POINT('Ctrl Pts',(0.163166963467383,-0.227173362941872,
-0.260503017062257));
#86218=CARTESIAN_POINT('Ctrl Pts',(0.279373120447245,0.0134842345034367,
-0.244648696663271));
#86219=CARTESIAN_POINT('Ctrl Pts',(0.140530005448733,0.241831618920349,
-0.228794376264287));
#86220=CARTESIAN_POINT('Ctrl Pts',(-0.126608111552335,0.249402499476613,
-0.212940055865302));
#86221=CARTESIAN_POINT('Ctrl Pts',(-0.278160749939319,0.0292852273004961,
-0.197085735466316));
#86222=CARTESIAN_POINT('Ctrl Pts',(-0.17577181348236,-0.217567634271371,
-0.181231415067331));
#86223=CARTESIAN_POINT('Ctrl Pts',(0.0870872805517992,-0.265795280397715,
-0.165377094668346));
#86224=CARTESIAN_POINT('Ctrl Pts',(0.270437612831538,-0.0713695130114197,
-0.149522774269361));
#86225=CARTESIAN_POINT('Ctrl Pts',(0.206903247343454,0.188212580286055,
-0.133668453870376));
#86226=CARTESIAN_POINT('Ctrl Pts',(-0.0455340097501608,0.275967690647318,
-0.117814133471391));
#86227=CARTESIAN_POINT('Ctrl Pts',(-0.256375438305264,0.111784581355383,
-0.101959813072406));
#86228=CARTESIAN_POINT('Ctrl Pts',(-0.233213003869395,-0.154454880299785,
-0.0861054926734209));
#86229=CARTESIAN_POINT('Ctrl Pts',(0.00295361272834789,-0.279678854419679,
-0.0702511722744358));
#86230=CARTESIAN_POINT('Ctrl Pts',(0.236240033908498,-0.14959004476596,
-0.0543968518754509));
#86231=CARTESIAN_POINT('Ctrl Pts',(0.254209355375769,0.117094399321184,
-0.0385425314764656));
#86232=CARTESIAN_POINT('Ctrl Pts',(0.0393936381945584,0.27682614867795,
-0.0226882110774808));
#86233=CARTESIAN_POINT('Ctrl Pts',(-0.126717381518695,0.214885434336106,
-0.0121186641448238));
#86234=CARTESIAN_POINT('Ctrl Pts',(-0.178400367917765,0.155647215752429,
-0.00683389067849545));
#86235=CARTESIAN_POINT('Ctrl Pts',(0.133736061201431,0.262046381265468,
-1.5608));
#86236=CARTESIAN_POINT('Ctrl Pts',(0.132207210795712,0.262985442201215,
-1.5608));
#86237=CARTESIAN_POINT('Ctrl Pts',(0.130678360389994,0.263924503136962,
-1.5608));
#86238=CARTESIAN_POINT('Ctrl Pts',(0.129149509984275,0.264863564072709,
-1.5608));
#86239=CARTESIAN_POINT('Origin',(0.,0.,-0.04));
#86240=CARTESIAN_POINT('',(-0.3342,4.09276960275046E-17,0.));
#86241=CARTESIAN_POINT('Origin',(0.,0.,0.));
#86242=CARTESIAN_POINT('Origin',(-0.3342,-4.09276960275045E-17,-0.04));
#86243=CARTESIAN_POINT('Origin',(0.48,0.,0.));
#86244=CARTESIAN_POINT('',(-0.48,-5.8783046359073E-17,3.46944695195361E-18));
#86245=CARTESIAN_POINT('Origin',(0.,0.,0.));
#86246=CARTESIAN_POINT('Origin',(0.,0.,0.6066185719505));
#86247=CARTESIAN_POINT('',(-0.25,0.144337567297406,0.588452994616207));
#86248=CARTESIAN_POINT('',(-0.25,-5.3231743852413E-17,0.566123895246948));
#86249=CARTESIAN_POINT('Ctrl Pts',(-0.25,0.144337567297406,0.588452994616208));
#86250=CARTESIAN_POINT('Ctrl Pts',(-0.25,0.0669872981077805,0.566123895246948));
#86251=CARTESIAN_POINT('Ctrl Pts',(-0.25,-7.58473177261421E-17,0.566123895246948));
#86252=CARTESIAN_POINT('',(1.76762539787485E-17,0.288675134594813,0.588452994616207));
#86253=CARTESIAN_POINT('Ctrl Pts',(1.76762539787485E-17,0.288675134594813,
0.588452994616207));
#86254=CARTESIAN_POINT('Ctrl Pts',(-0.125,0.21650635094611,0.546786327949541));
#86255=CARTESIAN_POINT('Ctrl Pts',(-0.25,0.144337567297406,0.588452994616207));
#86256=CARTESIAN_POINT('',(0.25,0.144337567297406,0.588452994616207));
#86257=CARTESIAN_POINT('Ctrl Pts',(0.25,0.144337567297406,0.588452994616207));
#86258=CARTESIAN_POINT('Ctrl Pts',(0.125,0.21650635094611,0.546786327949541));
#86259=CARTESIAN_POINT('Ctrl Pts',(1.76762539787485E-17,0.288675134594813,
0.588452994616207));
#86260=CARTESIAN_POINT('',(0.25,-0.144337567297407,0.588452994616207));
#86261=CARTESIAN_POINT('Ctrl Pts',(0.25,-0.144337567297407,0.588452994616207));
#86262=CARTESIAN_POINT('Ctrl Pts',(0.25,-2.77555756156289E-17,0.546786327949541));
#86263=CARTESIAN_POINT('Ctrl Pts',(0.25,0.144337567297406,0.588452994616207));
#86264=CARTESIAN_POINT('',(-5.30287619362454E-17,-0.288675134594813,0.588452994616207));
#86265=CARTESIAN_POINT('Ctrl Pts',(-5.30287619362454E-17,-0.288675134594813,
0.588452994616207));
#86266=CARTESIAN_POINT('Ctrl Pts',(0.125,-0.21650635094611,0.546786327949541));
#86267=CARTESIAN_POINT('Ctrl Pts',(0.25,-0.144337567297407,0.588452994616207));
#86268=CARTESIAN_POINT('',(-0.25,-0.144337567297406,0.588452994616207));
#86269=CARTESIAN_POINT('Ctrl Pts',(-0.25,-0.144337567297406,0.588452994616207));
#86270=CARTESIAN_POINT('Ctrl Pts',(-0.125,-0.21650635094611,0.546786327949541));
#86271=CARTESIAN_POINT('Ctrl Pts',(-5.30287619362454E-17,-0.288675134594813,
0.588452994616207));
#86272=CARTESIAN_POINT('Ctrl Pts',(-0.25,-7.58473177261421E-17,0.566123895246948));
#86273=CARTESIAN_POINT('Ctrl Pts',(-0.25,-0.0669872981077807,0.566123895246948));
#86274=CARTESIAN_POINT('Ctrl Pts',(-0.25,-0.144337567297406,0.588452994616208));
#86275=CARTESIAN_POINT('',(-0.308675134594813,3.78018015557916E-17,0.6));
#86276=CARTESIAN_POINT('',(-0.320138837486628,-3.92057002610754E-17,0.6066185719505));
#86277=CARTESIAN_POINT('Origin',(0.,0.,0.6));
#86278=CARTESIAN_POINT('Origin',(-5.55111512312578E-17,-0.288675134594813,
0.6));
#86279=CARTESIAN_POINT('',(-5.55111512312578E-17,-0.288675134594813,0.25));
#86280=CARTESIAN_POINT('',(-5.30287619362453E-17,-0.288675134594813,0.6));
#86281=CARTESIAN_POINT('',(-0.25,-0.144337567297406,0.25));
#86282=CARTESIAN_POINT('',(-0.25,-0.144337567297406,0.25));
#86283=CARTESIAN_POINT('',(-0.25,-0.144337567297406,0.6));
#86284=CARTESIAN_POINT('Origin',(0.25,-0.144337567297407,0.6));
#86285=CARTESIAN_POINT('',(0.25,-0.144337567297407,0.25));
#86286=CARTESIAN_POINT('',(0.25,-0.144337567297407,0.6));
#86287=CARTESIAN_POINT('',(-5.30287619362453E-17,-0.288675134594813,0.25));
#86288=CARTESIAN_POINT('Origin',(0.25,0.144337567297406,0.6));
#86289=CARTESIAN_POINT('',(0.25,0.144337567297406,0.25));
#86290=CARTESIAN_POINT('',(0.25,0.144337567297406,0.6));
#86291=CARTESIAN_POINT('',(0.25,-0.144337567297407,0.25));
#86292=CARTESIAN_POINT('Origin',(0.,0.,0.176894574169124));
#86293=CARTESIAN_POINT('',(0.,0.,0.102789148338248));
#86294=CARTESIAN_POINT('',(-0.243346949651439,2.98014062972907E-17,0.25));
#86295=CARTESIAN_POINT('',(-0.1225,-1.50019232895551E-17,0.176894574169124));
#86296=CARTESIAN_POINT('Origin',(0.,0.,0.25));
#86297=CARTESIAN_POINT('Origin',(0.,0.288675134594813,0.6));
#86298=CARTESIAN_POINT('',(2.77555756156289E-17,0.288675134594813,0.25));
#86299=CARTESIAN_POINT('',(1.76762539787485E-17,0.288675134594813,0.6));
#86300=CARTESIAN_POINT('',(0.25,0.144337567297406,0.25));
#86301=CARTESIAN_POINT('Origin',(-0.25,0.144337567297406,0.6));
#86302=CARTESIAN_POINT('',(-0.25,0.144337567297406,0.25));
#86303=CARTESIAN_POINT('',(-0.25,0.144337567297406,0.6));
#86304=CARTESIAN_POINT('',(1.76762539787485E-17,0.288675134594813,0.25));
#86305=CARTESIAN_POINT('Origin',(-0.25,-0.144337567297406,0.6));
#86306=CARTESIAN_POINT('',(-0.25,0.144337567297406,0.25));
#86307=CARTESIAN_POINT('Origin',(0.,0.,0.25));
#86308=CARTESIAN_POINT('Origin',(0.,0.,0.54));
#86309=CARTESIAN_POINT('',(-0.44,-5.38844591624835E-17,0.6));
#86310=CARTESIAN_POINT('Origin',(0.,0.,0.6));
#86311=CARTESIAN_POINT('',(-0.5,-6.12323399573677E-17,0.54));
#86312=CARTESIAN_POINT('Origin',(-0.44,-5.38844591624835E-17,0.54));
#86313=CARTESIAN_POINT('Origin',(0.,0.,0.54));
#86314=CARTESIAN_POINT('Origin',(0.,0.,0.31));
#86315=CARTESIAN_POINT('',(-0.5,-6.12323399573677E-17,0.02));
#86316=CARTESIAN_POINT('',(-0.5,-6.12323399573677E-17,0.31));
#86317=CARTESIAN_POINT('Origin',(0.,0.,0.02));
#86318=CARTESIAN_POINT('Origin',(0.,0.,0.6));
#86319=CARTESIAN_POINT('Origin',(0.255,0.,-1.6));
#86320=CARTESIAN_POINT('',(-0.255,-3.12284933782575E-17,-1.6));
#86321=CARTESIAN_POINT('Origin',(0.,0.,-1.6));
#86322=CARTESIAN_POINT('Origin',(0.,0.,-1.5775));
#86323=CARTESIAN_POINT('',(-0.2775,-3.39839486763391E-17,-1.5775));
#86324=CARTESIAN_POINT('Origin',(0.,0.,0.01));
#86325=CARTESIAN_POINT('',(-0.49,-6.00076931582203E-17,0.01));
#86407=UNCERTAINTY_MEASURE_WITH_UNIT(LENGTH_MEASURE(0.001),#86430,
'DISTANCE_ACCURACY_VALUE',
'Maximum model space distance between geometric entities at asserted c
onnectivities');
#86409=UNCERTAINTY_MEASURE_WITH_UNIT(LENGTH_MEASURE(0.001),#86430,
'DISTANCE_ACCURACY_VALUE',
'Maximum model space distance between geometric entities at asserted c
onnectivities');
#86427=(
GEOMETRIC_REPRESENTATION_CONTEXT(3)
GLOBAL_UNCERTAINTY_ASSIGNED_CONTEXT((#86407))
GLOBAL_UNIT_ASSIGNED_CONTEXT((#86430,#86432,#86433))
REPRESENTATION_CONTEXT('','3D')
);
#86429=(
GEOMETRIC_REPRESENTATION_CONTEXT(3)
GLOBAL_UNCERTAINTY_ASSIGNED_CONTEXT((#86409))
GLOBAL_UNIT_ASSIGNED_CONTEXT((#86430,#86432,#86433))
REPRESENTATION_CONTEXT('','3D')
);
#86430=(
LENGTH_UNIT()
NAMED_UNIT(*)
SI_UNIT(.CENTI.,.METRE.)
);
#86432=(
NAMED_UNIT(*)
PLANE_ANGLE_UNIT()
SI_UNIT($,.RADIAN.)
);
#86433=(
NAMED_UNIT(*)
SI_UNIT($,.STERADIAN.)
SOLID_ANGLE_UNIT()
);
#86451=SHAPE_DEFINITION_REPRESENTATION(#86470,#86518);
#86470=PRODUCT_DEFINITION_SHAPE('',$,#86538);
#86518=SHAPE_REPRESENTATION('',(#17181),#86427);
#86520=PRODUCT_DEFINITION_CONTEXT('part definition',#86579,'design');
#86538=PRODUCT_DEFINITION('ISO 4762 M6x16 A2 SHCS',
'ISO 4762 M6x16 A2 SHCS',#86557,#86520);
#86557=PRODUCT_DEFINITION_FORMATION('',$,#86598);
#86579=APPLICATION_CONTEXT(
'Core Data for Automotive Mechanical Design Process');
#86580=PRODUCT_CONTEXT('part definition',#86579,'mechanical');
#86598=PRODUCT('ISO 4762 M6x16 A2 SHCS','ISO 4762 M6x16 A2 SHCS',$,(#86580));
#86617=PRESENTATION_STYLE_ASSIGNMENT((#86635));
#86635=SURFACE_STYLE_USAGE(.BOTH.,#86653);
#86653=SURFACE_SIDE_STYLE('',(#86671));
#86671=SURFACE_STYLE_FILL_AREA(#86689);
#86689=FILL_AREA_STYLE('Opaque(203,207,212)',(#86707));
#86707=FILL_AREA_STYLE_COLOUR('Opaque(203,207,212)',#86725);
#86725=COLOUR_RGB('Opaque(203,207,212)', 0.72549020, 0.75294118, 0.79215686);
ENDSEC;
END-ISO-10303-21;
